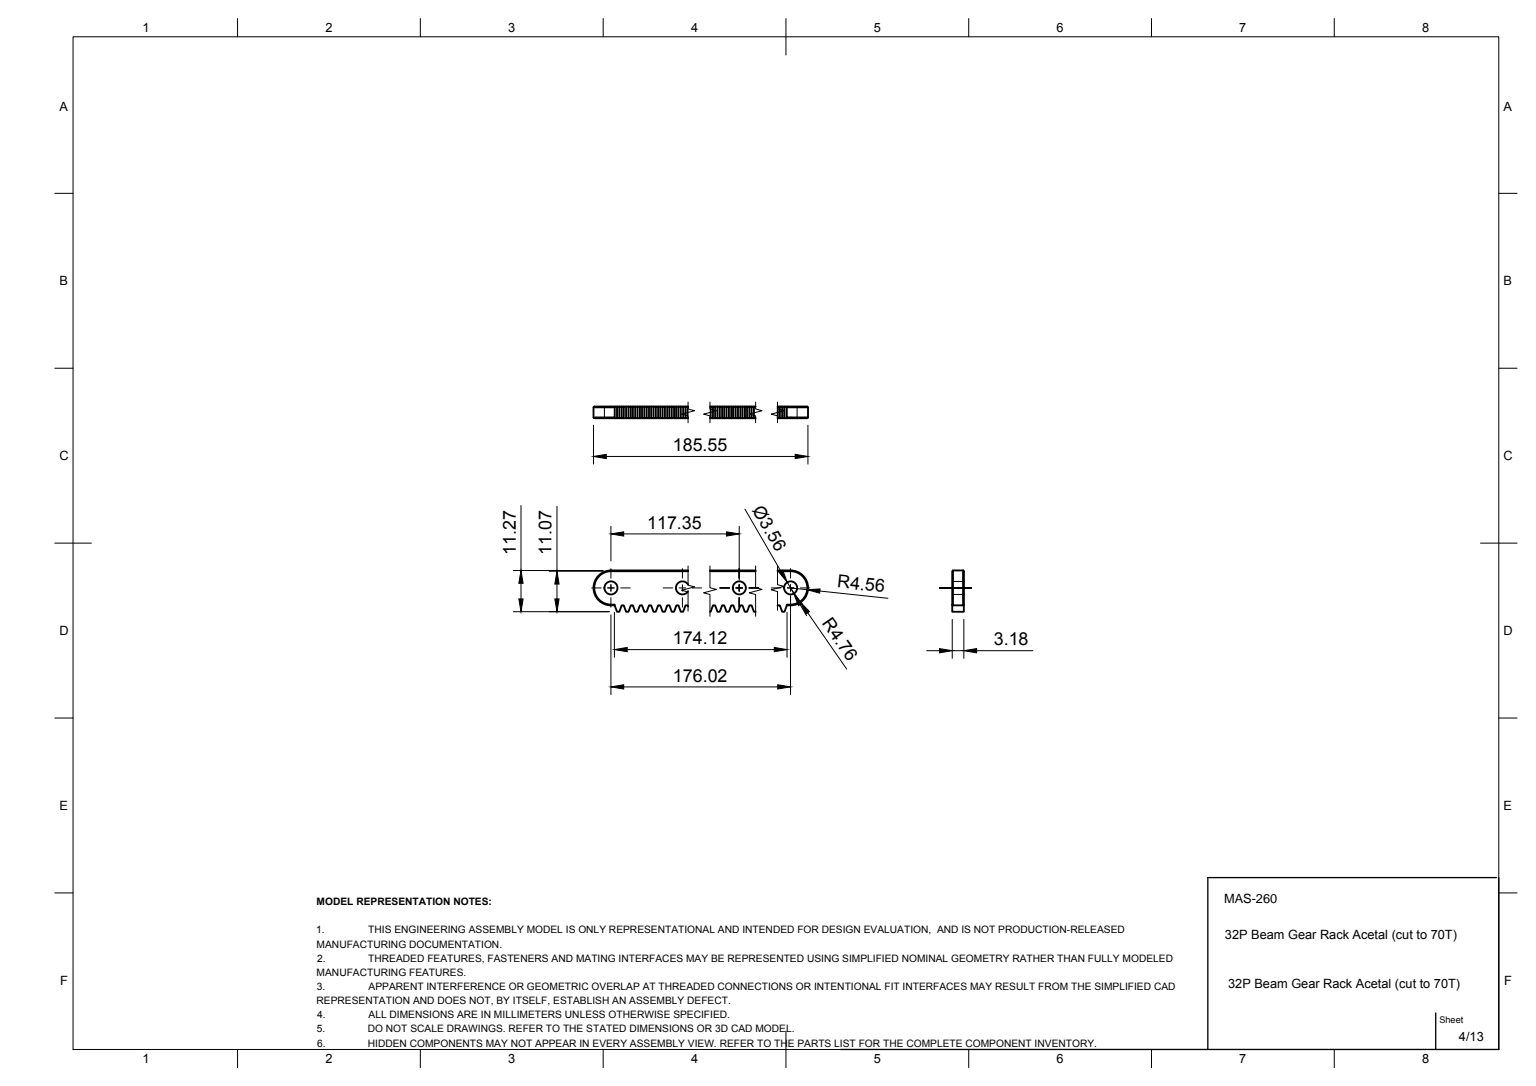
ISO-10303-21;
HEADER;
/* Generated by software containing ST-Developer
 * from STEP Tools, Inc. (www.steptools.com) 
 */

FILE_DESCRIPTION(
/* description */ (''),
/* implementation_level */ '2;1');

FILE_NAME(
/* name */ '32P Beam Gear Rack Acetal (cut to 70T).step',
/* time_stamp */ '2026-10-15T13:29:10-07:00',
/* author */ (''),
/* organization */ (''),
/* preprocessor_version */ 'ST-DEVELOPER v20.2',
/* originating_system */ 'Autodesk Translation Framework v15.15.0.0',
/* authorisation */ '');

FILE_SCHEMA (('AUTOMOTIVE_DESIGN { 1 0 10303 214 3 1 1 }'));
ENDSEC;

DATA;
#10=MECHANICAL_DESIGN_GEOMETRIC_PRESENTATION_REPRESENTATION('',(#939),#83219);
#911=SHAPE_REPRESENTATION_RELATIONSHIP('SRR','None',#83306,#925);
#925=ADVANCED_BREP_SHAPE_REPRESENTATION('',(#953),#83211);
#939=STYLED_ITEM('',(#83385),#953);
#953=MANIFOLD_SOLID_BREP('Body1',#26935);
#1061=FACE_BOUND('',#4681,.T.);
#1062=FACE_BOUND('',#4682,.T.);
#1063=FACE_BOUND('',#4683,.T.);
#1064=FACE_BOUND('',#4684,.T.);
#1065=FACE_BOUND('',#4685,.T.);
#1066=FACE_BOUND('',#4686,.T.);
#1067=FACE_BOUND('',#4687,.T.);
#1068=FACE_BOUND('',#4688,.T.);
#1069=FACE_BOUND('',#4689,.T.);
#1070=FACE_BOUND('',#4690,.T.);
#1071=FACE_BOUND('',#4692,.T.);
#1072=FACE_BOUND('',#4693,.T.);
#1073=FACE_BOUND('',#4694,.T.);
#1074=FACE_BOUND('',#4695,.T.);
#1075=FACE_BOUND('',#4696,.T.);
#1076=FACE_BOUND('',#4697,.T.);
#1077=FACE_BOUND('',#4698,.T.);
#1078=FACE_BOUND('',#4699,.T.);
#1079=FACE_BOUND('',#4700,.T.);
#1080=FACE_BOUND('',#4701,.T.);
#1423=PLANE('',#28001);
#1424=PLANE('',#28005);
#1425=PLANE('',#28009);
#1426=PLANE('',#28010);
#1427=PLANE('',#28013);
#1428=PLANE('',#28016);
#1429=PLANE('',#28017);
#1430=PLANE('',#28020);
#1431=PLANE('',#28023);
#1432=PLANE('',#28054);
#1433=PLANE('',#28055);
#1434=PLANE('',#28056);
#1435=PLANE('',#28057);
#1436=PLANE('',#28058);
#1437=PLANE('',#28059);
#1438=PLANE('',#28060);
#1439=PLANE('',#28061);
#1440=PLANE('',#28062);
#1441=PLANE('',#28063);
#1442=PLANE('',#28064);
#1443=PLANE('',#28065);
#1444=PLANE('',#28066);
#1445=PLANE('',#28067);
#1446=PLANE('',#28068);
#1447=PLANE('',#28069);
#1448=PLANE('',#28070);
#1449=PLANE('',#28071);
#1450=PLANE('',#28072);
#1451=PLANE('',#28073);
#1452=PLANE('',#28074);
#1453=PLANE('',#28075);
#1454=PLANE('',#28076);
#1455=PLANE('',#28077);
#1456=PLANE('',#28078);
#1457=PLANE('',#28079);
#1458=PLANE('',#28080);
#1459=PLANE('',#28081);
#1460=PLANE('',#28082);
#1461=PLANE('',#28083);
#1462=PLANE('',#28084);
#1463=PLANE('',#28085);
#1464=PLANE('',#28086);
#1465=PLANE('',#28087);
#1466=PLANE('',#28088);
#1467=PLANE('',#28089);
#1468=PLANE('',#28090);
#1469=PLANE('',#28091);
#1470=PLANE('',#28092);
#1471=PLANE('',#28093);
#1472=PLANE('',#28094);
#1473=PLANE('',#28095);
#1474=PLANE('',#28096);
#1475=PLANE('',#28097);
#1476=PLANE('',#28098);
#1477=PLANE('',#28099);
#1478=PLANE('',#28100);
#1479=PLANE('',#28101);
#1480=PLANE('',#28102);
#1481=PLANE('',#28103);
#1482=PLANE('',#28104);
#1483=PLANE('',#28105);
#1484=PLANE('',#28106);
#1485=PLANE('',#28107);
#1486=PLANE('',#28108);
#1487=PLANE('',#28109);
#1488=PLANE('',#28110);
#1489=PLANE('',#28111);
#1490=PLANE('',#28112);
#1491=PLANE('',#28113);
#1492=PLANE('',#28114);
#1493=PLANE('',#28115);
#1494=PLANE('',#28116);
#1495=PLANE('',#28117);
#1496=PLANE('',#28118);
#1497=PLANE('',#28119);
#1498=PLANE('',#28120);
#1499=PLANE('',#28121);
#1500=PLANE('',#28122);
#1501=PLANE('',#28123);
#1502=PLANE('',#28124);
#1503=PLANE('',#28125);
#1504=PLANE('',#28126);
#1505=PLANE('',#28127);
#1506=PLANE('',#28128);
#1507=PLANE('',#28129);
#1508=PLANE('',#28130);
#1509=PLANE('',#28131);
#1510=PLANE('',#28132);
#1511=PLANE('',#28133);
#1512=PLANE('',#28134);
#1513=PLANE('',#28135);
#1514=PLANE('',#28136);
#1515=PLANE('',#28137);
#1516=PLANE('',#28138);
#1517=PLANE('',#28139);
#1518=PLANE('',#28140);
#1519=PLANE('',#28141);
#1520=PLANE('',#28142);
#1521=PLANE('',#28143);
#1522=PLANE('',#28144);
#1523=PLANE('',#28145);
#1524=PLANE('',#28146);
#1525=PLANE('',#28147);
#1526=PLANE('',#28148);
#1527=PLANE('',#28149);
#1528=PLANE('',#28150);
#1529=PLANE('',#28151);
#1530=PLANE('',#28152);
#1531=PLANE('',#28153);
#1532=PLANE('',#28154);
#1533=PLANE('',#28155);
#1534=PLANE('',#28156);
#1535=PLANE('',#28157);
#1536=PLANE('',#28158);
#1537=PLANE('',#28159);
#1538=PLANE('',#28160);
#1539=PLANE('',#28161);
#1540=PLANE('',#28162);
#1541=PLANE('',#28163);
#1542=PLANE('',#28164);
#1543=PLANE('',#28165);
#1544=PLANE('',#28166);
#1545=PLANE('',#28167);
#1546=PLANE('',#28168);
#1547=PLANE('',#28169);
#1548=PLANE('',#28170);
#1549=PLANE('',#28171);
#1550=PLANE('',#28172);
#1551=PLANE('',#28173);
#1552=PLANE('',#28174);
#1553=PLANE('',#28175);
#1554=PLANE('',#28176);
#1555=PLANE('',#28177);
#1556=PLANE('',#28178);
#1557=PLANE('',#28179);
#1558=PLANE('',#28180);
#1559=PLANE('',#28181);
#1560=PLANE('',#28182);
#1561=PLANE('',#28183);
#1562=PLANE('',#28184);
#1563=PLANE('',#28185);
#1564=PLANE('',#28186);
#1565=PLANE('',#28187);
#1566=PLANE('',#28188);
#1567=PLANE('',#28189);
#1568=PLANE('',#28190);
#1569=PLANE('',#28191);
#1570=PLANE('',#28192);
#1571=PLANE('',#28193);
#1572=PLANE('',#28194);
#1573=PLANE('',#28195);
#1574=PLANE('',#28196);
#1575=PLANE('',#28197);
#1576=PLANE('',#28198);
#1577=PLANE('',#28199);
#1578=PLANE('',#28200);
#1579=PLANE('',#28201);
#1580=PLANE('',#28202);
#1581=PLANE('',#28203);
#1582=PLANE('',#28204);
#1583=PLANE('',#28205);
#1584=PLANE('',#28206);
#1585=PLANE('',#28207);
#1586=PLANE('',#28208);
#1587=PLANE('',#28209);
#1588=PLANE('',#28210);
#1589=PLANE('',#28211);
#1590=PLANE('',#28212);
#1591=PLANE('',#28213);
#1592=PLANE('',#28214);
#1593=PLANE('',#28215);
#1594=PLANE('',#28216);
#1595=PLANE('',#28217);
#1596=PLANE('',#28218);
#1597=PLANE('',#28219);
#1598=PLANE('',#28220);
#1599=PLANE('',#28221);
#1600=PLANE('',#28222);
#1601=PLANE('',#28223);
#1602=PLANE('',#28224);
#1603=PLANE('',#28225);
#1604=PLANE('',#28226);
#1605=PLANE('',#28227);
#1606=PLANE('',#28228);
#1607=PLANE('',#28229);
#1608=PLANE('',#28230);
#1609=PLANE('',#28231);
#1610=PLANE('',#28232);
#1611=PLANE('',#28233);
#1612=PLANE('',#28234);
#1613=PLANE('',#28235);
#1614=PLANE('',#28236);
#1615=PLANE('',#28237);
#1616=PLANE('',#28238);
#1617=PLANE('',#28239);
#1618=PLANE('',#28240);
#1619=PLANE('',#28241);
#1620=PLANE('',#28242);
#1621=PLANE('',#28243);
#1622=PLANE('',#28244);
#1623=PLANE('',#28245);
#1624=PLANE('',#28246);
#1625=PLANE('',#28247);
#1626=PLANE('',#28248);
#1627=PLANE('',#28249);
#1628=PLANE('',#28250);
#1629=PLANE('',#28251);
#1630=PLANE('',#28252);
#1631=PLANE('',#28253);
#1632=PLANE('',#28254);
#1633=PLANE('',#28255);
#1634=PLANE('',#28256);
#1635=PLANE('',#28257);
#1636=PLANE('',#28258);
#1637=PLANE('',#28259);
#1638=PLANE('',#28260);
#1639=PLANE('',#28261);
#1640=PLANE('',#28262);
#1641=PLANE('',#28263);
#1642=PLANE('',#28264);
#1643=PLANE('',#28265);
#1644=PLANE('',#28266);
#1645=PLANE('',#28267);
#1646=PLANE('',#28268);
#1647=PLANE('',#28269);
#1648=PLANE('',#28270);
#1649=PLANE('',#28271);
#1650=PLANE('',#28272);
#1651=PLANE('',#28273);
#1652=PLANE('',#28274);
#1653=PLANE('',#28275);
#1654=PLANE('',#28276);
#1655=PLANE('',#28277);
#1656=PLANE('',#28278);
#1657=PLANE('',#28279);
#1658=PLANE('',#28280);
#1659=PLANE('',#28281);
#1660=PLANE('',#28282);
#1661=PLANE('',#28283);
#1662=PLANE('',#28284);
#1663=PLANE('',#28285);
#1664=PLANE('',#28286);
#1665=PLANE('',#28287);
#1666=PLANE('',#28288);
#1667=PLANE('',#28289);
#1668=PLANE('',#28290);
#1669=PLANE('',#28291);
#1670=PLANE('',#28292);
#1671=PLANE('',#28293);
#1672=PLANE('',#28294);
#1673=PLANE('',#28295);
#1674=PLANE('',#28296);
#1675=PLANE('',#28297);
#1676=PLANE('',#28298);
#1677=PLANE('',#28299);
#1678=PLANE('',#28300);
#1679=PLANE('',#28301);
#1680=PLANE('',#28302);
#1681=PLANE('',#28303);
#1682=PLANE('',#28304);
#1683=PLANE('',#28305);
#1684=PLANE('',#28306);
#1685=PLANE('',#28307);
#1686=PLANE('',#28308);
#1687=PLANE('',#28309);
#1688=PLANE('',#28310);
#1689=PLANE('',#28311);
#1690=PLANE('',#28312);
#1691=PLANE('',#28313);
#1692=PLANE('',#28314);
#1693=PLANE('',#28315);
#1694=PLANE('',#28316);
#1695=PLANE('',#28317);
#1696=PLANE('',#28318);
#1697=PLANE('',#28319);
#1698=PLANE('',#28320);
#1699=PLANE('',#28321);
#1700=PLANE('',#28322);
#1701=PLANE('',#28323);
#1702=PLANE('',#28324);
#1703=PLANE('',#28325);
#1704=PLANE('',#28326);
#1705=PLANE('',#28327);
#1706=PLANE('',#28328);
#1707=PLANE('',#28329);
#1708=PLANE('',#28330);
#1709=PLANE('',#28331);
#1710=PLANE('',#28332);
#1711=PLANE('',#28333);
#1712=PLANE('',#28334);
#2282=CYLINDRICAL_SURFACE('',#28011,4.7625);
#2283=CYLINDRICAL_SURFACE('',#28014,4.7625);
#2284=CYLINDRICAL_SURFACE('',#28024,1.778);
#2285=CYLINDRICAL_SURFACE('',#28027,1.778);
#2286=CYLINDRICAL_SURFACE('',#28030,1.778);
#2287=CYLINDRICAL_SURFACE('',#28033,1.778);
#2288=CYLINDRICAL_SURFACE('',#28036,1.778);
#2289=CYLINDRICAL_SURFACE('',#28039,1.778);
#2290=CYLINDRICAL_SURFACE('',#28042,1.778);
#2291=CYLINDRICAL_SURFACE('',#28045,1.778);
#2292=CYLINDRICAL_SURFACE('',#28048,1.778);
#2293=CYLINDRICAL_SURFACE('',#28051,1.778);
#2897=FACE_OUTER_BOUND('',#4376,.T.);
#2898=FACE_OUTER_BOUND('',#4377,.T.);
#2899=FACE_OUTER_BOUND('',#4378,.T.);
#2900=FACE_OUTER_BOUND('',#4379,.T.);
#2901=FACE_OUTER_BOUND('',#4380,.T.);
#2902=FACE_OUTER_BOUND('',#4381,.T.);
#2903=FACE_OUTER_BOUND('',#4382,.T.);
#2904=FACE_OUTER_BOUND('',#4383,.T.);
#2905=FACE_OUTER_BOUND('',#4384,.T.);
#2906=FACE_OUTER_BOUND('',#4385,.T.);
#2907=FACE_OUTER_BOUND('',#4386,.T.);
#2908=FACE_OUTER_BOUND('',#4387,.T.);
#2909=FACE_OUTER_BOUND('',#4388,.T.);
#2910=FACE_OUTER_BOUND('',#4389,.T.);
#2911=FACE_OUTER_BOUND('',#4390,.T.);
#2912=FACE_OUTER_BOUND('',#4391,.T.);
#2913=FACE_OUTER_BOUND('',#4392,.T.);
#2914=FACE_OUTER_BOUND('',#4393,.T.);
#2915=FACE_OUTER_BOUND('',#4394,.T.);
#2916=FACE_OUTER_BOUND('',#4395,.T.);
#2917=FACE_OUTER_BOUND('',#4396,.T.);
#2918=FACE_OUTER_BOUND('',#4397,.T.);
#2919=FACE_OUTER_BOUND('',#4398,.T.);
#2920=FACE_OUTER_BOUND('',#4399,.T.);
#2921=FACE_OUTER_BOUND('',#4400,.T.);
#2922=FACE_OUTER_BOUND('',#4401,.T.);
#2923=FACE_OUTER_BOUND('',#4402,.T.);
#2924=FACE_OUTER_BOUND('',#4403,.T.);
#2925=FACE_OUTER_BOUND('',#4404,.T.);
#2926=FACE_OUTER_BOUND('',#4405,.T.);
#2927=FACE_OUTER_BOUND('',#4406,.T.);
#2928=FACE_OUTER_BOUND('',#4407,.T.);
#2929=FACE_OUTER_BOUND('',#4408,.T.);
#2930=FACE_OUTER_BOUND('',#4409,.T.);
#2931=FACE_OUTER_BOUND('',#4410,.T.);
#2932=FACE_OUTER_BOUND('',#4411,.T.);
#2933=FACE_OUTER_BOUND('',#4412,.T.);
#2934=FACE_OUTER_BOUND('',#4413,.T.);
#2935=FACE_OUTER_BOUND('',#4414,.T.);
#2936=FACE_OUTER_BOUND('',#4415,.T.);
#2937=FACE_OUTER_BOUND('',#4416,.T.);
#2938=FACE_OUTER_BOUND('',#4417,.T.);
#2939=FACE_OUTER_BOUND('',#4418,.T.);
#2940=FACE_OUTER_BOUND('',#4419,.T.);
#2941=FACE_OUTER_BOUND('',#4420,.T.);
#2942=FACE_OUTER_BOUND('',#4421,.T.);
#2943=FACE_OUTER_BOUND('',#4422,.T.);
#2944=FACE_OUTER_BOUND('',#4423,.T.);
#2945=FACE_OUTER_BOUND('',#4424,.T.);
#2946=FACE_OUTER_BOUND('',#4425,.T.);
#2947=FACE_OUTER_BOUND('',#4426,.T.);
#2948=FACE_OUTER_BOUND('',#4427,.T.);
#2949=FACE_OUTER_BOUND('',#4428,.T.);
#2950=FACE_OUTER_BOUND('',#4429,.T.);
#2951=FACE_OUTER_BOUND('',#4430,.T.);
#2952=FACE_OUTER_BOUND('',#4431,.T.);
#2953=FACE_OUTER_BOUND('',#4432,.T.);
#2954=FACE_OUTER_BOUND('',#4433,.T.);
#2955=FACE_OUTER_BOUND('',#4434,.T.);
#2956=FACE_OUTER_BOUND('',#4435,.T.);
#2957=FACE_OUTER_BOUND('',#4436,.T.);
#2958=FACE_OUTER_BOUND('',#4437,.T.);
#2959=FACE_OUTER_BOUND('',#4438,.T.);
#2960=FACE_OUTER_BOUND('',#4439,.T.);
#2961=FACE_OUTER_BOUND('',#4440,.T.);
#2962=FACE_OUTER_BOUND('',#4441,.T.);
#2963=FACE_OUTER_BOUND('',#4442,.T.);
#2964=FACE_OUTER_BOUND('',#4443,.T.);
#2965=FACE_OUTER_BOUND('',#4444,.T.);
#2966=FACE_OUTER_BOUND('',#4445,.T.);
#2967=FACE_OUTER_BOUND('',#4446,.T.);
#2968=FACE_OUTER_BOUND('',#4447,.T.);
#2969=FACE_OUTER_BOUND('',#4448,.T.);
#2970=FACE_OUTER_BOUND('',#4449,.T.);
#2971=FACE_OUTER_BOUND('',#4450,.T.);
#2972=FACE_OUTER_BOUND('',#4451,.T.);
#2973=FACE_OUTER_BOUND('',#4452,.T.);
#2974=FACE_OUTER_BOUND('',#4453,.T.);
#2975=FACE_OUTER_BOUND('',#4454,.T.);
#2976=FACE_OUTER_BOUND('',#4455,.T.);
#2977=FACE_OUTER_BOUND('',#4456,.T.);
#2978=FACE_OUTER_BOUND('',#4457,.T.);
#2979=FACE_OUTER_BOUND('',#4458,.T.);
#2980=FACE_OUTER_BOUND('',#4459,.T.);
#2981=FACE_OUTER_BOUND('',#4460,.T.);
#2982=FACE_OUTER_BOUND('',#4461,.T.);
#2983=FACE_OUTER_BOUND('',#4462,.T.);
#2984=FACE_OUTER_BOUND('',#4463,.T.);
#2985=FACE_OUTER_BOUND('',#4464,.T.);
#2986=FACE_OUTER_BOUND('',#4465,.T.);
#2987=FACE_OUTER_BOUND('',#4466,.T.);
#2988=FACE_OUTER_BOUND('',#4467,.T.);
#2989=FACE_OUTER_BOUND('',#4468,.T.);
#2990=FACE_OUTER_BOUND('',#4469,.T.);
#2991=FACE_OUTER_BOUND('',#4470,.T.);
#2992=FACE_OUTER_BOUND('',#4471,.T.);
#2993=FACE_OUTER_BOUND('',#4472,.T.);
#2994=FACE_OUTER_BOUND('',#4473,.T.);
#2995=FACE_OUTER_BOUND('',#4474,.T.);
#2996=FACE_OUTER_BOUND('',#4475,.T.);
#2997=FACE_OUTER_BOUND('',#4476,.T.);
#2998=FACE_OUTER_BOUND('',#4477,.T.);
#2999=FACE_OUTER_BOUND('',#4478,.T.);
#3000=FACE_OUTER_BOUND('',#4479,.T.);
#3001=FACE_OUTER_BOUND('',#4480,.T.);
#3002=FACE_OUTER_BOUND('',#4481,.T.);
#3003=FACE_OUTER_BOUND('',#4482,.T.);
#3004=FACE_OUTER_BOUND('',#4483,.T.);
#3005=FACE_OUTER_BOUND('',#4484,.T.);
#3006=FACE_OUTER_BOUND('',#4485,.T.);
#3007=FACE_OUTER_BOUND('',#4486,.T.);
#3008=FACE_OUTER_BOUND('',#4487,.T.);
#3009=FACE_OUTER_BOUND('',#4488,.T.);
#3010=FACE_OUTER_BOUND('',#4489,.T.);
#3011=FACE_OUTER_BOUND('',#4490,.T.);
#3012=FACE_OUTER_BOUND('',#4491,.T.);
#3013=FACE_OUTER_BOUND('',#4492,.T.);
#3014=FACE_OUTER_BOUND('',#4493,.T.);
#3015=FACE_OUTER_BOUND('',#4494,.T.);
#3016=FACE_OUTER_BOUND('',#4495,.T.);
#3017=FACE_OUTER_BOUND('',#4496,.T.);
#3018=FACE_OUTER_BOUND('',#4497,.T.);
#3019=FACE_OUTER_BOUND('',#4498,.T.);
#3020=FACE_OUTER_BOUND('',#4499,.T.);
#3021=FACE_OUTER_BOUND('',#4500,.T.);
#3022=FACE_OUTER_BOUND('',#4501,.T.);
#3023=FACE_OUTER_BOUND('',#4502,.T.);
#3024=FACE_OUTER_BOUND('',#4503,.T.);
#3025=FACE_OUTER_BOUND('',#4504,.T.);
#3026=FACE_OUTER_BOUND('',#4505,.T.);
#3027=FACE_OUTER_BOUND('',#4506,.T.);
#3028=FACE_OUTER_BOUND('',#4507,.T.);
#3029=FACE_OUTER_BOUND('',#4508,.T.);
#3030=FACE_OUTER_BOUND('',#4509,.T.);
#3031=FACE_OUTER_BOUND('',#4510,.T.);
#3032=FACE_OUTER_BOUND('',#4511,.T.);
#3033=FACE_OUTER_BOUND('',#4512,.T.);
#3034=FACE_OUTER_BOUND('',#4513,.T.);
#3035=FACE_OUTER_BOUND('',#4514,.T.);
#3036=FACE_OUTER_BOUND('',#4515,.T.);
#3037=FACE_OUTER_BOUND('',#4516,.T.);
#3038=FACE_OUTER_BOUND('',#4517,.T.);
#3039=FACE_OUTER_BOUND('',#4518,.T.);
#3040=FACE_OUTER_BOUND('',#4519,.T.);
#3041=FACE_OUTER_BOUND('',#4520,.T.);
#3042=FACE_OUTER_BOUND('',#4521,.T.);
#3043=FACE_OUTER_BOUND('',#4522,.T.);
#3044=FACE_OUTER_BOUND('',#4523,.T.);
#3045=FACE_OUTER_BOUND('',#4524,.T.);
#3046=FACE_OUTER_BOUND('',#4525,.T.);
#3047=FACE_OUTER_BOUND('',#4526,.T.);
#3048=FACE_OUTER_BOUND('',#4527,.T.);
#3049=FACE_OUTER_BOUND('',#4528,.T.);
#3050=FACE_OUTER_BOUND('',#4529,.T.);
#3051=FACE_OUTER_BOUND('',#4530,.T.);
#3052=FACE_OUTER_BOUND('',#4531,.T.);
#3053=FACE_OUTER_BOUND('',#4532,.T.);
#3054=FACE_OUTER_BOUND('',#4533,.T.);
#3055=FACE_OUTER_BOUND('',#4534,.T.);
#3056=FACE_OUTER_BOUND('',#4535,.T.);
#3057=FACE_OUTER_BOUND('',#4536,.T.);
#3058=FACE_OUTER_BOUND('',#4537,.T.);
#3059=FACE_OUTER_BOUND('',#4538,.T.);
#3060=FACE_OUTER_BOUND('',#4539,.T.);
#3061=FACE_OUTER_BOUND('',#4540,.T.);
#3062=FACE_OUTER_BOUND('',#4541,.T.);
#3063=FACE_OUTER_BOUND('',#4542,.T.);
#3064=FACE_OUTER_BOUND('',#4543,.T.);
#3065=FACE_OUTER_BOUND('',#4544,.T.);
#3066=FACE_OUTER_BOUND('',#4545,.T.);
#3067=FACE_OUTER_BOUND('',#4546,.T.);
#3068=FACE_OUTER_BOUND('',#4547,.T.);
#3069=FACE_OUTER_BOUND('',#4548,.T.);
#3070=FACE_OUTER_BOUND('',#4549,.T.);
#3071=FACE_OUTER_BOUND('',#4550,.T.);
#3072=FACE_OUTER_BOUND('',#4551,.T.);
#3073=FACE_OUTER_BOUND('',#4552,.T.);
#3074=FACE_OUTER_BOUND('',#4553,.T.);
#3075=FACE_OUTER_BOUND('',#4554,.T.);
#3076=FACE_OUTER_BOUND('',#4555,.T.);
#3077=FACE_OUTER_BOUND('',#4556,.T.);
#3078=FACE_OUTER_BOUND('',#4557,.T.);
#3079=FACE_OUTER_BOUND('',#4558,.T.);
#3080=FACE_OUTER_BOUND('',#4559,.T.);
#3081=FACE_OUTER_BOUND('',#4560,.T.);
#3082=FACE_OUTER_BOUND('',#4561,.T.);
#3083=FACE_OUTER_BOUND('',#4562,.T.);
#3084=FACE_OUTER_BOUND('',#4563,.T.);
#3085=FACE_OUTER_BOUND('',#4564,.T.);
#3086=FACE_OUTER_BOUND('',#4565,.T.);
#3087=FACE_OUTER_BOUND('',#4566,.T.);
#3088=FACE_OUTER_BOUND('',#4567,.T.);
#3089=FACE_OUTER_BOUND('',#4568,.T.);
#3090=FACE_OUTER_BOUND('',#4569,.T.);
#3091=FACE_OUTER_BOUND('',#4570,.T.);
#3092=FACE_OUTER_BOUND('',#4571,.T.);
#3093=FACE_OUTER_BOUND('',#4572,.T.);
#3094=FACE_OUTER_BOUND('',#4573,.T.);
#3095=FACE_OUTER_BOUND('',#4574,.T.);
#3096=FACE_OUTER_BOUND('',#4575,.T.);
#3097=FACE_OUTER_BOUND('',#4576,.T.);
#3098=FACE_OUTER_BOUND('',#4577,.T.);
#3099=FACE_OUTER_BOUND('',#4578,.T.);
#3100=FACE_OUTER_BOUND('',#4579,.T.);
#3101=FACE_OUTER_BOUND('',#4580,.T.);
#3102=FACE_OUTER_BOUND('',#4581,.T.);
#3103=FACE_OUTER_BOUND('',#4582,.T.);
#3104=FACE_OUTER_BOUND('',#4583,.T.);
#3105=FACE_OUTER_BOUND('',#4584,.T.);
#3106=FACE_OUTER_BOUND('',#4585,.T.);
#3107=FACE_OUTER_BOUND('',#4586,.T.);
#3108=FACE_OUTER_BOUND('',#4587,.T.);
#3109=FACE_OUTER_BOUND('',#4588,.T.);
#3110=FACE_OUTER_BOUND('',#4589,.T.);
#3111=FACE_OUTER_BOUND('',#4590,.T.);
#3112=FACE_OUTER_BOUND('',#4591,.T.);
#3113=FACE_OUTER_BOUND('',#4592,.T.);
#3114=FACE_OUTER_BOUND('',#4593,.T.);
#3115=FACE_OUTER_BOUND('',#4594,.T.);
#3116=FACE_OUTER_BOUND('',#4595,.T.);
#3117=FACE_OUTER_BOUND('',#4596,.T.);
#3118=FACE_OUTER_BOUND('',#4597,.T.);
#3119=FACE_OUTER_BOUND('',#4598,.T.);
#3120=FACE_OUTER_BOUND('',#4599,.T.);
#3121=FACE_OUTER_BOUND('',#4600,.T.);
#3122=FACE_OUTER_BOUND('',#4601,.T.);
#3123=FACE_OUTER_BOUND('',#4602,.T.);
#3124=FACE_OUTER_BOUND('',#4603,.T.);
#3125=FACE_OUTER_BOUND('',#4604,.T.);
#3126=FACE_OUTER_BOUND('',#4605,.T.);
#3127=FACE_OUTER_BOUND('',#4606,.T.);
#3128=FACE_OUTER_BOUND('',#4607,.T.);
#3129=FACE_OUTER_BOUND('',#4608,.T.);
#3130=FACE_OUTER_BOUND('',#4609,.T.);
#3131=FACE_OUTER_BOUND('',#4610,.T.);
#3132=FACE_OUTER_BOUND('',#4611,.T.);
#3133=FACE_OUTER_BOUND('',#4612,.T.);
#3134=FACE_OUTER_BOUND('',#4613,.T.);
#3135=FACE_OUTER_BOUND('',#4614,.T.);
#3136=FACE_OUTER_BOUND('',#4615,.T.);
#3137=FACE_OUTER_BOUND('',#4616,.T.);
#3138=FACE_OUTER_BOUND('',#4617,.T.);
#3139=FACE_OUTER_BOUND('',#4618,.T.);
#3140=FACE_OUTER_BOUND('',#4619,.T.);
#3141=FACE_OUTER_BOUND('',#4620,.T.);
#3142=FACE_OUTER_BOUND('',#4621,.T.);
#3143=FACE_OUTER_BOUND('',#4622,.T.);
#3144=FACE_OUTER_BOUND('',#4623,.T.);
#3145=FACE_OUTER_BOUND('',#4624,.T.);
#3146=FACE_OUTER_BOUND('',#4625,.T.);
#3147=FACE_OUTER_BOUND('',#4626,.T.);
#3148=FACE_OUTER_BOUND('',#4627,.T.);
#3149=FACE_OUTER_BOUND('',#4628,.T.);
#3150=FACE_OUTER_BOUND('',#4629,.T.);
#3151=FACE_OUTER_BOUND('',#4630,.T.);
#3152=FACE_OUTER_BOUND('',#4631,.T.);
#3153=FACE_OUTER_BOUND('',#4632,.T.);
#3154=FACE_OUTER_BOUND('',#4633,.T.);
#3155=FACE_OUTER_BOUND('',#4634,.T.);
#3156=FACE_OUTER_BOUND('',#4635,.T.);
#3157=FACE_OUTER_BOUND('',#4636,.T.);
#3158=FACE_OUTER_BOUND('',#4637,.T.);
#3159=FACE_OUTER_BOUND('',#4638,.T.);
#3160=FACE_OUTER_BOUND('',#4639,.T.);
#3161=FACE_OUTER_BOUND('',#4640,.T.);
#3162=FACE_OUTER_BOUND('',#4641,.T.);
#3163=FACE_OUTER_BOUND('',#4642,.T.);
#3164=FACE_OUTER_BOUND('',#4643,.T.);
#3165=FACE_OUTER_BOUND('',#4644,.T.);
#3166=FACE_OUTER_BOUND('',#4645,.T.);
#3167=FACE_OUTER_BOUND('',#4646,.T.);
#3168=FACE_OUTER_BOUND('',#4647,.T.);
#3169=FACE_OUTER_BOUND('',#4648,.T.);
#3170=FACE_OUTER_BOUND('',#4649,.T.);
#3171=FACE_OUTER_BOUND('',#4650,.T.);
#3172=FACE_OUTER_BOUND('',#4651,.T.);
#3173=FACE_OUTER_BOUND('',#4652,.T.);
#3174=FACE_OUTER_BOUND('',#4653,.T.);
#3175=FACE_OUTER_BOUND('',#4654,.T.);
#3176=FACE_OUTER_BOUND('',#4655,.T.);
#3177=FACE_OUTER_BOUND('',#4656,.T.);
#3178=FACE_OUTER_BOUND('',#4657,.T.);
#3179=FACE_OUTER_BOUND('',#4658,.T.);
#3180=FACE_OUTER_BOUND('',#4659,.T.);
#3181=FACE_OUTER_BOUND('',#4660,.T.);
#3182=FACE_OUTER_BOUND('',#4661,.T.);
#3183=FACE_OUTER_BOUND('',#4662,.T.);
#3184=FACE_OUTER_BOUND('',#4663,.T.);
#3185=FACE_OUTER_BOUND('',#4664,.T.);
#3186=FACE_OUTER_BOUND('',#4665,.T.);
#3187=FACE_OUTER_BOUND('',#4666,.T.);
#3188=FACE_OUTER_BOUND('',#4667,.T.);
#3189=FACE_OUTER_BOUND('',#4668,.T.);
#3190=FACE_OUTER_BOUND('',#4669,.T.);
#3191=FACE_OUTER_BOUND('',#4670,.T.);
#3192=FACE_OUTER_BOUND('',#4671,.T.);
#3193=FACE_OUTER_BOUND('',#4672,.T.);
#3194=FACE_OUTER_BOUND('',#4673,.T.);
#3195=FACE_OUTER_BOUND('',#4674,.T.);
#3196=FACE_OUTER_BOUND('',#4675,.T.);
#3197=FACE_OUTER_BOUND('',#4676,.T.);
#3198=FACE_OUTER_BOUND('',#4677,.T.);
#3199=FACE_OUTER_BOUND('',#4678,.T.);
#3200=FACE_OUTER_BOUND('',#4679,.T.);
#3201=FACE_OUTER_BOUND('',#4680,.T.);
#3202=FACE_OUTER_BOUND('',#4691,.T.);
#4376=EDGE_LOOP('',(#20474,#20475,#20476,#20477));
#4377=EDGE_LOOP('',(#20478,#20479,#20480,#20481));
#4378=EDGE_LOOP('',(#20482,#20483,#20484,#20485));
#4379=EDGE_LOOP('',(#20486,#20487,#20488,#20489));
#4380=EDGE_LOOP('',(#20490,#20491,#20492,#20493));
#4381=EDGE_LOOP('',(#20494,#20495,#20496,#20497));
#4382=EDGE_LOOP('',(#20498,#20499,#20500,#20501));
#4383=EDGE_LOOP('',(#20502,#20503,#20504,#20505));
#4384=EDGE_LOOP('',(#20506,#20507,#20508,#20509));
#4385=EDGE_LOOP('',(#20510,#20511,#20512,#20513));
#4386=EDGE_LOOP('',(#20514,#20515,#20516,#20517));
#4387=EDGE_LOOP('',(#20518,#20519,#20520,#20521));
#4388=EDGE_LOOP('',(#20522,#20523,#20524,#20525));
#4389=EDGE_LOOP('',(#20526,#20527,#20528,#20529));
#4390=EDGE_LOOP('',(#20530,#20531,#20532,#20533));
#4391=EDGE_LOOP('',(#20534,#20535,#20536,#20537));
#4392=EDGE_LOOP('',(#20538,#20539,#20540,#20541));
#4393=EDGE_LOOP('',(#20542,#20543,#20544,#20545));
#4394=EDGE_LOOP('',(#20546,#20547,#20548,#20549));
#4395=EDGE_LOOP('',(#20550,#20551,#20552,#20553));
#4396=EDGE_LOOP('',(#20554,#20555,#20556,#20557));
#4397=EDGE_LOOP('',(#20558,#20559,#20560,#20561));
#4398=EDGE_LOOP('',(#20562,#20563,#20564,#20565));
#4399=EDGE_LOOP('',(#20566,#20567,#20568,#20569));
#4400=EDGE_LOOP('',(#20570,#20571,#20572,#20573));
#4401=EDGE_LOOP('',(#20574,#20575,#20576,#20577,#20578,#20579));
#4402=EDGE_LOOP('',(#20580,#20581,#20582,#20583));
#4403=EDGE_LOOP('',(#20584,#20585,#20586,#20587));
#4404=EDGE_LOOP('',(#20588,#20589,#20590,#20591));
#4405=EDGE_LOOP('',(#20592,#20593,#20594,#20595));
#4406=EDGE_LOOP('',(#20596,#20597,#20598,#20599));
#4407=EDGE_LOOP('',(#20600,#20601,#20602,#20603));
#4408=EDGE_LOOP('',(#20604,#20605,#20606,#20607));
#4409=EDGE_LOOP('',(#20608,#20609,#20610,#20611));
#4410=EDGE_LOOP('',(#20612,#20613,#20614,#20615));
#4411=EDGE_LOOP('',(#20616,#20617,#20618,#20619));
#4412=EDGE_LOOP('',(#20620,#20621,#20622,#20623));
#4413=EDGE_LOOP('',(#20624,#20625,#20626,#20627));
#4414=EDGE_LOOP('',(#20628,#20629,#20630,#20631));
#4415=EDGE_LOOP('',(#20632,#20633,#20634,#20635));
#4416=EDGE_LOOP('',(#20636,#20637,#20638,#20639));
#4417=EDGE_LOOP('',(#20640,#20641,#20642,#20643));
#4418=EDGE_LOOP('',(#20644,#20645,#20646,#20647));
#4419=EDGE_LOOP('',(#20648,#20649,#20650,#20651));
#4420=EDGE_LOOP('',(#20652,#20653,#20654,#20655));
#4421=EDGE_LOOP('',(#20656,#20657,#20658,#20659));
#4422=EDGE_LOOP('',(#20660,#20661,#20662,#20663));
#4423=EDGE_LOOP('',(#20664,#20665,#20666,#20667));
#4424=EDGE_LOOP('',(#20668,#20669,#20670,#20671));
#4425=EDGE_LOOP('',(#20672,#20673,#20674,#20675));
#4426=EDGE_LOOP('',(#20676,#20677,#20678,#20679));
#4427=EDGE_LOOP('',(#20680,#20681,#20682,#20683));
#4428=EDGE_LOOP('',(#20684,#20685,#20686,#20687));
#4429=EDGE_LOOP('',(#20688,#20689,#20690,#20691));
#4430=EDGE_LOOP('',(#20692,#20693,#20694,#20695));
#4431=EDGE_LOOP('',(#20696,#20697,#20698,#20699));
#4432=EDGE_LOOP('',(#20700,#20701,#20702,#20703));
#4433=EDGE_LOOP('',(#20704,#20705,#20706,#20707));
#4434=EDGE_LOOP('',(#20708,#20709,#20710,#20711));
#4435=EDGE_LOOP('',(#20712,#20713,#20714,#20715));
#4436=EDGE_LOOP('',(#20716,#20717,#20718,#20719));
#4437=EDGE_LOOP('',(#20720,#20721,#20722,#20723));
#4438=EDGE_LOOP('',(#20724,#20725,#20726,#20727));
#4439=EDGE_LOOP('',(#20728,#20729,#20730,#20731));
#4440=EDGE_LOOP('',(#20732,#20733,#20734,#20735));
#4441=EDGE_LOOP('',(#20736,#20737,#20738,#20739));
#4442=EDGE_LOOP('',(#20740,#20741,#20742,#20743));
#4443=EDGE_LOOP('',(#20744,#20745,#20746,#20747));
#4444=EDGE_LOOP('',(#20748,#20749,#20750,#20751));
#4445=EDGE_LOOP('',(#20752,#20753,#20754,#20755));
#4446=EDGE_LOOP('',(#20756,#20757,#20758,#20759));
#4447=EDGE_LOOP('',(#20760,#20761,#20762,#20763));
#4448=EDGE_LOOP('',(#20764,#20765,#20766,#20767));
#4449=EDGE_LOOP('',(#20768,#20769,#20770,#20771));
#4450=EDGE_LOOP('',(#20772,#20773,#20774,#20775));
#4451=EDGE_LOOP('',(#20776,#20777,#20778,#20779));
#4452=EDGE_LOOP('',(#20780,#20781,#20782,#20783));
#4453=EDGE_LOOP('',(#20784,#20785,#20786,#20787));
#4454=EDGE_LOOP('',(#20788,#20789,#20790,#20791));
#4455=EDGE_LOOP('',(#20792,#20793,#20794,#20795));
#4456=EDGE_LOOP('',(#20796,#20797,#20798,#20799));
#4457=EDGE_LOOP('',(#20800,#20801,#20802,#20803));
#4458=EDGE_LOOP('',(#20804,#20805,#20806,#20807));
#4459=EDGE_LOOP('',(#20808,#20809,#20810,#20811));
#4460=EDGE_LOOP('',(#20812,#20813,#20814,#20815));
#4461=EDGE_LOOP('',(#20816,#20817,#20818,#20819));
#4462=EDGE_LOOP('',(#20820,#20821,#20822,#20823));
#4463=EDGE_LOOP('',(#20824,#20825,#20826,#20827));
#4464=EDGE_LOOP('',(#20828,#20829,#20830,#20831));
#4465=EDGE_LOOP('',(#20832,#20833,#20834,#20835));
#4466=EDGE_LOOP('',(#20836,#20837,#20838,#20839));
#4467=EDGE_LOOP('',(#20840,#20841,#20842,#20843));
#4468=EDGE_LOOP('',(#20844,#20845,#20846,#20847));
#4469=EDGE_LOOP('',(#20848,#20849,#20850,#20851));
#4470=EDGE_LOOP('',(#20852,#20853,#20854,#20855));
#4471=EDGE_LOOP('',(#20856,#20857,#20858,#20859));
#4472=EDGE_LOOP('',(#20860,#20861,#20862,#20863));
#4473=EDGE_LOOP('',(#20864,#20865,#20866,#20867));
#4474=EDGE_LOOP('',(#20868,#20869,#20870,#20871));
#4475=EDGE_LOOP('',(#20872,#20873,#20874,#20875));
#4476=EDGE_LOOP('',(#20876,#20877,#20878,#20879));
#4477=EDGE_LOOP('',(#20880,#20881,#20882,#20883));
#4478=EDGE_LOOP('',(#20884,#20885,#20886,#20887));
#4479=EDGE_LOOP('',(#20888,#20889,#20890,#20891));
#4480=EDGE_LOOP('',(#20892,#20893,#20894,#20895));
#4481=EDGE_LOOP('',(#20896,#20897,#20898,#20899));
#4482=EDGE_LOOP('',(#20900,#20901,#20902,#20903));
#4483=EDGE_LOOP('',(#20904,#20905,#20906,#20907));
#4484=EDGE_LOOP('',(#20908,#20909,#20910,#20911));
#4485=EDGE_LOOP('',(#20912,#20913,#20914,#20915));
#4486=EDGE_LOOP('',(#20916,#20917,#20918,#20919));
#4487=EDGE_LOOP('',(#20920,#20921,#20922,#20923));
#4488=EDGE_LOOP('',(#20924,#20925,#20926,#20927));
#4489=EDGE_LOOP('',(#20928,#20929,#20930,#20931));
#4490=EDGE_LOOP('',(#20932,#20933,#20934,#20935));
#4491=EDGE_LOOP('',(#20936,#20937,#20938,#20939));
#4492=EDGE_LOOP('',(#20940,#20941,#20942,#20943));
#4493=EDGE_LOOP('',(#20944,#20945,#20946,#20947));
#4494=EDGE_LOOP('',(#20948,#20949,#20950,#20951));
#4495=EDGE_LOOP('',(#20952,#20953,#20954,#20955));
#4496=EDGE_LOOP('',(#20956,#20957,#20958,#20959));
#4497=EDGE_LOOP('',(#20960,#20961,#20962,#20963));
#4498=EDGE_LOOP('',(#20964,#20965,#20966,#20967));
#4499=EDGE_LOOP('',(#20968,#20969,#20970,#20971));
#4500=EDGE_LOOP('',(#20972,#20973,#20974,#20975));
#4501=EDGE_LOOP('',(#20976,#20977,#20978,#20979));
#4502=EDGE_LOOP('',(#20980,#20981,#20982,#20983));
#4503=EDGE_LOOP('',(#20984,#20985,#20986,#20987));
#4504=EDGE_LOOP('',(#20988,#20989,#20990,#20991));
#4505=EDGE_LOOP('',(#20992,#20993,#20994,#20995));
#4506=EDGE_LOOP('',(#20996,#20997,#20998,#20999));
#4507=EDGE_LOOP('',(#21000,#21001,#21002,#21003));
#4508=EDGE_LOOP('',(#21004,#21005,#21006,#21007));
#4509=EDGE_LOOP('',(#21008,#21009,#21010,#21011));
#4510=EDGE_LOOP('',(#21012,#21013,#21014,#21015));
#4511=EDGE_LOOP('',(#21016,#21017,#21018,#21019));
#4512=EDGE_LOOP('',(#21020,#21021,#21022,#21023));
#4513=EDGE_LOOP('',(#21024,#21025,#21026,#21027));
#4514=EDGE_LOOP('',(#21028,#21029,#21030,#21031));
#4515=EDGE_LOOP('',(#21032,#21033,#21034,#21035));
#4516=EDGE_LOOP('',(#21036,#21037,#21038,#21039));
#4517=EDGE_LOOP('',(#21040,#21041,#21042,#21043));
#4518=EDGE_LOOP('',(#21044,#21045,#21046,#21047));
#4519=EDGE_LOOP('',(#21048,#21049,#21050,#21051));
#4520=EDGE_LOOP('',(#21052,#21053,#21054,#21055));
#4521=EDGE_LOOP('',(#21056,#21057,#21058,#21059));
#4522=EDGE_LOOP('',(#21060,#21061,#21062,#21063));
#4523=EDGE_LOOP('',(#21064,#21065,#21066,#21067));
#4524=EDGE_LOOP('',(#21068,#21069,#21070,#21071));
#4525=EDGE_LOOP('',(#21072,#21073,#21074,#21075));
#4526=EDGE_LOOP('',(#21076,#21077,#21078,#21079));
#4527=EDGE_LOOP('',(#21080,#21081,#21082,#21083));
#4528=EDGE_LOOP('',(#21084,#21085,#21086,#21087));
#4529=EDGE_LOOP('',(#21088,#21089,#21090,#21091));
#4530=EDGE_LOOP('',(#21092,#21093,#21094,#21095));
#4531=EDGE_LOOP('',(#21096,#21097,#21098,#21099));
#4532=EDGE_LOOP('',(#21100,#21101,#21102,#21103));
#4533=EDGE_LOOP('',(#21104,#21105,#21106,#21107));
#4534=EDGE_LOOP('',(#21108,#21109,#21110,#21111));
#4535=EDGE_LOOP('',(#21112,#21113,#21114,#21115));
#4536=EDGE_LOOP('',(#21116,#21117,#21118,#21119));
#4537=EDGE_LOOP('',(#21120,#21121,#21122,#21123));
#4538=EDGE_LOOP('',(#21124,#21125,#21126,#21127));
#4539=EDGE_LOOP('',(#21128,#21129,#21130,#21131));
#4540=EDGE_LOOP('',(#21132,#21133,#21134,#21135));
#4541=EDGE_LOOP('',(#21136,#21137,#21138,#21139));
#4542=EDGE_LOOP('',(#21140,#21141,#21142,#21143));
#4543=EDGE_LOOP('',(#21144,#21145,#21146,#21147));
#4544=EDGE_LOOP('',(#21148,#21149,#21150,#21151));
#4545=EDGE_LOOP('',(#21152,#21153,#21154,#21155));
#4546=EDGE_LOOP('',(#21156,#21157,#21158,#21159));
#4547=EDGE_LOOP('',(#21160,#21161,#21162,#21163));
#4548=EDGE_LOOP('',(#21164,#21165,#21166,#21167));
#4549=EDGE_LOOP('',(#21168,#21169,#21170,#21171));
#4550=EDGE_LOOP('',(#21172,#21173,#21174,#21175));
#4551=EDGE_LOOP('',(#21176,#21177,#21178,#21179));
#4552=EDGE_LOOP('',(#21180,#21181,#21182,#21183));
#4553=EDGE_LOOP('',(#21184,#21185,#21186,#21187));
#4554=EDGE_LOOP('',(#21188,#21189,#21190,#21191));
#4555=EDGE_LOOP('',(#21192,#21193,#21194,#21195));
#4556=EDGE_LOOP('',(#21196,#21197,#21198,#21199));
#4557=EDGE_LOOP('',(#21200,#21201,#21202,#21203));
#4558=EDGE_LOOP('',(#21204,#21205,#21206,#21207));
#4559=EDGE_LOOP('',(#21208,#21209,#21210,#21211));
#4560=EDGE_LOOP('',(#21212,#21213,#21214,#21215));
#4561=EDGE_LOOP('',(#21216,#21217,#21218,#21219));
#4562=EDGE_LOOP('',(#21220,#21221,#21222,#21223));
#4563=EDGE_LOOP('',(#21224,#21225,#21226,#21227));
#4564=EDGE_LOOP('',(#21228,#21229,#21230,#21231));
#4565=EDGE_LOOP('',(#21232,#21233,#21234,#21235));
#4566=EDGE_LOOP('',(#21236,#21237,#21238,#21239));
#4567=EDGE_LOOP('',(#21240,#21241,#21242,#21243));
#4568=EDGE_LOOP('',(#21244,#21245,#21246,#21247));
#4569=EDGE_LOOP('',(#21248,#21249,#21250,#21251));
#4570=EDGE_LOOP('',(#21252,#21253,#21254,#21255));
#4571=EDGE_LOOP('',(#21256,#21257,#21258,#21259));
#4572=EDGE_LOOP('',(#21260,#21261,#21262,#21263));
#4573=EDGE_LOOP('',(#21264,#21265,#21266,#21267));
#4574=EDGE_LOOP('',(#21268,#21269,#21270,#21271));
#4575=EDGE_LOOP('',(#21272,#21273,#21274,#21275));
#4576=EDGE_LOOP('',(#21276,#21277,#21278,#21279));
#4577=EDGE_LOOP('',(#21280,#21281,#21282,#21283));
#4578=EDGE_LOOP('',(#21284,#21285,#21286,#21287));
#4579=EDGE_LOOP('',(#21288,#21289,#21290,#21291));
#4580=EDGE_LOOP('',(#21292,#21293,#21294,#21295));
#4581=EDGE_LOOP('',(#21296,#21297,#21298,#21299));
#4582=EDGE_LOOP('',(#21300,#21301,#21302,#21303));
#4583=EDGE_LOOP('',(#21304,#21305,#21306,#21307));
#4584=EDGE_LOOP('',(#21308,#21309,#21310,#21311));
#4585=EDGE_LOOP('',(#21312,#21313,#21314,#21315));
#4586=EDGE_LOOP('',(#21316,#21317,#21318,#21319));
#4587=EDGE_LOOP('',(#21320,#21321,#21322,#21323));
#4588=EDGE_LOOP('',(#21324,#21325,#21326,#21327));
#4589=EDGE_LOOP('',(#21328,#21329,#21330,#21331));
#4590=EDGE_LOOP('',(#21332,#21333,#21334,#21335));
#4591=EDGE_LOOP('',(#21336,#21337,#21338,#21339));
#4592=EDGE_LOOP('',(#21340,#21341,#21342,#21343));
#4593=EDGE_LOOP('',(#21344,#21345,#21346,#21347));
#4594=EDGE_LOOP('',(#21348,#21349,#21350,#21351));
#4595=EDGE_LOOP('',(#21352,#21353,#21354,#21355));
#4596=EDGE_LOOP('',(#21356,#21357,#21358,#21359));
#4597=EDGE_LOOP('',(#21360,#21361,#21362,#21363));
#4598=EDGE_LOOP('',(#21364,#21365,#21366,#21367));
#4599=EDGE_LOOP('',(#21368,#21369,#21370,#21371));
#4600=EDGE_LOOP('',(#21372,#21373,#21374,#21375));
#4601=EDGE_LOOP('',(#21376,#21377,#21378,#21379));
#4602=EDGE_LOOP('',(#21380,#21381,#21382,#21383));
#4603=EDGE_LOOP('',(#21384,#21385,#21386,#21387));
#4604=EDGE_LOOP('',(#21388,#21389,#21390,#21391));
#4605=EDGE_LOOP('',(#21392,#21393,#21394,#21395));
#4606=EDGE_LOOP('',(#21396,#21397,#21398,#21399));
#4607=EDGE_LOOP('',(#21400,#21401,#21402,#21403));
#4608=EDGE_LOOP('',(#21404,#21405,#21406,#21407));
#4609=EDGE_LOOP('',(#21408,#21409,#21410,#21411));
#4610=EDGE_LOOP('',(#21412,#21413,#21414,#21415));
#4611=EDGE_LOOP('',(#21416,#21417,#21418,#21419));
#4612=EDGE_LOOP('',(#21420,#21421,#21422,#21423));
#4613=EDGE_LOOP('',(#21424,#21425,#21426,#21427));
#4614=EDGE_LOOP('',(#21428,#21429,#21430,#21431));
#4615=EDGE_LOOP('',(#21432,#21433,#21434,#21435));
#4616=EDGE_LOOP('',(#21436,#21437,#21438,#21439));
#4617=EDGE_LOOP('',(#21440,#21441,#21442,#21443));
#4618=EDGE_LOOP('',(#21444,#21445,#21446,#21447));
#4619=EDGE_LOOP('',(#21448,#21449,#21450,#21451));
#4620=EDGE_LOOP('',(#21452,#21453,#21454,#21455));
#4621=EDGE_LOOP('',(#21456,#21457,#21458,#21459));
#4622=EDGE_LOOP('',(#21460,#21461,#21462,#21463));
#4623=EDGE_LOOP('',(#21464,#21465,#21466,#21467));
#4624=EDGE_LOOP('',(#21468,#21469,#21470,#21471));
#4625=EDGE_LOOP('',(#21472,#21473,#21474,#21475));
#4626=EDGE_LOOP('',(#21476,#21477,#21478,#21479));
#4627=EDGE_LOOP('',(#21480,#21481,#21482,#21483));
#4628=EDGE_LOOP('',(#21484,#21485,#21486,#21487));
#4629=EDGE_LOOP('',(#21488,#21489,#21490,#21491));
#4630=EDGE_LOOP('',(#21492,#21493,#21494,#21495));
#4631=EDGE_LOOP('',(#21496,#21497,#21498,#21499));
#4632=EDGE_LOOP('',(#21500,#21501,#21502,#21503));
#4633=EDGE_LOOP('',(#21504,#21505,#21506,#21507));
#4634=EDGE_LOOP('',(#21508,#21509,#21510,#21511));
#4635=EDGE_LOOP('',(#21512,#21513,#21514,#21515));
#4636=EDGE_LOOP('',(#21516,#21517,#21518,#21519));
#4637=EDGE_LOOP('',(#21520,#21521,#21522,#21523));
#4638=EDGE_LOOP('',(#21524,#21525,#21526,#21527));
#4639=EDGE_LOOP('',(#21528,#21529,#21530,#21531));
#4640=EDGE_LOOP('',(#21532,#21533,#21534,#21535));
#4641=EDGE_LOOP('',(#21536,#21537,#21538,#21539));
#4642=EDGE_LOOP('',(#21540,#21541,#21542,#21543));
#4643=EDGE_LOOP('',(#21544,#21545,#21546,#21547));
#4644=EDGE_LOOP('',(#21548,#21549,#21550,#21551));
#4645=EDGE_LOOP('',(#21552,#21553,#21554,#21555));
#4646=EDGE_LOOP('',(#21556,#21557,#21558,#21559));
#4647=EDGE_LOOP('',(#21560,#21561,#21562,#21563));
#4648=EDGE_LOOP('',(#21564,#21565,#21566,#21567));
#4649=EDGE_LOOP('',(#21568,#21569,#21570,#21571));
#4650=EDGE_LOOP('',(#21572,#21573,#21574,#21575));
#4651=EDGE_LOOP('',(#21576,#21577,#21578,#21579));
#4652=EDGE_LOOP('',(#21580,#21581,#21582,#21583));
#4653=EDGE_LOOP('',(#21584,#21585,#21586,#21587));
#4654=EDGE_LOOP('',(#21588,#21589,#21590,#21591));
#4655=EDGE_LOOP('',(#21592,#21593,#21594,#21595));
#4656=EDGE_LOOP('',(#21596,#21597,#21598,#21599));
#4657=EDGE_LOOP('',(#21600,#21601,#21602,#21603));
#4658=EDGE_LOOP('',(#21604,#21605,#21606,#21607));
#4659=EDGE_LOOP('',(#21608,#21609,#21610,#21611));
#4660=EDGE_LOOP('',(#21612,#21613,#21614,#21615));
#4661=EDGE_LOOP('',(#21616,#21617,#21618,#21619));
#4662=EDGE_LOOP('',(#21620,#21621,#21622,#21623));
#4663=EDGE_LOOP('',(#21624,#21625,#21626,#21627));
#4664=EDGE_LOOP('',(#21628,#21629,#21630,#21631));
#4665=EDGE_LOOP('',(#21632,#21633,#21634,#21635));
#4666=EDGE_LOOP('',(#21636,#21637,#21638,#21639));
#4667=EDGE_LOOP('',(#21640,#21641,#21642,#21643));
#4668=EDGE_LOOP('',(#21644,#21645,#21646,#21647));
#4669=EDGE_LOOP('',(#21648,#21649,#21650,#21651));
#4670=EDGE_LOOP('',(#21652,#21653,#21654,#21655));
#4671=EDGE_LOOP('',(#21656,#21657,#21658,#21659));
#4672=EDGE_LOOP('',(#21660,#21661,#21662,#21663));
#4673=EDGE_LOOP('',(#21664,#21665,#21666,#21667));
#4674=EDGE_LOOP('',(#21668,#21669,#21670,#21671));
#4675=EDGE_LOOP('',(#21672,#21673,#21674,#21675));
#4676=EDGE_LOOP('',(#21676,#21677,#21678,#21679));
#4677=EDGE_LOOP('',(#21680,#21681,#21682,#21683));
#4678=EDGE_LOOP('',(#21684,#21685,#21686,#21687));
#4679=EDGE_LOOP('',(#21688,#21689,#21690,#21691,#21692,#21693));
#4680=EDGE_LOOP('',(#21694,#21695,#21696,#21697,#21698,#21699,#21700,#21701,
#21702,#21703,#21704,#21705,#21706,#21707,#21708,#21709,#21710,#21711,#21712,
#21713,#21714,#21715,#21716,#21717,#21718,#21719,#21720,#21721,#21722,#21723,
#21724,#21725,#21726,#21727,#21728,#21729,#21730,#21731,#21732,#21733,#21734,
#21735,#21736,#21737,#21738,#21739,#21740,#21741,#21742,#21743,#21744,#21745,
#21746,#21747,#21748,#21749,#21750,#21751,#21752,#21753,#21754,#21755,#21756,
#21757,#21758,#21759,#21760,#21761,#21762,#21763,#21764,#21765,#21766,#21767,
#21768,#21769,#21770,#21771,#21772,#21773,#21774,#21775,#21776,#21777,#21778,
#21779,#21780,#21781,#21782,#21783,#21784,#21785,#21786,#21787,#21788,#21789,
#21790,#21791,#21792,#21793,#21794,#21795,#21796,#21797,#21798,#21799,#21800,
#21801,#21802,#21803,#21804,#21805,#21806,#21807,#21808,#21809,#21810,#21811,
#21812,#21813,#21814,#21815,#21816,#21817,#21818,#21819,#21820,#21821,#21822,
#21823,#21824,#21825,#21826,#21827,#21828,#21829,#21830,#21831,#21832,#21833,
#21834,#21835,#21836,#21837,#21838,#21839,#21840,#21841,#21842,#21843,#21844,
#21845,#21846,#21847,#21848,#21849,#21850,#21851,#21852,#21853,#21854,#21855,
#21856,#21857,#21858,#21859,#21860,#21861,#21862,#21863,#21864,#21865,#21866,
#21867,#21868,#21869,#21870,#21871,#21872,#21873,#21874,#21875,#21876,#21877,
#21878,#21879,#21880,#21881,#21882,#21883,#21884,#21885,#21886,#21887,#21888,
#21889,#21890,#21891,#21892,#21893,#21894,#21895,#21896,#21897,#21898,#21899,
#21900,#21901,#21902,#21903,#21904,#21905,#21906,#21907,#21908,#21909,#21910,
#21911,#21912,#21913,#21914,#21915,#21916,#21917,#21918,#21919,#21920,#21921,
#21922,#21923,#21924,#21925,#21926,#21927,#21928,#21929,#21930,#21931,#21932,
#21933,#21934,#21935,#21936,#21937,#21938,#21939,#21940,#21941,#21942,#21943,
#21944,#21945,#21946,#21947,#21948,#21949,#21950,#21951,#21952,#21953,#21954,
#21955,#21956,#21957,#21958,#21959,#21960,#21961,#21962,#21963,#21964,#21965,
#21966,#21967,#21968,#21969,#21970,#21971,#21972,#21973,#21974,#21975,#21976,
#21977));
#4681=EDGE_LOOP('',(#21978));
#4682=EDGE_LOOP('',(#21979));
#4683=EDGE_LOOP('',(#21980));
#4684=EDGE_LOOP('',(#21981));
#4685=EDGE_LOOP('',(#21982));
#4686=EDGE_LOOP('',(#21983));
#4687=EDGE_LOOP('',(#21984));
#4688=EDGE_LOOP('',(#21985));
#4689=EDGE_LOOP('',(#21986));
#4690=EDGE_LOOP('',(#21987));
#4691=EDGE_LOOP('',(#21988,#21989,#21990,#21991,#21992,#21993,#21994,#21995,
#21996,#21997,#21998,#21999,#22000,#22001,#22002,#22003,#22004,#22005,#22006,
#22007,#22008,#22009,#22010,#22011,#22012,#22013,#22014,#22015,#22016,#22017,
#22018,#22019,#22020,#22021,#22022,#22023,#22024,#22025,#22026,#22027,#22028,
#22029,#22030,#22031,#22032,#22033,#22034,#22035,#22036,#22037,#22038,#22039,
#22040,#22041,#22042,#22043,#22044,#22045,#22046,#22047,#22048,#22049,#22050,
#22051,#22052,#22053,#22054,#22055,#22056,#22057,#22058,#22059,#22060,#22061,
#22062,#22063,#22064,#22065,#22066,#22067,#22068,#22069,#22070,#22071,#22072,
#22073,#22074,#22075,#22076,#22077,#22078,#22079,#22080,#22081,#22082,#22083,
#22084,#22085,#22086,#22087,#22088,#22089,#22090,#22091,#22092,#22093,#22094,
#22095,#22096,#22097,#22098,#22099,#22100,#22101,#22102,#22103,#22104,#22105,
#22106,#22107,#22108,#22109,#22110,#22111,#22112,#22113,#22114,#22115,#22116,
#22117,#22118,#22119,#22120,#22121,#22122,#22123,#22124,#22125,#22126,#22127,
#22128,#22129,#22130,#22131,#22132,#22133,#22134,#22135,#22136,#22137,#22138,
#22139,#22140,#22141,#22142,#22143,#22144,#22145,#22146,#22147,#22148,#22149,
#22150,#22151,#22152,#22153,#22154,#22155,#22156,#22157,#22158,#22159,#22160,
#22161,#22162,#22163,#22164,#22165,#22166,#22167,#22168,#22169,#22170,#22171,
#22172,#22173,#22174,#22175,#22176,#22177,#22178,#22179,#22180,#22181,#22182,
#22183,#22184,#22185,#22186,#22187,#22188,#22189,#22190,#22191,#22192,#22193,
#22194,#22195,#22196,#22197,#22198,#22199,#22200,#22201,#22202,#22203,#22204,
#22205,#22206,#22207,#22208,#22209,#22210,#22211,#22212,#22213,#22214,#22215,
#22216,#22217,#22218,#22219,#22220,#22221,#22222,#22223,#22224,#22225,#22226,
#22227,#22228,#22229,#22230,#22231,#22232,#22233,#22234,#22235,#22236,#22237,
#22238,#22239,#22240,#22241,#22242,#22243,#22244,#22245,#22246,#22247,#22248,
#22249,#22250,#22251,#22252,#22253,#22254,#22255,#22256,#22257,#22258,#22259,
#22260,#22261,#22262,#22263,#22264,#22265,#22266,#22267,#22268,#22269,#22270,
#22271));
#4692=EDGE_LOOP('',(#22272));
#4693=EDGE_LOOP('',(#22273));
#4694=EDGE_LOOP('',(#22274));
#4695=EDGE_LOOP('',(#22275));
#4696=EDGE_LOOP('',(#22276));
#4697=EDGE_LOOP('',(#22277));
#4698=EDGE_LOOP('',(#22278));
#4699=EDGE_LOOP('',(#22279));
#4700=EDGE_LOOP('',(#22280));
#4701=EDGE_LOOP('',(#22281));
#6115=LINE('',#50944,#8626);
#6116=LINE('',#50946,#8627);
#6117=LINE('',#50948,#8628);
#6118=LINE('',#50949,#8629);
#6119=LINE('',#50953,#8630);
#6120=LINE('',#50959,#8631);
#6121=LINE('',#50960,#8632);
#6122=LINE('',#50961,#8633);
#6123=LINE('',#50965,#8634);
#6124=LINE('',#50971,#8635);
#6125=LINE('',#50972,#8636);
#6126=LINE('',#50973,#8637);
#6127=LINE('',#50976,#8638);
#6128=LINE('',#50978,#8639);
#6129=LINE('',#50979,#8640);
#6130=LINE('',#50982,#8641);
#6131=LINE('',#50986,#8642);
#6132=LINE('',#50987,#8643);
#6133=LINE('',#50990,#8644);
#6134=LINE('',#50994,#8645);
#6135=LINE('',#50995,#8646);
#6136=LINE('',#50998,#8647);
#6137=LINE('',#51000,#8648);
#6138=LINE('',#51001,#8649);
#6139=LINE('',#51004,#8650);
#6140=LINE('',#51008,#8651);
#6141=LINE('',#51009,#8652);
#6142=LINE('',#51012,#8653);
#6143=LINE('',#51016,#8654);
#6144=LINE('',#51017,#8655);
#6145=LINE('',#51022,#8656);
#6146=LINE('',#51028,#8657);
#6147=LINE('',#51034,#8658);
#6148=LINE('',#51040,#8659);
#6149=LINE('',#51046,#8660);
#6150=LINE('',#51052,#8661);
#6151=LINE('',#51058,#8662);
#6152=LINE('',#51064,#8663);
#6153=LINE('',#51070,#8664);
#6154=LINE('',#51076,#8665);
#6155=LINE('',#51080,#8666);
#6156=LINE('',#51082,#8667);
#6157=LINE('',#51083,#8668);
#6158=LINE('',#51086,#8669);
#6159=LINE('',#51088,#8670);
#6160=LINE('',#51089,#8671);
#6161=LINE('',#51092,#8672);
#6162=LINE('',#51094,#8673);
#6163=LINE('',#51095,#8674);
#6164=LINE('',#51098,#8675);
#6165=LINE('',#51100,#8676);
#6166=LINE('',#51101,#8677);
#6167=LINE('',#51104,#8678);
#6168=LINE('',#51106,#8679);
#6169=LINE('',#51107,#8680);
#6170=LINE('',#51110,#8681);
#6171=LINE('',#51112,#8682);
#6172=LINE('',#51113,#8683);
#6173=LINE('',#51116,#8684);
#6174=LINE('',#51118,#8685);
#6175=LINE('',#51119,#8686);
#6176=LINE('',#51122,#8687);
#6177=LINE('',#51124,#8688);
#6178=LINE('',#51125,#8689);
#6179=LINE('',#51128,#8690);
#6180=LINE('',#51130,#8691);
#6181=LINE('',#51131,#8692);
#6182=LINE('',#51134,#8693);
#6183=LINE('',#51136,#8694);
#6184=LINE('',#51137,#8695);
#6185=LINE('',#51140,#8696);
#6186=LINE('',#51142,#8697);
#6187=LINE('',#51143,#8698);
#6188=LINE('',#51146,#8699);
#6189=LINE('',#51148,#8700);
#6190=LINE('',#51149,#8701);
#6191=LINE('',#51152,#8702);
#6192=LINE('',#51154,#8703);
#6193=LINE('',#51155,#8704);
#6194=LINE('',#51158,#8705);
#6195=LINE('',#51160,#8706);
#6196=LINE('',#51161,#8707);
#6197=LINE('',#51164,#8708);
#6198=LINE('',#51166,#8709);
#6199=LINE('',#51167,#8710);
#6200=LINE('',#51170,#8711);
#6201=LINE('',#51172,#8712);
#6202=LINE('',#51173,#8713);
#6203=LINE('',#51176,#8714);
#6204=LINE('',#51178,#8715);
#6205=LINE('',#51179,#8716);
#6206=LINE('',#51182,#8717);
#6207=LINE('',#51184,#8718);
#6208=LINE('',#51185,#8719);
#6209=LINE('',#51188,#8720);
#6210=LINE('',#51190,#8721);
#6211=LINE('',#51191,#8722);
#6212=LINE('',#51194,#8723);
#6213=LINE('',#51196,#8724);
#6214=LINE('',#51197,#8725);
#6215=LINE('',#51200,#8726);
#6216=LINE('',#51202,#8727);
#6217=LINE('',#51203,#8728);
#6218=LINE('',#51206,#8729);
#6219=LINE('',#51208,#8730);
#6220=LINE('',#51209,#8731);
#6221=LINE('',#51212,#8732);
#6222=LINE('',#51214,#8733);
#6223=LINE('',#51215,#8734);
#6224=LINE('',#51218,#8735);
#6225=LINE('',#51220,#8736);
#6226=LINE('',#51221,#8737);
#6227=LINE('',#51224,#8738);
#6228=LINE('',#51226,#8739);
#6229=LINE('',#51227,#8740);
#6230=LINE('',#51230,#8741);
#6231=LINE('',#51232,#8742);
#6232=LINE('',#51233,#8743);
#6233=LINE('',#51236,#8744);
#6234=LINE('',#51238,#8745);
#6235=LINE('',#51239,#8746);
#6236=LINE('',#51242,#8747);
#6237=LINE('',#51244,#8748);
#6238=LINE('',#51245,#8749);
#6239=LINE('',#51248,#8750);
#6240=LINE('',#51250,#8751);
#6241=LINE('',#51251,#8752);
#6242=LINE('',#51254,#8753);
#6243=LINE('',#51256,#8754);
#6244=LINE('',#51257,#8755);
#6245=LINE('',#51260,#8756);
#6246=LINE('',#51262,#8757);
#6247=LINE('',#51263,#8758);
#6248=LINE('',#51266,#8759);
#6249=LINE('',#51268,#8760);
#6250=LINE('',#51269,#8761);
#6251=LINE('',#51272,#8762);
#6252=LINE('',#51274,#8763);
#6253=LINE('',#51275,#8764);
#6254=LINE('',#51278,#8765);
#6255=LINE('',#51280,#8766);
#6256=LINE('',#51281,#8767);
#6257=LINE('',#51284,#8768);
#6258=LINE('',#51286,#8769);
#6259=LINE('',#51287,#8770);
#6260=LINE('',#51290,#8771);
#6261=LINE('',#51292,#8772);
#6262=LINE('',#51293,#8773);
#6263=LINE('',#51296,#8774);
#6264=LINE('',#51298,#8775);
#6265=LINE('',#51299,#8776);
#6266=LINE('',#51302,#8777);
#6267=LINE('',#51304,#8778);
#6268=LINE('',#51305,#8779);
#6269=LINE('',#51308,#8780);
#6270=LINE('',#51310,#8781);
#6271=LINE('',#51311,#8782);
#6272=LINE('',#51314,#8783);
#6273=LINE('',#51316,#8784);
#6274=LINE('',#51317,#8785);
#6275=LINE('',#51320,#8786);
#6276=LINE('',#51322,#8787);
#6277=LINE('',#51323,#8788);
#6278=LINE('',#51326,#8789);
#6279=LINE('',#51328,#8790);
#6280=LINE('',#51329,#8791);
#6281=LINE('',#51332,#8792);
#6282=LINE('',#51334,#8793);
#6283=LINE('',#51335,#8794);
#6284=LINE('',#51338,#8795);
#6285=LINE('',#51340,#8796);
#6286=LINE('',#51341,#8797);
#6287=LINE('',#51344,#8798);
#6288=LINE('',#51346,#8799);
#6289=LINE('',#51347,#8800);
#6290=LINE('',#51350,#8801);
#6291=LINE('',#51352,#8802);
#6292=LINE('',#51353,#8803);
#6293=LINE('',#51356,#8804);
#6294=LINE('',#51358,#8805);
#6295=LINE('',#51359,#8806);
#6296=LINE('',#51362,#8807);
#6297=LINE('',#51364,#8808);
#6298=LINE('',#51365,#8809);
#6299=LINE('',#51368,#8810);
#6300=LINE('',#51370,#8811);
#6301=LINE('',#51371,#8812);
#6302=LINE('',#51374,#8813);
#6303=LINE('',#51376,#8814);
#6304=LINE('',#51377,#8815);
#6305=LINE('',#51380,#8816);
#6306=LINE('',#51382,#8817);
#6307=LINE('',#51383,#8818);
#6308=LINE('',#51386,#8819);
#6309=LINE('',#51388,#8820);
#6310=LINE('',#51389,#8821);
#6311=LINE('',#51392,#8822);
#6312=LINE('',#51394,#8823);
#6313=LINE('',#51395,#8824);
#6314=LINE('',#51398,#8825);
#6315=LINE('',#51400,#8826);
#6316=LINE('',#51401,#8827);
#6317=LINE('',#51404,#8828);
#6318=LINE('',#51406,#8829);
#6319=LINE('',#51407,#8830);
#6320=LINE('',#51410,#8831);
#6321=LINE('',#51412,#8832);
#6322=LINE('',#51413,#8833);
#6323=LINE('',#51416,#8834);
#6324=LINE('',#51418,#8835);
#6325=LINE('',#51419,#8836);
#6326=LINE('',#51422,#8837);
#6327=LINE('',#51424,#8838);
#6328=LINE('',#51425,#8839);
#6329=LINE('',#51428,#8840);
#6330=LINE('',#51430,#8841);
#6331=LINE('',#51431,#8842);
#6332=LINE('',#51434,#8843);
#6333=LINE('',#51436,#8844);
#6334=LINE('',#51437,#8845);
#6335=LINE('',#51440,#8846);
#6336=LINE('',#51442,#8847);
#6337=LINE('',#51443,#8848);
#6338=LINE('',#51446,#8849);
#6339=LINE('',#51448,#8850);
#6340=LINE('',#51449,#8851);
#6341=LINE('',#51452,#8852);
#6342=LINE('',#51454,#8853);
#6343=LINE('',#51455,#8854);
#6344=LINE('',#51458,#8855);
#6345=LINE('',#51460,#8856);
#6346=LINE('',#51461,#8857);
#6347=LINE('',#51464,#8858);
#6348=LINE('',#51466,#8859);
#6349=LINE('',#51467,#8860);
#6350=LINE('',#51470,#8861);
#6351=LINE('',#51472,#8862);
#6352=LINE('',#51473,#8863);
#6353=LINE('',#51476,#8864);
#6354=LINE('',#51478,#8865);
#6355=LINE('',#51479,#8866);
#6356=LINE('',#51482,#8867);
#6357=LINE('',#51484,#8868);
#6358=LINE('',#51485,#8869);
#6359=LINE('',#51488,#8870);
#6360=LINE('',#51490,#8871);
#6361=LINE('',#51491,#8872);
#6362=LINE('',#51494,#8873);
#6363=LINE('',#51496,#8874);
#6364=LINE('',#51497,#8875);
#6365=LINE('',#51500,#8876);
#6366=LINE('',#51502,#8877);
#6367=LINE('',#51503,#8878);
#6368=LINE('',#51506,#8879);
#6369=LINE('',#51508,#8880);
#6370=LINE('',#51509,#8881);
#6371=LINE('',#51512,#8882);
#6372=LINE('',#51514,#8883);
#6373=LINE('',#51515,#8884);
#6374=LINE('',#51518,#8885);
#6375=LINE('',#51520,#8886);
#6376=LINE('',#51521,#8887);
#6377=LINE('',#51524,#8888);
#6378=LINE('',#51526,#8889);
#6379=LINE('',#51527,#8890);
#6380=LINE('',#51530,#8891);
#6381=LINE('',#51532,#8892);
#6382=LINE('',#51533,#8893);
#6383=LINE('',#51536,#8894);
#6384=LINE('',#51538,#8895);
#6385=LINE('',#51539,#8896);
#6386=LINE('',#51542,#8897);
#6387=LINE('',#51544,#8898);
#6388=LINE('',#51545,#8899);
#6389=LINE('',#51548,#8900);
#6390=LINE('',#51550,#8901);
#6391=LINE('',#51551,#8902);
#6392=LINE('',#51554,#8903);
#6393=LINE('',#51556,#8904);
#6394=LINE('',#51557,#8905);
#6395=LINE('',#51560,#8906);
#6396=LINE('',#51562,#8907);
#6397=LINE('',#51563,#8908);
#6398=LINE('',#51566,#8909);
#6399=LINE('',#51568,#8910);
#6400=LINE('',#51569,#8911);
#6401=LINE('',#51572,#8912);
#6402=LINE('',#51574,#8913);
#6403=LINE('',#51575,#8914);
#6404=LINE('',#51578,#8915);
#6405=LINE('',#51580,#8916);
#6406=LINE('',#51581,#8917);
#6407=LINE('',#51584,#8918);
#6408=LINE('',#51586,#8919);
#6409=LINE('',#51587,#8920);
#6410=LINE('',#51590,#8921);
#6411=LINE('',#51592,#8922);
#6412=LINE('',#51593,#8923);
#6413=LINE('',#51596,#8924);
#6414=LINE('',#51598,#8925);
#6415=LINE('',#51599,#8926);
#6416=LINE('',#51602,#8927);
#6417=LINE('',#51604,#8928);
#6418=LINE('',#51605,#8929);
#6419=LINE('',#51608,#8930);
#6420=LINE('',#51610,#8931);
#6421=LINE('',#51611,#8932);
#6422=LINE('',#51614,#8933);
#6423=LINE('',#51616,#8934);
#6424=LINE('',#51617,#8935);
#6425=LINE('',#51620,#8936);
#6426=LINE('',#51622,#8937);
#6427=LINE('',#51623,#8938);
#6428=LINE('',#51626,#8939);
#6429=LINE('',#51628,#8940);
#6430=LINE('',#51629,#8941);
#6431=LINE('',#51632,#8942);
#6432=LINE('',#51634,#8943);
#6433=LINE('',#51635,#8944);
#6434=LINE('',#51638,#8945);
#6435=LINE('',#51640,#8946);
#6436=LINE('',#51641,#8947);
#6437=LINE('',#51644,#8948);
#6438=LINE('',#51646,#8949);
#6439=LINE('',#51647,#8950);
#6440=LINE('',#51650,#8951);
#6441=LINE('',#51652,#8952);
#6442=LINE('',#51653,#8953);
#6443=LINE('',#51656,#8954);
#6444=LINE('',#51658,#8955);
#6445=LINE('',#51659,#8956);
#6446=LINE('',#51662,#8957);
#6447=LINE('',#51664,#8958);
#6448=LINE('',#51665,#8959);
#6449=LINE('',#51668,#8960);
#6450=LINE('',#51670,#8961);
#6451=LINE('',#51671,#8962);
#6452=LINE('',#51674,#8963);
#6453=LINE('',#51676,#8964);
#6454=LINE('',#51677,#8965);
#6455=LINE('',#51680,#8966);
#6456=LINE('',#51682,#8967);
#6457=LINE('',#51683,#8968);
#6458=LINE('',#51686,#8969);
#6459=LINE('',#51688,#8970);
#6460=LINE('',#51689,#8971);
#6461=LINE('',#51692,#8972);
#6462=LINE('',#51694,#8973);
#6463=LINE('',#51695,#8974);
#6464=LINE('',#51698,#8975);
#6465=LINE('',#51700,#8976);
#6466=LINE('',#51701,#8977);
#6467=LINE('',#51704,#8978);
#6468=LINE('',#51706,#8979);
#6469=LINE('',#51707,#8980);
#6470=LINE('',#51710,#8981);
#6471=LINE('',#51712,#8982);
#6472=LINE('',#51713,#8983);
#6473=LINE('',#51716,#8984);
#6474=LINE('',#51718,#8985);
#6475=LINE('',#51719,#8986);
#6476=LINE('',#51722,#8987);
#6477=LINE('',#51724,#8988);
#6478=LINE('',#51725,#8989);
#6479=LINE('',#51728,#8990);
#6480=LINE('',#51730,#8991);
#6481=LINE('',#51731,#8992);
#6482=LINE('',#51734,#8993);
#6483=LINE('',#51736,#8994);
#6484=LINE('',#51737,#8995);
#6485=LINE('',#51740,#8996);
#6486=LINE('',#51742,#8997);
#6487=LINE('',#51743,#8998);
#6488=LINE('',#51746,#8999);
#6489=LINE('',#51748,#9000);
#6490=LINE('',#51749,#9001);
#6491=LINE('',#51752,#9002);
#6492=LINE('',#51754,#9003);
#6493=LINE('',#51755,#9004);
#6494=LINE('',#51758,#9005);
#6495=LINE('',#51760,#9006);
#6496=LINE('',#51761,#9007);
#6497=LINE('',#51764,#9008);
#6498=LINE('',#51766,#9009);
#6499=LINE('',#51767,#9010);
#6500=LINE('',#51770,#9011);
#6501=LINE('',#51772,#9012);
#6502=LINE('',#51773,#9013);
#6503=LINE('',#51776,#9014);
#6504=LINE('',#51778,#9015);
#6505=LINE('',#51779,#9016);
#6506=LINE('',#51782,#9017);
#6507=LINE('',#51784,#9018);
#6508=LINE('',#51785,#9019);
#6509=LINE('',#51788,#9020);
#6510=LINE('',#51790,#9021);
#6511=LINE('',#51791,#9022);
#6512=LINE('',#51794,#9023);
#6513=LINE('',#51796,#9024);
#6514=LINE('',#51797,#9025);
#6515=LINE('',#51800,#9026);
#6516=LINE('',#51802,#9027);
#6517=LINE('',#51803,#9028);
#6518=LINE('',#51806,#9029);
#6519=LINE('',#51808,#9030);
#6520=LINE('',#51809,#9031);
#6521=LINE('',#51812,#9032);
#6522=LINE('',#51814,#9033);
#6523=LINE('',#51815,#9034);
#6524=LINE('',#51818,#9035);
#6525=LINE('',#51820,#9036);
#6526=LINE('',#51821,#9037);
#6527=LINE('',#51824,#9038);
#6528=LINE('',#51826,#9039);
#6529=LINE('',#51827,#9040);
#6530=LINE('',#51830,#9041);
#6531=LINE('',#51832,#9042);
#6532=LINE('',#51833,#9043);
#6533=LINE('',#51836,#9044);
#6534=LINE('',#51838,#9045);
#6535=LINE('',#51839,#9046);
#6536=LINE('',#51842,#9047);
#6537=LINE('',#51844,#9048);
#6538=LINE('',#51845,#9049);
#6539=LINE('',#51848,#9050);
#6540=LINE('',#51850,#9051);
#6541=LINE('',#51851,#9052);
#6542=LINE('',#51854,#9053);
#6543=LINE('',#51856,#9054);
#6544=LINE('',#51857,#9055);
#6545=LINE('',#51860,#9056);
#6546=LINE('',#51862,#9057);
#6547=LINE('',#51863,#9058);
#6548=LINE('',#51866,#9059);
#6549=LINE('',#51868,#9060);
#6550=LINE('',#51869,#9061);
#6551=LINE('',#51872,#9062);
#6552=LINE('',#51874,#9063);
#6553=LINE('',#51875,#9064);
#6554=LINE('',#51878,#9065);
#6555=LINE('',#51880,#9066);
#6556=LINE('',#51881,#9067);
#6557=LINE('',#51884,#9068);
#6558=LINE('',#51886,#9069);
#6559=LINE('',#51887,#9070);
#6560=LINE('',#51890,#9071);
#6561=LINE('',#51892,#9072);
#6562=LINE('',#51893,#9073);
#6563=LINE('',#51896,#9074);
#6564=LINE('',#51898,#9075);
#6565=LINE('',#51899,#9076);
#6566=LINE('',#51902,#9077);
#6567=LINE('',#51904,#9078);
#6568=LINE('',#51905,#9079);
#6569=LINE('',#51908,#9080);
#6570=LINE('',#51910,#9081);
#6571=LINE('',#51911,#9082);
#6572=LINE('',#51914,#9083);
#6573=LINE('',#51916,#9084);
#6574=LINE('',#51917,#9085);
#6575=LINE('',#51920,#9086);
#6576=LINE('',#51922,#9087);
#6577=LINE('',#51923,#9088);
#6578=LINE('',#51926,#9089);
#6579=LINE('',#51928,#9090);
#6580=LINE('',#51929,#9091);
#6581=LINE('',#51932,#9092);
#6582=LINE('',#51934,#9093);
#6583=LINE('',#51935,#9094);
#6584=LINE('',#51938,#9095);
#6585=LINE('',#51940,#9096);
#6586=LINE('',#51941,#9097);
#6587=LINE('',#51944,#9098);
#6588=LINE('',#51946,#9099);
#6589=LINE('',#51947,#9100);
#6590=LINE('',#51950,#9101);
#6591=LINE('',#51952,#9102);
#6592=LINE('',#51953,#9103);
#6593=LINE('',#51956,#9104);
#6594=LINE('',#51958,#9105);
#6595=LINE('',#51959,#9106);
#6596=LINE('',#51962,#9107);
#6597=LINE('',#51964,#9108);
#6598=LINE('',#51965,#9109);
#6599=LINE('',#51968,#9110);
#6600=LINE('',#51970,#9111);
#6601=LINE('',#51971,#9112);
#6602=LINE('',#51974,#9113);
#6603=LINE('',#51976,#9114);
#6604=LINE('',#51977,#9115);
#6605=LINE('',#51980,#9116);
#6606=LINE('',#51982,#9117);
#6607=LINE('',#51983,#9118);
#6608=LINE('',#51986,#9119);
#6609=LINE('',#51988,#9120);
#6610=LINE('',#51989,#9121);
#6611=LINE('',#51992,#9122);
#6612=LINE('',#51994,#9123);
#6613=LINE('',#51995,#9124);
#6614=LINE('',#51998,#9125);
#6615=LINE('',#52000,#9126);
#6616=LINE('',#52001,#9127);
#6617=LINE('',#52004,#9128);
#6618=LINE('',#52006,#9129);
#6619=LINE('',#52007,#9130);
#6620=LINE('',#52010,#9131);
#6621=LINE('',#52012,#9132);
#6622=LINE('',#52013,#9133);
#6623=LINE('',#52016,#9134);
#6624=LINE('',#52018,#9135);
#6625=LINE('',#52019,#9136);
#6626=LINE('',#52022,#9137);
#6627=LINE('',#52024,#9138);
#6628=LINE('',#52025,#9139);
#6629=LINE('',#52028,#9140);
#6630=LINE('',#52030,#9141);
#6631=LINE('',#52031,#9142);
#6632=LINE('',#52034,#9143);
#6633=LINE('',#52036,#9144);
#6634=LINE('',#52037,#9145);
#6635=LINE('',#52040,#9146);
#6636=LINE('',#52042,#9147);
#6637=LINE('',#52043,#9148);
#6638=LINE('',#52046,#9149);
#6639=LINE('',#52048,#9150);
#6640=LINE('',#52049,#9151);
#6641=LINE('',#52052,#9152);
#6642=LINE('',#52054,#9153);
#6643=LINE('',#52055,#9154);
#6644=LINE('',#52058,#9155);
#6645=LINE('',#52060,#9156);
#6646=LINE('',#52061,#9157);
#6647=LINE('',#52064,#9158);
#6648=LINE('',#52066,#9159);
#6649=LINE('',#52067,#9160);
#6650=LINE('',#52070,#9161);
#6651=LINE('',#52072,#9162);
#6652=LINE('',#52073,#9163);
#6653=LINE('',#52076,#9164);
#6654=LINE('',#52078,#9165);
#6655=LINE('',#52079,#9166);
#6656=LINE('',#52082,#9167);
#6657=LINE('',#52084,#9168);
#6658=LINE('',#52085,#9169);
#6659=LINE('',#52088,#9170);
#6660=LINE('',#52090,#9171);
#6661=LINE('',#52091,#9172);
#6662=LINE('',#52094,#9173);
#6663=LINE('',#52096,#9174);
#6664=LINE('',#52097,#9175);
#6665=LINE('',#52100,#9176);
#6666=LINE('',#52102,#9177);
#6667=LINE('',#52103,#9178);
#6668=LINE('',#52106,#9179);
#6669=LINE('',#52108,#9180);
#6670=LINE('',#52109,#9181);
#6671=LINE('',#52112,#9182);
#6672=LINE('',#52114,#9183);
#6673=LINE('',#52115,#9184);
#6674=LINE('',#52118,#9185);
#6675=LINE('',#52120,#9186);
#6676=LINE('',#52121,#9187);
#6677=LINE('',#52124,#9188);
#6678=LINE('',#52126,#9189);
#6679=LINE('',#52127,#9190);
#6680=LINE('',#52130,#9191);
#6681=LINE('',#52132,#9192);
#6682=LINE('',#52133,#9193);
#6683=LINE('',#52136,#9194);
#6684=LINE('',#52138,#9195);
#6685=LINE('',#52139,#9196);
#6686=LINE('',#52142,#9197);
#6687=LINE('',#52144,#9198);
#6688=LINE('',#52145,#9199);
#6689=LINE('',#52148,#9200);
#6690=LINE('',#52150,#9201);
#6691=LINE('',#52151,#9202);
#6692=LINE('',#52154,#9203);
#6693=LINE('',#52156,#9204);
#6694=LINE('',#52157,#9205);
#6695=LINE('',#52160,#9206);
#6696=LINE('',#52162,#9207);
#6697=LINE('',#52163,#9208);
#6698=LINE('',#52166,#9209);
#6699=LINE('',#52168,#9210);
#6700=LINE('',#52169,#9211);
#6701=LINE('',#52172,#9212);
#6702=LINE('',#52174,#9213);
#6703=LINE('',#52175,#9214);
#6704=LINE('',#52178,#9215);
#6705=LINE('',#52180,#9216);
#6706=LINE('',#52181,#9217);
#6707=LINE('',#52184,#9218);
#6708=LINE('',#52186,#9219);
#6709=LINE('',#52187,#9220);
#6710=LINE('',#52190,#9221);
#6711=LINE('',#52192,#9222);
#6712=LINE('',#52193,#9223);
#6713=LINE('',#52196,#9224);
#6714=LINE('',#52198,#9225);
#6715=LINE('',#52199,#9226);
#6716=LINE('',#52202,#9227);
#6717=LINE('',#52204,#9228);
#6718=LINE('',#52205,#9229);
#6719=LINE('',#52208,#9230);
#6720=LINE('',#52210,#9231);
#6721=LINE('',#52211,#9232);
#6722=LINE('',#52214,#9233);
#6723=LINE('',#52216,#9234);
#6724=LINE('',#52217,#9235);
#6725=LINE('',#52220,#9236);
#6726=LINE('',#52222,#9237);
#6727=LINE('',#52223,#9238);
#6728=LINE('',#52226,#9239);
#6729=LINE('',#52228,#9240);
#6730=LINE('',#52229,#9241);
#6731=LINE('',#52232,#9242);
#6732=LINE('',#52234,#9243);
#6733=LINE('',#52235,#9244);
#6734=LINE('',#52238,#9245);
#6735=LINE('',#52240,#9246);
#6736=LINE('',#52241,#9247);
#6737=LINE('',#52244,#9248);
#6738=LINE('',#52246,#9249);
#6739=LINE('',#52247,#9250);
#6740=LINE('',#52250,#9251);
#6741=LINE('',#52252,#9252);
#6742=LINE('',#52253,#9253);
#6743=LINE('',#52256,#9254);
#6744=LINE('',#52258,#9255);
#6745=LINE('',#52259,#9256);
#6746=LINE('',#52262,#9257);
#6747=LINE('',#52264,#9258);
#6748=LINE('',#52265,#9259);
#6749=LINE('',#52268,#9260);
#6750=LINE('',#52270,#9261);
#6751=LINE('',#52271,#9262);
#6752=LINE('',#52274,#9263);
#6753=LINE('',#52276,#9264);
#6754=LINE('',#52277,#9265);
#6755=LINE('',#52280,#9266);
#6756=LINE('',#52282,#9267);
#6757=LINE('',#52283,#9268);
#6758=LINE('',#52286,#9269);
#6759=LINE('',#52288,#9270);
#6760=LINE('',#52289,#9271);
#6761=LINE('',#52292,#9272);
#6762=LINE('',#52294,#9273);
#6763=LINE('',#52295,#9274);
#6764=LINE('',#52298,#9275);
#6765=LINE('',#52300,#9276);
#6766=LINE('',#52301,#9277);
#6767=LINE('',#52304,#9278);
#6768=LINE('',#52306,#9279);
#6769=LINE('',#52307,#9280);
#6770=LINE('',#52310,#9281);
#6771=LINE('',#52312,#9282);
#6772=LINE('',#52313,#9283);
#6773=LINE('',#52316,#9284);
#6774=LINE('',#52318,#9285);
#6775=LINE('',#52319,#9286);
#6776=LINE('',#52322,#9287);
#6777=LINE('',#52324,#9288);
#6778=LINE('',#52325,#9289);
#6779=LINE('',#52328,#9290);
#6780=LINE('',#52330,#9291);
#6781=LINE('',#52331,#9292);
#6782=LINE('',#52334,#9293);
#6783=LINE('',#52336,#9294);
#6784=LINE('',#52337,#9295);
#6785=LINE('',#52340,#9296);
#6786=LINE('',#52342,#9297);
#6787=LINE('',#52343,#9298);
#6788=LINE('',#52346,#9299);
#6789=LINE('',#52348,#9300);
#6790=LINE('',#52349,#9301);
#6791=LINE('',#52352,#9302);
#6792=LINE('',#52354,#9303);
#6793=LINE('',#52355,#9304);
#6794=LINE('',#52358,#9305);
#6795=LINE('',#52360,#9306);
#6796=LINE('',#52361,#9307);
#6797=LINE('',#52364,#9308);
#6798=LINE('',#52366,#9309);
#6799=LINE('',#52367,#9310);
#6800=LINE('',#52370,#9311);
#6801=LINE('',#52372,#9312);
#6802=LINE('',#52373,#9313);
#6803=LINE('',#52376,#9314);
#6804=LINE('',#52378,#9315);
#6805=LINE('',#52379,#9316);
#6806=LINE('',#52382,#9317);
#6807=LINE('',#52384,#9318);
#6808=LINE('',#52385,#9319);
#6809=LINE('',#52388,#9320);
#6810=LINE('',#52390,#9321);
#6811=LINE('',#52391,#9322);
#6812=LINE('',#52394,#9323);
#6813=LINE('',#52396,#9324);
#6814=LINE('',#52397,#9325);
#6815=LINE('',#52400,#9326);
#6816=LINE('',#52402,#9327);
#6817=LINE('',#52403,#9328);
#6818=LINE('',#52406,#9329);
#6819=LINE('',#52408,#9330);
#6820=LINE('',#52409,#9331);
#6821=LINE('',#52412,#9332);
#6822=LINE('',#52414,#9333);
#6823=LINE('',#52415,#9334);
#6824=LINE('',#52418,#9335);
#6825=LINE('',#52420,#9336);
#6826=LINE('',#52421,#9337);
#6827=LINE('',#52424,#9338);
#6828=LINE('',#52426,#9339);
#6829=LINE('',#52427,#9340);
#6830=LINE('',#52430,#9341);
#6831=LINE('',#52432,#9342);
#6832=LINE('',#52433,#9343);
#6833=LINE('',#52436,#9344);
#6834=LINE('',#52438,#9345);
#6835=LINE('',#52439,#9346);
#6836=LINE('',#52442,#9347);
#6837=LINE('',#52444,#9348);
#6838=LINE('',#52445,#9349);
#6839=LINE('',#52448,#9350);
#6840=LINE('',#52450,#9351);
#6841=LINE('',#52451,#9352);
#6842=LINE('',#52454,#9353);
#6843=LINE('',#52456,#9354);
#6844=LINE('',#52457,#9355);
#6845=LINE('',#52460,#9356);
#6846=LINE('',#52462,#9357);
#6847=LINE('',#52463,#9358);
#6848=LINE('',#52466,#9359);
#6849=LINE('',#52468,#9360);
#6850=LINE('',#52469,#9361);
#6851=LINE('',#52472,#9362);
#6852=LINE('',#52474,#9363);
#6853=LINE('',#52475,#9364);
#6854=LINE('',#52478,#9365);
#6855=LINE('',#52480,#9366);
#6856=LINE('',#52481,#9367);
#6857=LINE('',#52484,#9368);
#6858=LINE('',#52486,#9369);
#6859=LINE('',#52487,#9370);
#6860=LINE('',#52490,#9371);
#6861=LINE('',#52492,#9372);
#6862=LINE('',#52493,#9373);
#6863=LINE('',#52496,#9374);
#6864=LINE('',#52498,#9375);
#6865=LINE('',#52499,#9376);
#6866=LINE('',#52502,#9377);
#6867=LINE('',#52504,#9378);
#6868=LINE('',#52505,#9379);
#6869=LINE('',#52508,#9380);
#6870=LINE('',#52510,#9381);
#6871=LINE('',#52511,#9382);
#6872=LINE('',#52514,#9383);
#6873=LINE('',#52516,#9384);
#6874=LINE('',#52517,#9385);
#6875=LINE('',#52520,#9386);
#6876=LINE('',#52522,#9387);
#6877=LINE('',#52523,#9388);
#6878=LINE('',#52526,#9389);
#6879=LINE('',#52528,#9390);
#6880=LINE('',#52529,#9391);
#6881=LINE('',#52532,#9392);
#6882=LINE('',#52534,#9393);
#6883=LINE('',#52535,#9394);
#6884=LINE('',#52538,#9395);
#6885=LINE('',#52540,#9396);
#6886=LINE('',#52541,#9397);
#6887=LINE('',#52544,#9398);
#6888=LINE('',#52546,#9399);
#6889=LINE('',#52547,#9400);
#6890=LINE('',#52550,#9401);
#6891=LINE('',#52552,#9402);
#6892=LINE('',#52553,#9403);
#6893=LINE('',#52556,#9404);
#6894=LINE('',#52558,#9405);
#6895=LINE('',#52559,#9406);
#6896=LINE('',#52562,#9407);
#6897=LINE('',#52564,#9408);
#6898=LINE('',#52565,#9409);
#6899=LINE('',#52568,#9410);
#6900=LINE('',#52570,#9411);
#6901=LINE('',#52571,#9412);
#6902=LINE('',#52574,#9413);
#6903=LINE('',#52576,#9414);
#6904=LINE('',#52577,#9415);
#6905=LINE('',#52580,#9416);
#6906=LINE('',#52582,#9417);
#6907=LINE('',#52583,#9418);
#6908=LINE('',#52586,#9419);
#6909=LINE('',#52588,#9420);
#6910=LINE('',#52589,#9421);
#6911=LINE('',#52592,#9422);
#6912=LINE('',#52594,#9423);
#6913=LINE('',#52595,#9424);
#6914=LINE('',#52598,#9425);
#6915=LINE('',#52600,#9426);
#6916=LINE('',#52601,#9427);
#6917=LINE('',#52604,#9428);
#6918=LINE('',#52606,#9429);
#6919=LINE('',#52607,#9430);
#6920=LINE('',#52610,#9431);
#6921=LINE('',#52612,#9432);
#6922=LINE('',#52613,#9433);
#6923=LINE('',#52616,#9434);
#6924=LINE('',#52618,#9435);
#6925=LINE('',#52619,#9436);
#6926=LINE('',#52622,#9437);
#6927=LINE('',#52624,#9438);
#6928=LINE('',#52625,#9439);
#6929=LINE('',#52628,#9440);
#6930=LINE('',#52630,#9441);
#6931=LINE('',#52631,#9442);
#6932=LINE('',#52634,#9443);
#6933=LINE('',#52636,#9444);
#6934=LINE('',#52637,#9445);
#6935=LINE('',#52640,#9446);
#6936=LINE('',#52642,#9447);
#6937=LINE('',#52643,#9448);
#6938=LINE('',#52646,#9449);
#6939=LINE('',#52648,#9450);
#6940=LINE('',#52649,#9451);
#6941=LINE('',#52652,#9452);
#6942=LINE('',#52654,#9453);
#6943=LINE('',#52655,#9454);
#6944=LINE('',#52658,#9455);
#6945=LINE('',#52660,#9456);
#6946=LINE('',#52661,#9457);
#6947=LINE('',#52664,#9458);
#6948=LINE('',#52666,#9459);
#6949=LINE('',#52667,#9460);
#6950=LINE('',#52670,#9461);
#6951=LINE('',#52672,#9462);
#6952=LINE('',#52673,#9463);
#6953=LINE('',#52676,#9464);
#6954=LINE('',#52678,#9465);
#6955=LINE('',#52679,#9466);
#6956=LINE('',#52682,#9467);
#6957=LINE('',#52684,#9468);
#6958=LINE('',#52685,#9469);
#6959=LINE('',#52688,#9470);
#6960=LINE('',#52690,#9471);
#6961=LINE('',#52691,#9472);
#6962=LINE('',#52694,#9473);
#6963=LINE('',#52696,#9474);
#6964=LINE('',#52697,#9475);
#6965=LINE('',#52700,#9476);
#6966=LINE('',#52702,#9477);
#6967=LINE('',#52703,#9478);
#6968=LINE('',#52706,#9479);
#6969=LINE('',#52708,#9480);
#6970=LINE('',#52709,#9481);
#6971=LINE('',#52712,#9482);
#6972=LINE('',#52714,#9483);
#6973=LINE('',#52715,#9484);
#6974=LINE('',#52718,#9485);
#6975=LINE('',#52720,#9486);
#6976=LINE('',#52721,#9487);
#6977=LINE('',#52724,#9488);
#6978=LINE('',#52726,#9489);
#6979=LINE('',#52727,#9490);
#6980=LINE('',#52730,#9491);
#6981=LINE('',#52732,#9492);
#6982=LINE('',#52733,#9493);
#6983=LINE('',#52736,#9494);
#6984=LINE('',#52738,#9495);
#6985=LINE('',#52739,#9496);
#6986=LINE('',#52742,#9497);
#6987=LINE('',#52744,#9498);
#6988=LINE('',#52745,#9499);
#6989=LINE('',#52747,#9500);
#6990=LINE('',#52748,#9501);
#8626=VECTOR('',#31901,10.);
#8627=VECTOR('',#31902,10.);
#8628=VECTOR('',#31903,10.);
#8629=VECTOR('',#31904,10.);
#8630=VECTOR('',#31907,10.);
#8631=VECTOR('',#31914,10.);
#8632=VECTOR('',#31915,10.);
#8633=VECTOR('',#31916,10.);
#8634=VECTOR('',#31919,10.);
#8635=VECTOR('',#31926,10.);
#8636=VECTOR('',#31927,10.);
#8637=VECTOR('',#31928,10.);
#8638=VECTOR('',#31931,10.);
#8639=VECTOR('',#31932,10.);
#8640=VECTOR('',#31933,10.);
#8641=VECTOR('',#31936,10.);
#8642=VECTOR('',#31941,10.);
#8643=VECTOR('',#31942,10.);
#8644=VECTOR('',#31945,10.);
#8645=VECTOR('',#31950,10.);
#8646=VECTOR('',#31951,10.);
#8647=VECTOR('',#31954,10.);
#8648=VECTOR('',#31955,10.);
#8649=VECTOR('',#31956,10.);
#8650=VECTOR('',#31959,10.);
#8651=VECTOR('',#31964,10.);
#8652=VECTOR('',#31965,10.);
#8653=VECTOR('',#31968,10.);
#8654=VECTOR('',#31973,10.);
#8655=VECTOR('',#31974,10.);
#8656=VECTOR('',#31979,1.778);
#8657=VECTOR('',#31986,1.778);
#8658=VECTOR('',#31993,1.778);
#8659=VECTOR('',#32000,1.778);
#8660=VECTOR('',#32007,1.778);
#8661=VECTOR('',#32014,1.778);
#8662=VECTOR('',#32021,1.778);
#8663=VECTOR('',#32028,1.778);
#8664=VECTOR('',#32035,1.778);
#8665=VECTOR('',#32042,1.778);
#8666=VECTOR('',#32047,10.);
#8667=VECTOR('',#32048,10.);
#8668=VECTOR('',#32049,10.);
#8669=VECTOR('',#32052,10.);
#8670=VECTOR('',#32053,10.);
#8671=VECTOR('',#32054,10.);
#8672=VECTOR('',#32057,10.);
#8673=VECTOR('',#32058,10.);
#8674=VECTOR('',#32059,10.);
#8675=VECTOR('',#32062,10.);
#8676=VECTOR('',#32063,10.);
#8677=VECTOR('',#32064,10.);
#8678=VECTOR('',#32067,10.);
#8679=VECTOR('',#32068,10.);
#8680=VECTOR('',#32069,10.);
#8681=VECTOR('',#32072,10.);
#8682=VECTOR('',#32073,10.);
#8683=VECTOR('',#32074,10.);
#8684=VECTOR('',#32077,10.);
#8685=VECTOR('',#32078,10.);
#8686=VECTOR('',#32079,10.);
#8687=VECTOR('',#32082,10.);
#8688=VECTOR('',#32083,10.);
#8689=VECTOR('',#32084,10.);
#8690=VECTOR('',#32087,10.);
#8691=VECTOR('',#32088,10.);
#8692=VECTOR('',#32089,10.);
#8693=VECTOR('',#32092,10.);
#8694=VECTOR('',#32093,10.);
#8695=VECTOR('',#32094,10.);
#8696=VECTOR('',#32097,10.);
#8697=VECTOR('',#32098,10.);
#8698=VECTOR('',#32099,10.);
#8699=VECTOR('',#32102,10.);
#8700=VECTOR('',#32103,10.);
#8701=VECTOR('',#32104,10.);
#8702=VECTOR('',#32107,10.);
#8703=VECTOR('',#32108,10.);
#8704=VECTOR('',#32109,10.);
#8705=VECTOR('',#32112,10.);
#8706=VECTOR('',#32113,10.);
#8707=VECTOR('',#32114,10.);
#8708=VECTOR('',#32117,10.);
#8709=VECTOR('',#32118,10.);
#8710=VECTOR('',#32119,10.);
#8711=VECTOR('',#32122,10.);
#8712=VECTOR('',#32123,10.);
#8713=VECTOR('',#32124,10.);
#8714=VECTOR('',#32127,10.);
#8715=VECTOR('',#32128,10.);
#8716=VECTOR('',#32129,10.);
#8717=VECTOR('',#32132,10.);
#8718=VECTOR('',#32133,10.);
#8719=VECTOR('',#32134,10.);
#8720=VECTOR('',#32137,10.);
#8721=VECTOR('',#32138,10.);
#8722=VECTOR('',#32139,10.);
#8723=VECTOR('',#32142,10.);
#8724=VECTOR('',#32143,10.);
#8725=VECTOR('',#32144,10.);
#8726=VECTOR('',#32147,10.);
#8727=VECTOR('',#32148,10.);
#8728=VECTOR('',#32149,10.);
#8729=VECTOR('',#32152,10.);
#8730=VECTOR('',#32153,10.);
#8731=VECTOR('',#32154,10.);
#8732=VECTOR('',#32157,10.);
#8733=VECTOR('',#32158,10.);
#8734=VECTOR('',#32159,10.);
#8735=VECTOR('',#32162,10.);
#8736=VECTOR('',#32163,10.);
#8737=VECTOR('',#32164,10.);
#8738=VECTOR('',#32167,10.);
#8739=VECTOR('',#32168,10.);
#8740=VECTOR('',#32169,10.);
#8741=VECTOR('',#32172,10.);
#8742=VECTOR('',#32173,10.);
#8743=VECTOR('',#32174,10.);
#8744=VECTOR('',#32177,10.);
#8745=VECTOR('',#32178,10.);
#8746=VECTOR('',#32179,10.);
#8747=VECTOR('',#32182,10.);
#8748=VECTOR('',#32183,10.);
#8749=VECTOR('',#32184,10.);
#8750=VECTOR('',#32187,10.);
#8751=VECTOR('',#32188,10.);
#8752=VECTOR('',#32189,10.);
#8753=VECTOR('',#32192,10.);
#8754=VECTOR('',#32193,10.);
#8755=VECTOR('',#32194,10.);
#8756=VECTOR('',#32197,10.);
#8757=VECTOR('',#32198,10.);
#8758=VECTOR('',#32199,10.);
#8759=VECTOR('',#32202,10.);
#8760=VECTOR('',#32203,10.);
#8761=VECTOR('',#32204,10.);
#8762=VECTOR('',#32207,10.);
#8763=VECTOR('',#32208,10.);
#8764=VECTOR('',#32209,10.);
#8765=VECTOR('',#32212,10.);
#8766=VECTOR('',#32213,10.);
#8767=VECTOR('',#32214,10.);
#8768=VECTOR('',#32217,10.);
#8769=VECTOR('',#32218,10.);
#8770=VECTOR('',#32219,10.);
#8771=VECTOR('',#32222,10.);
#8772=VECTOR('',#32223,10.);
#8773=VECTOR('',#32224,10.);
#8774=VECTOR('',#32227,9.99999999999999);
#8775=VECTOR('',#32228,9.99999999999999);
#8776=VECTOR('',#32229,10.);
#8777=VECTOR('',#32232,10.);
#8778=VECTOR('',#32233,10.);
#8779=VECTOR('',#32234,10.);
#8780=VECTOR('',#32237,9.99999999999999);
#8781=VECTOR('',#32238,9.99999999999999);
#8782=VECTOR('',#32239,10.);
#8783=VECTOR('',#32242,10.);
#8784=VECTOR('',#32243,10.);
#8785=VECTOR('',#32244,10.);
#8786=VECTOR('',#32247,9.99999999999999);
#8787=VECTOR('',#32248,9.99999999999999);
#8788=VECTOR('',#32249,10.);
#8789=VECTOR('',#32252,10.);
#8790=VECTOR('',#32253,10.);
#8791=VECTOR('',#32254,10.);
#8792=VECTOR('',#32257,10.);
#8793=VECTOR('',#32258,10.);
#8794=VECTOR('',#32259,10.);
#8795=VECTOR('',#32262,10.);
#8796=VECTOR('',#32263,10.);
#8797=VECTOR('',#32264,10.);
#8798=VECTOR('',#32267,10.);
#8799=VECTOR('',#32268,10.);
#8800=VECTOR('',#32269,10.);
#8801=VECTOR('',#32272,10.);
#8802=VECTOR('',#32273,10.);
#8803=VECTOR('',#32274,10.);
#8804=VECTOR('',#32277,10.);
#8805=VECTOR('',#32278,10.);
#8806=VECTOR('',#32279,10.);
#8807=VECTOR('',#32282,10.);
#8808=VECTOR('',#32283,10.);
#8809=VECTOR('',#32284,10.);
#8810=VECTOR('',#32287,10.);
#8811=VECTOR('',#32288,10.);
#8812=VECTOR('',#32289,10.);
#8813=VECTOR('',#32292,10.);
#8814=VECTOR('',#32293,10.);
#8815=VECTOR('',#32294,10.);
#8816=VECTOR('',#32297,10.);
#8817=VECTOR('',#32298,10.);
#8818=VECTOR('',#32299,10.);
#8819=VECTOR('',#32302,10.);
#8820=VECTOR('',#32303,10.);
#8821=VECTOR('',#32304,10.);
#8822=VECTOR('',#32307,10.);
#8823=VECTOR('',#32308,10.);
#8824=VECTOR('',#32309,10.);
#8825=VECTOR('',#32312,10.);
#8826=VECTOR('',#32313,10.);
#8827=VECTOR('',#32314,10.);
#8828=VECTOR('',#32317,9.99999999999999);
#8829=VECTOR('',#32318,9.99999999999999);
#8830=VECTOR('',#32319,10.);
#8831=VECTOR('',#32322,10.);
#8832=VECTOR('',#32323,10.);
#8833=VECTOR('',#32324,10.);
#8834=VECTOR('',#32327,9.99999999999999);
#8835=VECTOR('',#32328,9.99999999999999);
#8836=VECTOR('',#32329,10.);
#8837=VECTOR('',#32332,10.);
#8838=VECTOR('',#32333,10.);
#8839=VECTOR('',#32334,10.);
#8840=VECTOR('',#32337,9.99999999999999);
#8841=VECTOR('',#32338,9.99999999999999);
#8842=VECTOR('',#32339,10.);
#8843=VECTOR('',#32342,10.);
#8844=VECTOR('',#32343,10.);
#8845=VECTOR('',#32344,10.);
#8846=VECTOR('',#32347,9.99999999999999);
#8847=VECTOR('',#32348,9.99999999999999);
#8848=VECTOR('',#32349,10.);
#8849=VECTOR('',#32352,10.);
#8850=VECTOR('',#32353,10.);
#8851=VECTOR('',#32354,10.);
#8852=VECTOR('',#32357,9.99999999999999);
#8853=VECTOR('',#32358,9.99999999999999);
#8854=VECTOR('',#32359,10.);
#8855=VECTOR('',#32362,10.);
#8856=VECTOR('',#32363,10.);
#8857=VECTOR('',#32364,10.);
#8858=VECTOR('',#32367,9.99999999999999);
#8859=VECTOR('',#32368,9.99999999999999);
#8860=VECTOR('',#32369,10.);
#8861=VECTOR('',#32372,10.);
#8862=VECTOR('',#32373,10.);
#8863=VECTOR('',#32374,10.);
#8864=VECTOR('',#32377,10.);
#8865=VECTOR('',#32378,10.);
#8866=VECTOR('',#32379,10.);
#8867=VECTOR('',#32382,10.);
#8868=VECTOR('',#32383,10.);
#8869=VECTOR('',#32384,10.);
#8870=VECTOR('',#32387,10.);
#8871=VECTOR('',#32388,10.);
#8872=VECTOR('',#32389,10.);
#8873=VECTOR('',#32392,10.);
#8874=VECTOR('',#32393,10.);
#8875=VECTOR('',#32394,10.);
#8876=VECTOR('',#32397,10.);
#8877=VECTOR('',#32398,10.);
#8878=VECTOR('',#32399,10.);
#8879=VECTOR('',#32402,10.);
#8880=VECTOR('',#32403,10.);
#8881=VECTOR('',#32404,10.);
#8882=VECTOR('',#32407,10.);
#8883=VECTOR('',#32408,10.);
#8884=VECTOR('',#32409,10.);
#8885=VECTOR('',#32412,10.);
#8886=VECTOR('',#32413,10.);
#8887=VECTOR('',#32414,10.);
#8888=VECTOR('',#32417,10.);
#8889=VECTOR('',#32418,10.);
#8890=VECTOR('',#32419,10.);
#8891=VECTOR('',#32422,10.);
#8892=VECTOR('',#32423,10.);
#8893=VECTOR('',#32424,10.);
#8894=VECTOR('',#32427,10.);
#8895=VECTOR('',#32428,10.);
#8896=VECTOR('',#32429,10.);
#8897=VECTOR('',#32432,10.);
#8898=VECTOR('',#32433,10.);
#8899=VECTOR('',#32434,10.);
#8900=VECTOR('',#32437,10.);
#8901=VECTOR('',#32438,10.);
#8902=VECTOR('',#32439,10.);
#8903=VECTOR('',#32442,10.);
#8904=VECTOR('',#32443,10.);
#8905=VECTOR('',#32444,10.);
#8906=VECTOR('',#32447,10.);
#8907=VECTOR('',#32448,10.);
#8908=VECTOR('',#32449,10.);
#8909=VECTOR('',#32452,10.);
#8910=VECTOR('',#32453,10.);
#8911=VECTOR('',#32454,10.);
#8912=VECTOR('',#32457,10.);
#8913=VECTOR('',#32458,10.);
#8914=VECTOR('',#32459,10.);
#8915=VECTOR('',#32462,10.);
#8916=VECTOR('',#32463,10.);
#8917=VECTOR('',#32464,10.);
#8918=VECTOR('',#32467,10.);
#8919=VECTOR('',#32468,10.);
#8920=VECTOR('',#32469,10.);
#8921=VECTOR('',#32472,10.);
#8922=VECTOR('',#32473,10.);
#8923=VECTOR('',#32474,10.);
#8924=VECTOR('',#32477,10.);
#8925=VECTOR('',#32478,10.);
#8926=VECTOR('',#32479,10.);
#8927=VECTOR('',#32482,10.);
#8928=VECTOR('',#32483,10.);
#8929=VECTOR('',#32484,10.);
#8930=VECTOR('',#32487,10.);
#8931=VECTOR('',#32488,10.);
#8932=VECTOR('',#32489,10.);
#8933=VECTOR('',#32492,10.);
#8934=VECTOR('',#32493,10.);
#8935=VECTOR('',#32494,10.);
#8936=VECTOR('',#32497,10.);
#8937=VECTOR('',#32498,10.);
#8938=VECTOR('',#32499,10.);
#8939=VECTOR('',#32502,10.);
#8940=VECTOR('',#32503,10.);
#8941=VECTOR('',#32504,10.);
#8942=VECTOR('',#32507,10.);
#8943=VECTOR('',#32508,10.);
#8944=VECTOR('',#32509,10.);
#8945=VECTOR('',#32512,10.);
#8946=VECTOR('',#32513,10.);
#8947=VECTOR('',#32514,10.);
#8948=VECTOR('',#32517,10.);
#8949=VECTOR('',#32518,10.);
#8950=VECTOR('',#32519,10.);
#8951=VECTOR('',#32522,10.);
#8952=VECTOR('',#32523,10.);
#8953=VECTOR('',#32524,10.);
#8954=VECTOR('',#32527,10.);
#8955=VECTOR('',#32528,10.);
#8956=VECTOR('',#32529,10.);
#8957=VECTOR('',#32532,10.);
#8958=VECTOR('',#32533,10.);
#8959=VECTOR('',#32534,10.);
#8960=VECTOR('',#32537,10.);
#8961=VECTOR('',#32538,10.);
#8962=VECTOR('',#32539,10.);
#8963=VECTOR('',#32542,10.);
#8964=VECTOR('',#32543,10.);
#8965=VECTOR('',#32544,10.);
#8966=VECTOR('',#32547,10.);
#8967=VECTOR('',#32548,10.);
#8968=VECTOR('',#32549,10.);
#8969=VECTOR('',#32552,10.);
#8970=VECTOR('',#32553,10.);
#8971=VECTOR('',#32554,10.);
#8972=VECTOR('',#32557,10.);
#8973=VECTOR('',#32558,10.);
#8974=VECTOR('',#32559,10.);
#8975=VECTOR('',#32562,10.);
#8976=VECTOR('',#32563,10.);
#8977=VECTOR('',#32564,10.);
#8978=VECTOR('',#32567,10.);
#8979=VECTOR('',#32568,10.);
#8980=VECTOR('',#32569,10.);
#8981=VECTOR('',#32572,10.);
#8982=VECTOR('',#32573,10.);
#8983=VECTOR('',#32574,10.);
#8984=VECTOR('',#32577,10.);
#8985=VECTOR('',#32578,10.);
#8986=VECTOR('',#32579,10.);
#8987=VECTOR('',#32582,10.);
#8988=VECTOR('',#32583,10.);
#8989=VECTOR('',#32584,10.);
#8990=VECTOR('',#32587,10.);
#8991=VECTOR('',#32588,10.);
#8992=VECTOR('',#32589,10.);
#8993=VECTOR('',#32592,10.);
#8994=VECTOR('',#32593,10.);
#8995=VECTOR('',#32594,10.);
#8996=VECTOR('',#32597,10.);
#8997=VECTOR('',#32598,10.);
#8998=VECTOR('',#32599,10.);
#8999=VECTOR('',#32602,10.);
#9000=VECTOR('',#32603,10.);
#9001=VECTOR('',#32604,10.);
#9002=VECTOR('',#32607,10.);
#9003=VECTOR('',#32608,10.);
#9004=VECTOR('',#32609,10.);
#9005=VECTOR('',#32612,10.);
#9006=VECTOR('',#32613,10.);
#9007=VECTOR('',#32614,10.);
#9008=VECTOR('',#32617,10.);
#9009=VECTOR('',#32618,10.);
#9010=VECTOR('',#32619,10.);
#9011=VECTOR('',#32622,10.);
#9012=VECTOR('',#32623,10.);
#9013=VECTOR('',#32624,10.);
#9014=VECTOR('',#32627,10.);
#9015=VECTOR('',#32628,10.);
#9016=VECTOR('',#32629,10.);
#9017=VECTOR('',#32632,10.);
#9018=VECTOR('',#32633,10.);
#9019=VECTOR('',#32634,10.);
#9020=VECTOR('',#32637,10.);
#9021=VECTOR('',#32638,10.);
#9022=VECTOR('',#32639,10.);
#9023=VECTOR('',#32642,10.);
#9024=VECTOR('',#32643,10.);
#9025=VECTOR('',#32644,10.);
#9026=VECTOR('',#32647,10.);
#9027=VECTOR('',#32648,10.);
#9028=VECTOR('',#32649,10.);
#9029=VECTOR('',#32652,10.);
#9030=VECTOR('',#32653,10.);
#9031=VECTOR('',#32654,10.);
#9032=VECTOR('',#32657,10.);
#9033=VECTOR('',#32658,10.);
#9034=VECTOR('',#32659,10.);
#9035=VECTOR('',#32662,10.);
#9036=VECTOR('',#32663,10.);
#9037=VECTOR('',#32664,10.);
#9038=VECTOR('',#32667,10.);
#9039=VECTOR('',#32668,10.);
#9040=VECTOR('',#32669,10.);
#9041=VECTOR('',#32672,10.);
#9042=VECTOR('',#32673,10.);
#9043=VECTOR('',#32674,10.);
#9044=VECTOR('',#32677,10.);
#9045=VECTOR('',#32678,10.);
#9046=VECTOR('',#32679,10.);
#9047=VECTOR('',#32682,10.);
#9048=VECTOR('',#32683,10.);
#9049=VECTOR('',#32684,10.);
#9050=VECTOR('',#32687,10.);
#9051=VECTOR('',#32688,10.);
#9052=VECTOR('',#32689,10.);
#9053=VECTOR('',#32692,10.);
#9054=VECTOR('',#32693,10.);
#9055=VECTOR('',#32694,10.);
#9056=VECTOR('',#32697,10.);
#9057=VECTOR('',#32698,10.);
#9058=VECTOR('',#32699,10.);
#9059=VECTOR('',#32702,10.);
#9060=VECTOR('',#32703,10.);
#9061=VECTOR('',#32704,10.);
#9062=VECTOR('',#32707,10.);
#9063=VECTOR('',#32708,10.);
#9064=VECTOR('',#32709,10.);
#9065=VECTOR('',#32712,10.);
#9066=VECTOR('',#32713,10.);
#9067=VECTOR('',#32714,10.);
#9068=VECTOR('',#32717,10.);
#9069=VECTOR('',#32718,10.);
#9070=VECTOR('',#32719,10.);
#9071=VECTOR('',#32722,10.);
#9072=VECTOR('',#32723,10.);
#9073=VECTOR('',#32724,10.);
#9074=VECTOR('',#32727,10.);
#9075=VECTOR('',#32728,10.);
#9076=VECTOR('',#32729,10.);
#9077=VECTOR('',#32732,10.);
#9078=VECTOR('',#32733,10.);
#9079=VECTOR('',#32734,10.);
#9080=VECTOR('',#32737,10.);
#9081=VECTOR('',#32738,10.);
#9082=VECTOR('',#32739,10.);
#9083=VECTOR('',#32742,10.);
#9084=VECTOR('',#32743,10.);
#9085=VECTOR('',#32744,10.);
#9086=VECTOR('',#32747,10.);
#9087=VECTOR('',#32748,10.);
#9088=VECTOR('',#32749,10.);
#9089=VECTOR('',#32752,10.);
#9090=VECTOR('',#32753,10.);
#9091=VECTOR('',#32754,10.);
#9092=VECTOR('',#32757,10.);
#9093=VECTOR('',#32758,10.);
#9094=VECTOR('',#32759,10.);
#9095=VECTOR('',#32762,10.);
#9096=VECTOR('',#32763,10.);
#9097=VECTOR('',#32764,10.);
#9098=VECTOR('',#32767,10.);
#9099=VECTOR('',#32768,10.);
#9100=VECTOR('',#32769,10.);
#9101=VECTOR('',#32772,10.);
#9102=VECTOR('',#32773,10.);
#9103=VECTOR('',#32774,10.);
#9104=VECTOR('',#32777,10.);
#9105=VECTOR('',#32778,10.);
#9106=VECTOR('',#32779,10.);
#9107=VECTOR('',#32782,10.);
#9108=VECTOR('',#32783,10.);
#9109=VECTOR('',#32784,10.);
#9110=VECTOR('',#32787,10.);
#9111=VECTOR('',#32788,10.);
#9112=VECTOR('',#32789,10.);
#9113=VECTOR('',#32792,10.);
#9114=VECTOR('',#32793,10.);
#9115=VECTOR('',#32794,10.);
#9116=VECTOR('',#32797,10.);
#9117=VECTOR('',#32798,10.);
#9118=VECTOR('',#32799,10.);
#9119=VECTOR('',#32802,10.);
#9120=VECTOR('',#32803,10.);
#9121=VECTOR('',#32804,10.);
#9122=VECTOR('',#32807,10.);
#9123=VECTOR('',#32808,10.);
#9124=VECTOR('',#32809,10.);
#9125=VECTOR('',#32812,10.);
#9126=VECTOR('',#32813,10.);
#9127=VECTOR('',#32814,10.);
#9128=VECTOR('',#32817,10.);
#9129=VECTOR('',#32818,10.);
#9130=VECTOR('',#32819,10.);
#9131=VECTOR('',#32822,10.);
#9132=VECTOR('',#32823,10.);
#9133=VECTOR('',#32824,10.);
#9134=VECTOR('',#32827,10.);
#9135=VECTOR('',#32828,10.);
#9136=VECTOR('',#32829,10.);
#9137=VECTOR('',#32832,10.);
#9138=VECTOR('',#32833,10.);
#9139=VECTOR('',#32834,10.);
#9140=VECTOR('',#32837,10.);
#9141=VECTOR('',#32838,10.);
#9142=VECTOR('',#32839,10.);
#9143=VECTOR('',#32842,10.);
#9144=VECTOR('',#32843,10.);
#9145=VECTOR('',#32844,10.);
#9146=VECTOR('',#32847,10.);
#9147=VECTOR('',#32848,10.);
#9148=VECTOR('',#32849,10.);
#9149=VECTOR('',#32852,10.);
#9150=VECTOR('',#32853,10.);
#9151=VECTOR('',#32854,10.);
#9152=VECTOR('',#32857,10.);
#9153=VECTOR('',#32858,10.);
#9154=VECTOR('',#32859,10.);
#9155=VECTOR('',#32862,10.);
#9156=VECTOR('',#32863,10.);
#9157=VECTOR('',#32864,10.);
#9158=VECTOR('',#32867,10.);
#9159=VECTOR('',#32868,10.);
#9160=VECTOR('',#32869,10.);
#9161=VECTOR('',#32872,10.);
#9162=VECTOR('',#32873,10.);
#9163=VECTOR('',#32874,10.);
#9164=VECTOR('',#32877,10.);
#9165=VECTOR('',#32878,10.);
#9166=VECTOR('',#32879,10.);
#9167=VECTOR('',#32882,10.);
#9168=VECTOR('',#32883,10.);
#9169=VECTOR('',#32884,10.);
#9170=VECTOR('',#32887,10.);
#9171=VECTOR('',#32888,10.);
#9172=VECTOR('',#32889,10.);
#9173=VECTOR('',#32892,10.);
#9174=VECTOR('',#32893,10.);
#9175=VECTOR('',#32894,10.);
#9176=VECTOR('',#32897,10.);
#9177=VECTOR('',#32898,10.);
#9178=VECTOR('',#32899,10.);
#9179=VECTOR('',#32902,10.);
#9180=VECTOR('',#32903,10.);
#9181=VECTOR('',#32904,10.);
#9182=VECTOR('',#32907,10.);
#9183=VECTOR('',#32908,10.);
#9184=VECTOR('',#32909,10.);
#9185=VECTOR('',#32912,10.);
#9186=VECTOR('',#32913,10.);
#9187=VECTOR('',#32914,10.);
#9188=VECTOR('',#32917,10.);
#9189=VECTOR('',#32918,10.);
#9190=VECTOR('',#32919,10.);
#9191=VECTOR('',#32922,10.);
#9192=VECTOR('',#32923,10.);
#9193=VECTOR('',#32924,10.);
#9194=VECTOR('',#32927,10.);
#9195=VECTOR('',#32928,10.);
#9196=VECTOR('',#32929,10.);
#9197=VECTOR('',#32932,10.);
#9198=VECTOR('',#32933,10.);
#9199=VECTOR('',#32934,10.);
#9200=VECTOR('',#32937,10.);
#9201=VECTOR('',#32938,10.);
#9202=VECTOR('',#32939,10.);
#9203=VECTOR('',#32942,10.);
#9204=VECTOR('',#32943,10.);
#9205=VECTOR('',#32944,10.);
#9206=VECTOR('',#32947,10.);
#9207=VECTOR('',#32948,10.);
#9208=VECTOR('',#32949,10.);
#9209=VECTOR('',#32952,10.);
#9210=VECTOR('',#32953,10.);
#9211=VECTOR('',#32954,10.);
#9212=VECTOR('',#32957,10.);
#9213=VECTOR('',#32958,10.);
#9214=VECTOR('',#32959,10.);
#9215=VECTOR('',#32962,10.);
#9216=VECTOR('',#32963,10.);
#9217=VECTOR('',#32964,10.);
#9218=VECTOR('',#32967,10.);
#9219=VECTOR('',#32968,10.);
#9220=VECTOR('',#32969,10.);
#9221=VECTOR('',#32972,10.);
#9222=VECTOR('',#32973,10.);
#9223=VECTOR('',#32974,10.);
#9224=VECTOR('',#32977,10.);
#9225=VECTOR('',#32978,10.);
#9226=VECTOR('',#32979,10.);
#9227=VECTOR('',#32982,10.);
#9228=VECTOR('',#32983,10.);
#9229=VECTOR('',#32984,10.);
#9230=VECTOR('',#32987,10.);
#9231=VECTOR('',#32988,10.);
#9232=VECTOR('',#32989,10.);
#9233=VECTOR('',#32992,10.);
#9234=VECTOR('',#32993,10.);
#9235=VECTOR('',#32994,10.);
#9236=VECTOR('',#32997,10.);
#9237=VECTOR('',#32998,10.);
#9238=VECTOR('',#32999,10.);
#9239=VECTOR('',#33002,10.);
#9240=VECTOR('',#33003,10.);
#9241=VECTOR('',#33004,10.);
#9242=VECTOR('',#33007,10.);
#9243=VECTOR('',#33008,10.);
#9244=VECTOR('',#33009,10.);
#9245=VECTOR('',#33012,10.);
#9246=VECTOR('',#33013,10.);
#9247=VECTOR('',#33014,10.);
#9248=VECTOR('',#33017,10.);
#9249=VECTOR('',#33018,10.);
#9250=VECTOR('',#33019,10.);
#9251=VECTOR('',#33022,10.);
#9252=VECTOR('',#33023,10.);
#9253=VECTOR('',#33024,10.);
#9254=VECTOR('',#33027,10.);
#9255=VECTOR('',#33028,10.);
#9256=VECTOR('',#33029,10.);
#9257=VECTOR('',#33032,10.);
#9258=VECTOR('',#33033,10.);
#9259=VECTOR('',#33034,10.);
#9260=VECTOR('',#33037,10.);
#9261=VECTOR('',#33038,10.);
#9262=VECTOR('',#33039,10.);
#9263=VECTOR('',#33042,10.);
#9264=VECTOR('',#33043,10.);
#9265=VECTOR('',#33044,10.);
#9266=VECTOR('',#33047,10.);
#9267=VECTOR('',#33048,10.);
#9268=VECTOR('',#33049,10.);
#9269=VECTOR('',#33052,10.);
#9270=VECTOR('',#33053,10.);
#9271=VECTOR('',#33054,10.);
#9272=VECTOR('',#33057,10.);
#9273=VECTOR('',#33058,10.);
#9274=VECTOR('',#33059,10.);
#9275=VECTOR('',#33062,10.);
#9276=VECTOR('',#33063,10.);
#9277=VECTOR('',#33064,10.);
#9278=VECTOR('',#33067,10.);
#9279=VECTOR('',#33068,10.);
#9280=VECTOR('',#33069,10.);
#9281=VECTOR('',#33072,10.);
#9282=VECTOR('',#33073,10.);
#9283=VECTOR('',#33074,10.);
#9284=VECTOR('',#33077,10.);
#9285=VECTOR('',#33078,10.);
#9286=VECTOR('',#33079,10.);
#9287=VECTOR('',#33082,10.);
#9288=VECTOR('',#33083,10.);
#9289=VECTOR('',#33084,10.);
#9290=VECTOR('',#33087,10.);
#9291=VECTOR('',#33088,10.);
#9292=VECTOR('',#33089,10.);
#9293=VECTOR('',#33092,10.);
#9294=VECTOR('',#33093,10.);
#9295=VECTOR('',#33094,10.);
#9296=VECTOR('',#33097,10.);
#9297=VECTOR('',#33098,10.);
#9298=VECTOR('',#33099,10.);
#9299=VECTOR('',#33102,10.);
#9300=VECTOR('',#33103,10.);
#9301=VECTOR('',#33104,10.);
#9302=VECTOR('',#33107,10.);
#9303=VECTOR('',#33108,10.);
#9304=VECTOR('',#33109,10.);
#9305=VECTOR('',#33112,10.);
#9306=VECTOR('',#33113,10.);
#9307=VECTOR('',#33114,10.);
#9308=VECTOR('',#33117,9.99999999999999);
#9309=VECTOR('',#33118,9.99999999999999);
#9310=VECTOR('',#33119,10.);
#9311=VECTOR('',#33122,10.);
#9312=VECTOR('',#33123,10.);
#9313=VECTOR('',#33124,10.);
#9314=VECTOR('',#33127,9.99999999999999);
#9315=VECTOR('',#33128,9.99999999999999);
#9316=VECTOR('',#33129,10.);
#9317=VECTOR('',#33132,10.);
#9318=VECTOR('',#33133,10.);
#9319=VECTOR('',#33134,10.);
#9320=VECTOR('',#33137,9.99999999999999);
#9321=VECTOR('',#33138,9.99999999999999);
#9322=VECTOR('',#33139,10.);
#9323=VECTOR('',#33142,10.);
#9324=VECTOR('',#33143,10.);
#9325=VECTOR('',#33144,10.);
#9326=VECTOR('',#33147,9.99999999999999);
#9327=VECTOR('',#33148,9.99999999999999);
#9328=VECTOR('',#33149,10.);
#9329=VECTOR('',#33152,10.);
#9330=VECTOR('',#33153,10.);
#9331=VECTOR('',#33154,10.);
#9332=VECTOR('',#33157,9.99999999999999);
#9333=VECTOR('',#33158,9.99999999999999);
#9334=VECTOR('',#33159,10.);
#9335=VECTOR('',#33162,10.);
#9336=VECTOR('',#33163,10.);
#9337=VECTOR('',#33164,10.);
#9338=VECTOR('',#33167,9.99999999999999);
#9339=VECTOR('',#33168,9.99999999999999);
#9340=VECTOR('',#33169,10.);
#9341=VECTOR('',#33172,10.);
#9342=VECTOR('',#33173,10.);
#9343=VECTOR('',#33174,10.);
#9344=VECTOR('',#33177,10.);
#9345=VECTOR('',#33178,10.);
#9346=VECTOR('',#33179,10.);
#9347=VECTOR('',#33182,10.);
#9348=VECTOR('',#33183,10.);
#9349=VECTOR('',#33184,10.);
#9350=VECTOR('',#33187,10.);
#9351=VECTOR('',#33188,10.);
#9352=VECTOR('',#33189,10.);
#9353=VECTOR('',#33192,10.);
#9354=VECTOR('',#33193,10.);
#9355=VECTOR('',#33194,10.);
#9356=VECTOR('',#33197,10.);
#9357=VECTOR('',#33198,10.);
#9358=VECTOR('',#33199,10.);
#9359=VECTOR('',#33202,10.);
#9360=VECTOR('',#33203,10.);
#9361=VECTOR('',#33204,10.);
#9362=VECTOR('',#33207,10.);
#9363=VECTOR('',#33208,10.);
#9364=VECTOR('',#33209,10.);
#9365=VECTOR('',#33212,10.);
#9366=VECTOR('',#33213,10.);
#9367=VECTOR('',#33214,10.);
#9368=VECTOR('',#33217,10.);
#9369=VECTOR('',#33218,10.);
#9370=VECTOR('',#33219,10.);
#9371=VECTOR('',#33222,10.);
#9372=VECTOR('',#33223,10.);
#9373=VECTOR('',#33224,10.);
#9374=VECTOR('',#33227,10.);
#9375=VECTOR('',#33228,10.);
#9376=VECTOR('',#33229,10.);
#9377=VECTOR('',#33232,10.);
#9378=VECTOR('',#33233,10.);
#9379=VECTOR('',#33234,10.);
#9380=VECTOR('',#33237,9.99999999999999);
#9381=VECTOR('',#33238,9.99999999999999);
#9382=VECTOR('',#33239,10.);
#9383=VECTOR('',#33242,10.);
#9384=VECTOR('',#33243,10.);
#9385=VECTOR('',#33244,10.);
#9386=VECTOR('',#33247,9.99999999999999);
#9387=VECTOR('',#33248,9.99999999999999);
#9388=VECTOR('',#33249,10.);
#9389=VECTOR('',#33252,10.);
#9390=VECTOR('',#33253,10.);
#9391=VECTOR('',#33254,10.);
#9392=VECTOR('',#33257,9.99999999999999);
#9393=VECTOR('',#33258,9.99999999999999);
#9394=VECTOR('',#33259,10.);
#9395=VECTOR('',#33262,10.);
#9396=VECTOR('',#33263,10.);
#9397=VECTOR('',#33264,10.);
#9398=VECTOR('',#33267,10.);
#9399=VECTOR('',#33268,10.);
#9400=VECTOR('',#33269,10.);
#9401=VECTOR('',#33272,10.);
#9402=VECTOR('',#33273,10.);
#9403=VECTOR('',#33274,10.);
#9404=VECTOR('',#33277,10.);
#9405=VECTOR('',#33278,10.);
#9406=VECTOR('',#33279,10.);
#9407=VECTOR('',#33282,10.);
#9408=VECTOR('',#33283,10.);
#9409=VECTOR('',#33284,10.);
#9410=VECTOR('',#33287,10.);
#9411=VECTOR('',#33288,10.);
#9412=VECTOR('',#33289,10.);
#9413=VECTOR('',#33292,10.);
#9414=VECTOR('',#33293,10.);
#9415=VECTOR('',#33294,10.);
#9416=VECTOR('',#33297,10.);
#9417=VECTOR('',#33298,10.);
#9418=VECTOR('',#33299,10.);
#9419=VECTOR('',#33302,10.);
#9420=VECTOR('',#33303,10.);
#9421=VECTOR('',#33304,10.);
#9422=VECTOR('',#33307,10.);
#9423=VECTOR('',#33308,10.);
#9424=VECTOR('',#33309,10.);
#9425=VECTOR('',#33312,10.);
#9426=VECTOR('',#33313,10.);
#9427=VECTOR('',#33314,10.);
#9428=VECTOR('',#33317,10.);
#9429=VECTOR('',#33318,10.);
#9430=VECTOR('',#33319,10.);
#9431=VECTOR('',#33322,10.);
#9432=VECTOR('',#33323,10.);
#9433=VECTOR('',#33324,10.);
#9434=VECTOR('',#33327,10.);
#9435=VECTOR('',#33328,10.);
#9436=VECTOR('',#33329,10.);
#9437=VECTOR('',#33332,10.);
#9438=VECTOR('',#33333,10.);
#9439=VECTOR('',#33334,10.);
#9440=VECTOR('',#33337,10.);
#9441=VECTOR('',#33338,10.);
#9442=VECTOR('',#33339,10.);
#9443=VECTOR('',#33342,10.);
#9444=VECTOR('',#33343,10.);
#9445=VECTOR('',#33344,10.);
#9446=VECTOR('',#33347,10.);
#9447=VECTOR('',#33348,10.);
#9448=VECTOR('',#33349,10.);
#9449=VECTOR('',#33352,10.);
#9450=VECTOR('',#33353,10.);
#9451=VECTOR('',#33354,10.);
#9452=VECTOR('',#33357,10.);
#9453=VECTOR('',#33358,10.);
#9454=VECTOR('',#33359,10.);
#9455=VECTOR('',#33362,10.);
#9456=VECTOR('',#33363,10.);
#9457=VECTOR('',#33364,10.);
#9458=VECTOR('',#33367,10.);
#9459=VECTOR('',#33368,10.);
#9460=VECTOR('',#33369,10.);
#9461=VECTOR('',#33372,10.);
#9462=VECTOR('',#33373,10.);
#9463=VECTOR('',#33374,10.);
#9464=VECTOR('',#33377,10.);
#9465=VECTOR('',#33378,10.);
#9466=VECTOR('',#33379,10.);
#9467=VECTOR('',#33382,10.);
#9468=VECTOR('',#33383,10.);
#9469=VECTOR('',#33384,10.);
#9470=VECTOR('',#33387,10.);
#9471=VECTOR('',#33388,10.);
#9472=VECTOR('',#33389,10.);
#9473=VECTOR('',#33392,10.);
#9474=VECTOR('',#33393,10.);
#9475=VECTOR('',#33394,10.);
#9476=VECTOR('',#33397,10.);
#9477=VECTOR('',#33398,10.);
#9478=VECTOR('',#33399,10.);
#9479=VECTOR('',#33402,10.);
#9480=VECTOR('',#33403,10.);
#9481=VECTOR('',#33404,10.);
#9482=VECTOR('',#33407,10.);
#9483=VECTOR('',#33408,10.);
#9484=VECTOR('',#33409,10.);
#9485=VECTOR('',#33412,10.);
#9486=VECTOR('',#33413,10.);
#9487=VECTOR('',#33414,10.);
#9488=VECTOR('',#33417,10.);
#9489=VECTOR('',#33418,10.);
#9490=VECTOR('',#33419,10.);
#9491=VECTOR('',#33422,10.);
#9492=VECTOR('',#33423,10.);
#9493=VECTOR('',#33424,10.);
#9494=VECTOR('',#33427,10.);
#9495=VECTOR('',#33428,10.);
#9496=VECTOR('',#33429,10.);
#9497=VECTOR('',#33432,10.);
#9498=VECTOR('',#33433,10.);
#9499=VECTOR('',#33434,10.);
#9500=VECTOR('',#33437,10.);
#9501=VECTOR('',#33438,10.);
#10688=CIRCLE('',#28003,4.5625);
#10689=CIRCLE('',#28004,4.7625);
#10690=CIRCLE('',#28007,4.5625);
#10691=CIRCLE('',#28008,4.7625);
#10692=CIRCLE('',#28012,4.7625);
#10693=CIRCLE('',#28015,4.7625);
#10694=CIRCLE('',#28019,4.5625);
#10695=CIRCLE('',#28022,4.5625);
#10696=CIRCLE('',#28025,1.778);
#10697=CIRCLE('',#28026,1.778);
#10698=CIRCLE('',#28028,1.778);
#10699=CIRCLE('',#28029,1.778);
#10700=CIRCLE('',#28031,1.778);
#10701=CIRCLE('',#28032,1.778);
#10702=CIRCLE('',#28034,1.778);
#10703=CIRCLE('',#28035,1.778);
#10704=CIRCLE('',#28037,1.778);
#10705=CIRCLE('',#28038,1.778);
#10706=CIRCLE('',#28040,1.778);
#10707=CIRCLE('',#28041,1.778);
#10708=CIRCLE('',#28043,1.778);
#10709=CIRCLE('',#28044,1.778);
#10710=CIRCLE('',#28046,1.778);
#10711=CIRCLE('',#28047,1.778);
#10712=CIRCLE('',#28049,1.778);
#10713=CIRCLE('',#28050,1.778);
#10714=CIRCLE('',#28052,1.778);
#10715=CIRCLE('',#28053,1.778);
#11979=VERTEX_POINT('',#50942);
#11980=VERTEX_POINT('',#50943);
#11981=VERTEX_POINT('',#50945);
#11982=VERTEX_POINT('',#50947);
#11983=VERTEX_POINT('',#50951);
#11984=VERTEX_POINT('',#50952);
#11985=VERTEX_POINT('',#50957);
#11986=VERTEX_POINT('',#50958);
#11987=VERTEX_POINT('',#50963);
#11988=VERTEX_POINT('',#50964);
#11989=VERTEX_POINT('',#50969);
#11990=VERTEX_POINT('',#50970);
#11991=VERTEX_POINT('',#50975);
#11992=VERTEX_POINT('',#50977);
#11993=VERTEX_POINT('',#50981);
#11994=VERTEX_POINT('',#50985);
#11995=VERTEX_POINT('',#50989);
#11996=VERTEX_POINT('',#50993);
#11997=VERTEX_POINT('',#50997);
#11998=VERTEX_POINT('',#50999);
#11999=VERTEX_POINT('',#51003);
#12000=VERTEX_POINT('',#51007);
#12001=VERTEX_POINT('',#51011);
#12002=VERTEX_POINT('',#51015);
#12003=VERTEX_POINT('',#51019);
#12004=VERTEX_POINT('',#51021);
#12005=VERTEX_POINT('',#51025);
#12006=VERTEX_POINT('',#51027);
#12007=VERTEX_POINT('',#51031);
#12008=VERTEX_POINT('',#51033);
#12009=VERTEX_POINT('',#51037);
#12010=VERTEX_POINT('',#51039);
#12011=VERTEX_POINT('',#51043);
#12012=VERTEX_POINT('',#51045);
#12013=VERTEX_POINT('',#51049);
#12014=VERTEX_POINT('',#51051);
#12015=VERTEX_POINT('',#51055);
#12016=VERTEX_POINT('',#51057);
#12017=VERTEX_POINT('',#51061);
#12018=VERTEX_POINT('',#51063);
#12019=VERTEX_POINT('',#51067);
#12020=VERTEX_POINT('',#51069);
#12021=VERTEX_POINT('',#51073);
#12022=VERTEX_POINT('',#51075);
#12023=VERTEX_POINT('',#51079);
#12024=VERTEX_POINT('',#51081);
#12025=VERTEX_POINT('',#51085);
#12026=VERTEX_POINT('',#51087);
#12027=VERTEX_POINT('',#51091);
#12028=VERTEX_POINT('',#51093);
#12029=VERTEX_POINT('',#51097);
#12030=VERTEX_POINT('',#51099);
#12031=VERTEX_POINT('',#51103);
#12032=VERTEX_POINT('',#51105);
#12033=VERTEX_POINT('',#51109);
#12034=VERTEX_POINT('',#51111);
#12035=VERTEX_POINT('',#51115);
#12036=VERTEX_POINT('',#51117);
#12037=VERTEX_POINT('',#51121);
#12038=VERTEX_POINT('',#51123);
#12039=VERTEX_POINT('',#51127);
#12040=VERTEX_POINT('',#51129);
#12041=VERTEX_POINT('',#51133);
#12042=VERTEX_POINT('',#51135);
#12043=VERTEX_POINT('',#51139);
#12044=VERTEX_POINT('',#51141);
#12045=VERTEX_POINT('',#51145);
#12046=VERTEX_POINT('',#51147);
#12047=VERTEX_POINT('',#51151);
#12048=VERTEX_POINT('',#51153);
#12049=VERTEX_POINT('',#51157);
#12050=VERTEX_POINT('',#51159);
#12051=VERTEX_POINT('',#51163);
#12052=VERTEX_POINT('',#51165);
#12053=VERTEX_POINT('',#51169);
#12054=VERTEX_POINT('',#51171);
#12055=VERTEX_POINT('',#51175);
#12056=VERTEX_POINT('',#51177);
#12057=VERTEX_POINT('',#51181);
#12058=VERTEX_POINT('',#51183);
#12059=VERTEX_POINT('',#51187);
#12060=VERTEX_POINT('',#51189);
#12061=VERTEX_POINT('',#51193);
#12062=VERTEX_POINT('',#51195);
#12063=VERTEX_POINT('',#51199);
#12064=VERTEX_POINT('',#51201);
#12065=VERTEX_POINT('',#51205);
#12066=VERTEX_POINT('',#51207);
#12067=VERTEX_POINT('',#51211);
#12068=VERTEX_POINT('',#51213);
#12069=VERTEX_POINT('',#51217);
#12070=VERTEX_POINT('',#51219);
#12071=VERTEX_POINT('',#51223);
#12072=VERTEX_POINT('',#51225);
#12073=VERTEX_POINT('',#51229);
#12074=VERTEX_POINT('',#51231);
#12075=VERTEX_POINT('',#51235);
#12076=VERTEX_POINT('',#51237);
#12077=VERTEX_POINT('',#51241);
#12078=VERTEX_POINT('',#51243);
#12079=VERTEX_POINT('',#51247);
#12080=VERTEX_POINT('',#51249);
#12081=VERTEX_POINT('',#51253);
#12082=VERTEX_POINT('',#51255);
#12083=VERTEX_POINT('',#51259);
#12084=VERTEX_POINT('',#51261);
#12085=VERTEX_POINT('',#51265);
#12086=VERTEX_POINT('',#51267);
#12087=VERTEX_POINT('',#51271);
#12088=VERTEX_POINT('',#51273);
#12089=VERTEX_POINT('',#51277);
#12090=VERTEX_POINT('',#51279);
#12091=VERTEX_POINT('',#51283);
#12092=VERTEX_POINT('',#51285);
#12093=VERTEX_POINT('',#51289);
#12094=VERTEX_POINT('',#51291);
#12095=VERTEX_POINT('',#51295);
#12096=VERTEX_POINT('',#51297);
#12097=VERTEX_POINT('',#51301);
#12098=VERTEX_POINT('',#51303);
#12099=VERTEX_POINT('',#51307);
#12100=VERTEX_POINT('',#51309);
#12101=VERTEX_POINT('',#51313);
#12102=VERTEX_POINT('',#51315);
#12103=VERTEX_POINT('',#51319);
#12104=VERTEX_POINT('',#51321);
#12105=VERTEX_POINT('',#51325);
#12106=VERTEX_POINT('',#51327);
#12107=VERTEX_POINT('',#51331);
#12108=VERTEX_POINT('',#51333);
#12109=VERTEX_POINT('',#51337);
#12110=VERTEX_POINT('',#51339);
#12111=VERTEX_POINT('',#51343);
#12112=VERTEX_POINT('',#51345);
#12113=VERTEX_POINT('',#51349);
#12114=VERTEX_POINT('',#51351);
#12115=VERTEX_POINT('',#51355);
#12116=VERTEX_POINT('',#51357);
#12117=VERTEX_POINT('',#51361);
#12118=VERTEX_POINT('',#51363);
#12119=VERTEX_POINT('',#51367);
#12120=VERTEX_POINT('',#51369);
#12121=VERTEX_POINT('',#51373);
#12122=VERTEX_POINT('',#51375);
#12123=VERTEX_POINT('',#51379);
#12124=VERTEX_POINT('',#51381);
#12125=VERTEX_POINT('',#51385);
#12126=VERTEX_POINT('',#51387);
#12127=VERTEX_POINT('',#51391);
#12128=VERTEX_POINT('',#51393);
#12129=VERTEX_POINT('',#51397);
#12130=VERTEX_POINT('',#51399);
#12131=VERTEX_POINT('',#51403);
#12132=VERTEX_POINT('',#51405);
#12133=VERTEX_POINT('',#51409);
#12134=VERTEX_POINT('',#51411);
#12135=VERTEX_POINT('',#51415);
#12136=VERTEX_POINT('',#51417);
#12137=VERTEX_POINT('',#51421);
#12138=VERTEX_POINT('',#51423);
#12139=VERTEX_POINT('',#51427);
#12140=VERTEX_POINT('',#51429);
#12141=VERTEX_POINT('',#51433);
#12142=VERTEX_POINT('',#51435);
#12143=VERTEX_POINT('',#51439);
#12144=VERTEX_POINT('',#51441);
#12145=VERTEX_POINT('',#51445);
#12146=VERTEX_POINT('',#51447);
#12147=VERTEX_POINT('',#51451);
#12148=VERTEX_POINT('',#51453);
#12149=VERTEX_POINT('',#51457);
#12150=VERTEX_POINT('',#51459);
#12151=VERTEX_POINT('',#51463);
#12152=VERTEX_POINT('',#51465);
#12153=VERTEX_POINT('',#51469);
#12154=VERTEX_POINT('',#51471);
#12155=VERTEX_POINT('',#51475);
#12156=VERTEX_POINT('',#51477);
#12157=VERTEX_POINT('',#51481);
#12158=VERTEX_POINT('',#51483);
#12159=VERTEX_POINT('',#51487);
#12160=VERTEX_POINT('',#51489);
#12161=VERTEX_POINT('',#51493);
#12162=VERTEX_POINT('',#51495);
#12163=VERTEX_POINT('',#51499);
#12164=VERTEX_POINT('',#51501);
#12165=VERTEX_POINT('',#51505);
#12166=VERTEX_POINT('',#51507);
#12167=VERTEX_POINT('',#51511);
#12168=VERTEX_POINT('',#51513);
#12169=VERTEX_POINT('',#51517);
#12170=VERTEX_POINT('',#51519);
#12171=VERTEX_POINT('',#51523);
#12172=VERTEX_POINT('',#51525);
#12173=VERTEX_POINT('',#51529);
#12174=VERTEX_POINT('',#51531);
#12175=VERTEX_POINT('',#51535);
#12176=VERTEX_POINT('',#51537);
#12177=VERTEX_POINT('',#51541);
#12178=VERTEX_POINT('',#51543);
#12179=VERTEX_POINT('',#51547);
#12180=VERTEX_POINT('',#51549);
#12181=VERTEX_POINT('',#51553);
#12182=VERTEX_POINT('',#51555);
#12183=VERTEX_POINT('',#51559);
#12184=VERTEX_POINT('',#51561);
#12185=VERTEX_POINT('',#51565);
#12186=VERTEX_POINT('',#51567);
#12187=VERTEX_POINT('',#51571);
#12188=VERTEX_POINT('',#51573);
#12189=VERTEX_POINT('',#51577);
#12190=VERTEX_POINT('',#51579);
#12191=VERTEX_POINT('',#51583);
#12192=VERTEX_POINT('',#51585);
#12193=VERTEX_POINT('',#51589);
#12194=VERTEX_POINT('',#51591);
#12195=VERTEX_POINT('',#51595);
#12196=VERTEX_POINT('',#51597);
#12197=VERTEX_POINT('',#51601);
#12198=VERTEX_POINT('',#51603);
#12199=VERTEX_POINT('',#51607);
#12200=VERTEX_POINT('',#51609);
#12201=VERTEX_POINT('',#51613);
#12202=VERTEX_POINT('',#51615);
#12203=VERTEX_POINT('',#51619);
#12204=VERTEX_POINT('',#51621);
#12205=VERTEX_POINT('',#51625);
#12206=VERTEX_POINT('',#51627);
#12207=VERTEX_POINT('',#51631);
#12208=VERTEX_POINT('',#51633);
#12209=VERTEX_POINT('',#51637);
#12210=VERTEX_POINT('',#51639);
#12211=VERTEX_POINT('',#51643);
#12212=VERTEX_POINT('',#51645);
#12213=VERTEX_POINT('',#51649);
#12214=VERTEX_POINT('',#51651);
#12215=VERTEX_POINT('',#51655);
#12216=VERTEX_POINT('',#51657);
#12217=VERTEX_POINT('',#51661);
#12218=VERTEX_POINT('',#51663);
#12219=VERTEX_POINT('',#51667);
#12220=VERTEX_POINT('',#51669);
#12221=VERTEX_POINT('',#51673);
#12222=VERTEX_POINT('',#51675);
#12223=VERTEX_POINT('',#51679);
#12224=VERTEX_POINT('',#51681);
#12225=VERTEX_POINT('',#51685);
#12226=VERTEX_POINT('',#51687);
#12227=VERTEX_POINT('',#51691);
#12228=VERTEX_POINT('',#51693);
#12229=VERTEX_POINT('',#51697);
#12230=VERTEX_POINT('',#51699);
#12231=VERTEX_POINT('',#51703);
#12232=VERTEX_POINT('',#51705);
#12233=VERTEX_POINT('',#51709);
#12234=VERTEX_POINT('',#51711);
#12235=VERTEX_POINT('',#51715);
#12236=VERTEX_POINT('',#51717);
#12237=VERTEX_POINT('',#51721);
#12238=VERTEX_POINT('',#51723);
#12239=VERTEX_POINT('',#51727);
#12240=VERTEX_POINT('',#51729);
#12241=VERTEX_POINT('',#51733);
#12242=VERTEX_POINT('',#51735);
#12243=VERTEX_POINT('',#51739);
#12244=VERTEX_POINT('',#51741);
#12245=VERTEX_POINT('',#51745);
#12246=VERTEX_POINT('',#51747);
#12247=VERTEX_POINT('',#51751);
#12248=VERTEX_POINT('',#51753);
#12249=VERTEX_POINT('',#51757);
#12250=VERTEX_POINT('',#51759);
#12251=VERTEX_POINT('',#51763);
#12252=VERTEX_POINT('',#51765);
#12253=VERTEX_POINT('',#51769);
#12254=VERTEX_POINT('',#51771);
#12255=VERTEX_POINT('',#51775);
#12256=VERTEX_POINT('',#51777);
#12257=VERTEX_POINT('',#51781);
#12258=VERTEX_POINT('',#51783);
#12259=VERTEX_POINT('',#51787);
#12260=VERTEX_POINT('',#51789);
#12261=VERTEX_POINT('',#51793);
#12262=VERTEX_POINT('',#51795);
#12263=VERTEX_POINT('',#51799);
#12264=VERTEX_POINT('',#51801);
#12265=VERTEX_POINT('',#51805);
#12266=VERTEX_POINT('',#51807);
#12267=VERTEX_POINT('',#51811);
#12268=VERTEX_POINT('',#51813);
#12269=VERTEX_POINT('',#51817);
#12270=VERTEX_POINT('',#51819);
#12271=VERTEX_POINT('',#51823);
#12272=VERTEX_POINT('',#51825);
#12273=VERTEX_POINT('',#51829);
#12274=VERTEX_POINT('',#51831);
#12275=VERTEX_POINT('',#51835);
#12276=VERTEX_POINT('',#51837);
#12277=VERTEX_POINT('',#51841);
#12278=VERTEX_POINT('',#51843);
#12279=VERTEX_POINT('',#51847);
#12280=VERTEX_POINT('',#51849);
#12281=VERTEX_POINT('',#51853);
#12282=VERTEX_POINT('',#51855);
#12283=VERTEX_POINT('',#51859);
#12284=VERTEX_POINT('',#51861);
#12285=VERTEX_POINT('',#51865);
#12286=VERTEX_POINT('',#51867);
#12287=VERTEX_POINT('',#51871);
#12288=VERTEX_POINT('',#51873);
#12289=VERTEX_POINT('',#51877);
#12290=VERTEX_POINT('',#51879);
#12291=VERTEX_POINT('',#51883);
#12292=VERTEX_POINT('',#51885);
#12293=VERTEX_POINT('',#51889);
#12294=VERTEX_POINT('',#51891);
#12295=VERTEX_POINT('',#51895);
#12296=VERTEX_POINT('',#51897);
#12297=VERTEX_POINT('',#51901);
#12298=VERTEX_POINT('',#51903);
#12299=VERTEX_POINT('',#51907);
#12300=VERTEX_POINT('',#51909);
#12301=VERTEX_POINT('',#51913);
#12302=VERTEX_POINT('',#51915);
#12303=VERTEX_POINT('',#51919);
#12304=VERTEX_POINT('',#51921);
#12305=VERTEX_POINT('',#51925);
#12306=VERTEX_POINT('',#51927);
#12307=VERTEX_POINT('',#51931);
#12308=VERTEX_POINT('',#51933);
#12309=VERTEX_POINT('',#51937);
#12310=VERTEX_POINT('',#51939);
#12311=VERTEX_POINT('',#51943);
#12312=VERTEX_POINT('',#51945);
#12313=VERTEX_POINT('',#51949);
#12314=VERTEX_POINT('',#51951);
#12315=VERTEX_POINT('',#51955);
#12316=VERTEX_POINT('',#51957);
#12317=VERTEX_POINT('',#51961);
#12318=VERTEX_POINT('',#51963);
#12319=VERTEX_POINT('',#51967);
#12320=VERTEX_POINT('',#51969);
#12321=VERTEX_POINT('',#51973);
#12322=VERTEX_POINT('',#51975);
#12323=VERTEX_POINT('',#51979);
#12324=VERTEX_POINT('',#51981);
#12325=VERTEX_POINT('',#51985);
#12326=VERTEX_POINT('',#51987);
#12327=VERTEX_POINT('',#51991);
#12328=VERTEX_POINT('',#51993);
#12329=VERTEX_POINT('',#51997);
#12330=VERTEX_POINT('',#51999);
#12331=VERTEX_POINT('',#52003);
#12332=VERTEX_POINT('',#52005);
#12333=VERTEX_POINT('',#52009);
#12334=VERTEX_POINT('',#52011);
#12335=VERTEX_POINT('',#52015);
#12336=VERTEX_POINT('',#52017);
#12337=VERTEX_POINT('',#52021);
#12338=VERTEX_POINT('',#52023);
#12339=VERTEX_POINT('',#52027);
#12340=VERTEX_POINT('',#52029);
#12341=VERTEX_POINT('',#52033);
#12342=VERTEX_POINT('',#52035);
#12343=VERTEX_POINT('',#52039);
#12344=VERTEX_POINT('',#52041);
#12345=VERTEX_POINT('',#52045);
#12346=VERTEX_POINT('',#52047);
#12347=VERTEX_POINT('',#52051);
#12348=VERTEX_POINT('',#52053);
#12349=VERTEX_POINT('',#52057);
#12350=VERTEX_POINT('',#52059);
#12351=VERTEX_POINT('',#52063);
#12352=VERTEX_POINT('',#52065);
#12353=VERTEX_POINT('',#52069);
#12354=VERTEX_POINT('',#52071);
#12355=VERTEX_POINT('',#52075);
#12356=VERTEX_POINT('',#52077);
#12357=VERTEX_POINT('',#52081);
#12358=VERTEX_POINT('',#52083);
#12359=VERTEX_POINT('',#52087);
#12360=VERTEX_POINT('',#52089);
#12361=VERTEX_POINT('',#52093);
#12362=VERTEX_POINT('',#52095);
#12363=VERTEX_POINT('',#52099);
#12364=VERTEX_POINT('',#52101);
#12365=VERTEX_POINT('',#52105);
#12366=VERTEX_POINT('',#52107);
#12367=VERTEX_POINT('',#52111);
#12368=VERTEX_POINT('',#52113);
#12369=VERTEX_POINT('',#52117);
#12370=VERTEX_POINT('',#52119);
#12371=VERTEX_POINT('',#52123);
#12372=VERTEX_POINT('',#52125);
#12373=VERTEX_POINT('',#52129);
#12374=VERTEX_POINT('',#52131);
#12375=VERTEX_POINT('',#52135);
#12376=VERTEX_POINT('',#52137);
#12377=VERTEX_POINT('',#52141);
#12378=VERTEX_POINT('',#52143);
#12379=VERTEX_POINT('',#52147);
#12380=VERTEX_POINT('',#52149);
#12381=VERTEX_POINT('',#52153);
#12382=VERTEX_POINT('',#52155);
#12383=VERTEX_POINT('',#52159);
#12384=VERTEX_POINT('',#52161);
#12385=VERTEX_POINT('',#52165);
#12386=VERTEX_POINT('',#52167);
#12387=VERTEX_POINT('',#52171);
#12388=VERTEX_POINT('',#52173);
#12389=VERTEX_POINT('',#52177);
#12390=VERTEX_POINT('',#52179);
#12391=VERTEX_POINT('',#52183);
#12392=VERTEX_POINT('',#52185);
#12393=VERTEX_POINT('',#52189);
#12394=VERTEX_POINT('',#52191);
#12395=VERTEX_POINT('',#52195);
#12396=VERTEX_POINT('',#52197);
#12397=VERTEX_POINT('',#52201);
#12398=VERTEX_POINT('',#52203);
#12399=VERTEX_POINT('',#52207);
#12400=VERTEX_POINT('',#52209);
#12401=VERTEX_POINT('',#52213);
#12402=VERTEX_POINT('',#52215);
#12403=VERTEX_POINT('',#52219);
#12404=VERTEX_POINT('',#52221);
#12405=VERTEX_POINT('',#52225);
#12406=VERTEX_POINT('',#52227);
#12407=VERTEX_POINT('',#52231);
#12408=VERTEX_POINT('',#52233);
#12409=VERTEX_POINT('',#52237);
#12410=VERTEX_POINT('',#52239);
#12411=VERTEX_POINT('',#52243);
#12412=VERTEX_POINT('',#52245);
#12413=VERTEX_POINT('',#52249);
#12414=VERTEX_POINT('',#52251);
#12415=VERTEX_POINT('',#52255);
#12416=VERTEX_POINT('',#52257);
#12417=VERTEX_POINT('',#52261);
#12418=VERTEX_POINT('',#52263);
#12419=VERTEX_POINT('',#52267);
#12420=VERTEX_POINT('',#52269);
#12421=VERTEX_POINT('',#52273);
#12422=VERTEX_POINT('',#52275);
#12423=VERTEX_POINT('',#52279);
#12424=VERTEX_POINT('',#52281);
#12425=VERTEX_POINT('',#52285);
#12426=VERTEX_POINT('',#52287);
#12427=VERTEX_POINT('',#52291);
#12428=VERTEX_POINT('',#52293);
#12429=VERTEX_POINT('',#52297);
#12430=VERTEX_POINT('',#52299);
#12431=VERTEX_POINT('',#52303);
#12432=VERTEX_POINT('',#52305);
#12433=VERTEX_POINT('',#52309);
#12434=VERTEX_POINT('',#52311);
#12435=VERTEX_POINT('',#52315);
#12436=VERTEX_POINT('',#52317);
#12437=VERTEX_POINT('',#52321);
#12438=VERTEX_POINT('',#52323);
#12439=VERTEX_POINT('',#52327);
#12440=VERTEX_POINT('',#52329);
#12441=VERTEX_POINT('',#52333);
#12442=VERTEX_POINT('',#52335);
#12443=VERTEX_POINT('',#52339);
#12444=VERTEX_POINT('',#52341);
#12445=VERTEX_POINT('',#52345);
#12446=VERTEX_POINT('',#52347);
#12447=VERTEX_POINT('',#52351);
#12448=VERTEX_POINT('',#52353);
#12449=VERTEX_POINT('',#52357);
#12450=VERTEX_POINT('',#52359);
#12451=VERTEX_POINT('',#52363);
#12452=VERTEX_POINT('',#52365);
#12453=VERTEX_POINT('',#52369);
#12454=VERTEX_POINT('',#52371);
#12455=VERTEX_POINT('',#52375);
#12456=VERTEX_POINT('',#52377);
#12457=VERTEX_POINT('',#52381);
#12458=VERTEX_POINT('',#52383);
#12459=VERTEX_POINT('',#52387);
#12460=VERTEX_POINT('',#52389);
#12461=VERTEX_POINT('',#52393);
#12462=VERTEX_POINT('',#52395);
#12463=VERTEX_POINT('',#52399);
#12464=VERTEX_POINT('',#52401);
#12465=VERTEX_POINT('',#52405);
#12466=VERTEX_POINT('',#52407);
#12467=VERTEX_POINT('',#52411);
#12468=VERTEX_POINT('',#52413);
#12469=VERTEX_POINT('',#52417);
#12470=VERTEX_POINT('',#52419);
#12471=VERTEX_POINT('',#52423);
#12472=VERTEX_POINT('',#52425);
#12473=VERTEX_POINT('',#52429);
#12474=VERTEX_POINT('',#52431);
#12475=VERTEX_POINT('',#52435);
#12476=VERTEX_POINT('',#52437);
#12477=VERTEX_POINT('',#52441);
#12478=VERTEX_POINT('',#52443);
#12479=VERTEX_POINT('',#52447);
#12480=VERTEX_POINT('',#52449);
#12481=VERTEX_POINT('',#52453);
#12482=VERTEX_POINT('',#52455);
#12483=VERTEX_POINT('',#52459);
#12484=VERTEX_POINT('',#52461);
#12485=VERTEX_POINT('',#52465);
#12486=VERTEX_POINT('',#52467);
#12487=VERTEX_POINT('',#52471);
#12488=VERTEX_POINT('',#52473);
#12489=VERTEX_POINT('',#52477);
#12490=VERTEX_POINT('',#52479);
#12491=VERTEX_POINT('',#52483);
#12492=VERTEX_POINT('',#52485);
#12493=VERTEX_POINT('',#52489);
#12494=VERTEX_POINT('',#52491);
#12495=VERTEX_POINT('',#52495);
#12496=VERTEX_POINT('',#52497);
#12497=VERTEX_POINT('',#52501);
#12498=VERTEX_POINT('',#52503);
#12499=VERTEX_POINT('',#52507);
#12500=VERTEX_POINT('',#52509);
#12501=VERTEX_POINT('',#52513);
#12502=VERTEX_POINT('',#52515);
#12503=VERTEX_POINT('',#52519);
#12504=VERTEX_POINT('',#52521);
#12505=VERTEX_POINT('',#52525);
#12506=VERTEX_POINT('',#52527);
#12507=VERTEX_POINT('',#52531);
#12508=VERTEX_POINT('',#52533);
#12509=VERTEX_POINT('',#52537);
#12510=VERTEX_POINT('',#52539);
#12511=VERTEX_POINT('',#52543);
#12512=VERTEX_POINT('',#52545);
#12513=VERTEX_POINT('',#52549);
#12514=VERTEX_POINT('',#52551);
#12515=VERTEX_POINT('',#52555);
#12516=VERTEX_POINT('',#52557);
#12517=VERTEX_POINT('',#52561);
#12518=VERTEX_POINT('',#52563);
#12519=VERTEX_POINT('',#52567);
#12520=VERTEX_POINT('',#52569);
#12521=VERTEX_POINT('',#52573);
#12522=VERTEX_POINT('',#52575);
#12523=VERTEX_POINT('',#52579);
#12524=VERTEX_POINT('',#52581);
#12525=VERTEX_POINT('',#52585);
#12526=VERTEX_POINT('',#52587);
#12527=VERTEX_POINT('',#52591);
#12528=VERTEX_POINT('',#52593);
#12529=VERTEX_POINT('',#52597);
#12530=VERTEX_POINT('',#52599);
#12531=VERTEX_POINT('',#52603);
#12532=VERTEX_POINT('',#52605);
#12533=VERTEX_POINT('',#52609);
#12534=VERTEX_POINT('',#52611);
#12535=VERTEX_POINT('',#52615);
#12536=VERTEX_POINT('',#52617);
#12537=VERTEX_POINT('',#52621);
#12538=VERTEX_POINT('',#52623);
#12539=VERTEX_POINT('',#52627);
#12540=VERTEX_POINT('',#52629);
#12541=VERTEX_POINT('',#52633);
#12542=VERTEX_POINT('',#52635);
#12543=VERTEX_POINT('',#52639);
#12544=VERTEX_POINT('',#52641);
#12545=VERTEX_POINT('',#52645);
#12546=VERTEX_POINT('',#52647);
#12547=VERTEX_POINT('',#52651);
#12548=VERTEX_POINT('',#52653);
#12549=VERTEX_POINT('',#52657);
#12550=VERTEX_POINT('',#52659);
#12551=VERTEX_POINT('',#52663);
#12552=VERTEX_POINT('',#52665);
#12553=VERTEX_POINT('',#52669);
#12554=VERTEX_POINT('',#52671);
#12555=VERTEX_POINT('',#52675);
#12556=VERTEX_POINT('',#52677);
#12557=VERTEX_POINT('',#52681);
#12558=VERTEX_POINT('',#52683);
#12559=VERTEX_POINT('',#52687);
#12560=VERTEX_POINT('',#52689);
#12561=VERTEX_POINT('',#52693);
#12562=VERTEX_POINT('',#52695);
#12563=VERTEX_POINT('',#52699);
#12564=VERTEX_POINT('',#52701);
#12565=VERTEX_POINT('',#52705);
#12566=VERTEX_POINT('',#52707);
#12567=VERTEX_POINT('',#52711);
#12568=VERTEX_POINT('',#52713);
#12569=VERTEX_POINT('',#52717);
#12570=VERTEX_POINT('',#52719);
#12571=VERTEX_POINT('',#52723);
#12572=VERTEX_POINT('',#52725);
#12573=VERTEX_POINT('',#52729);
#12574=VERTEX_POINT('',#52731);
#12575=VERTEX_POINT('',#52735);
#12576=VERTEX_POINT('',#52737);
#12577=VERTEX_POINT('',#52741);
#12578=VERTEX_POINT('',#52743);
#15098=EDGE_CURVE('',#11979,#11980,#6115,.F.);
#15099=EDGE_CURVE('',#11980,#11981,#6116,.T.);
#15100=EDGE_CURVE('',#11981,#11982,#6117,.T.);
#15101=EDGE_CURVE('',#11982,#11979,#6118,.T.);
#15102=EDGE_CURVE('',#11983,#11984,#6119,.T.);
#15103=EDGE_CURVE('',#11984,#11982,#10688,.T.);
#15104=EDGE_CURVE('',#11981,#11983,#10689,.T.);
#15105=EDGE_CURVE('',#11985,#11986,#6120,.T.);
#15106=EDGE_CURVE('',#11986,#11984,#6121,.T.);
#15107=EDGE_CURVE('',#11983,#11985,#6122,.T.);
#15108=EDGE_CURVE('',#11987,#11988,#6123,.T.);
#15109=EDGE_CURVE('',#11988,#11986,#10690,.T.);
#15110=EDGE_CURVE('',#11985,#11987,#10691,.T.);
#15111=EDGE_CURVE('',#11989,#11990,#6124,.F.);
#15112=EDGE_CURVE('',#11990,#11988,#6125,.T.);
#15113=EDGE_CURVE('',#11987,#11989,#6126,.T.);
#15114=EDGE_CURVE('',#11991,#11987,#6127,.T.);
#15115=EDGE_CURVE('',#11992,#11991,#6128,.T.);
#15116=EDGE_CURVE('',#11992,#11989,#6129,.T.);
#15117=EDGE_CURVE('',#11993,#11985,#6130,.T.);
#15118=EDGE_CURVE('',#11991,#11993,#10692,.T.);
#15119=EDGE_CURVE('',#11994,#11983,#6131,.T.);
#15120=EDGE_CURVE('',#11993,#11994,#6132,.T.);
#15121=EDGE_CURVE('',#11995,#11981,#6133,.T.);
#15122=EDGE_CURVE('',#11994,#11995,#10693,.T.);
#15123=EDGE_CURVE('',#11996,#11980,#6134,.T.);
#15124=EDGE_CURVE('',#11995,#11996,#6135,.T.);
#15125=EDGE_CURVE('',#11997,#11992,#6136,.F.);
#15126=EDGE_CURVE('',#11991,#11998,#6137,.T.);
#15127=EDGE_CURVE('',#11998,#11997,#6138,.T.);
#15128=EDGE_CURVE('',#11993,#11999,#6139,.T.);
#15129=EDGE_CURVE('',#11999,#11998,#10694,.T.);
#15130=EDGE_CURVE('',#11994,#12000,#6140,.T.);
#15131=EDGE_CURVE('',#12000,#11999,#6141,.T.);
#15132=EDGE_CURVE('',#11995,#12001,#6142,.T.);
#15133=EDGE_CURVE('',#12001,#12000,#10695,.T.);
#15134=EDGE_CURVE('',#11996,#12002,#6143,.F.);
#15135=EDGE_CURVE('',#12002,#12001,#6144,.T.);
#15136=EDGE_CURVE('',#12003,#12003,#10696,.T.);
#15137=EDGE_CURVE('',#12003,#12004,#6145,.T.);
#15138=EDGE_CURVE('',#12004,#12004,#10697,.T.);
#15139=EDGE_CURVE('',#12005,#12005,#10698,.T.);
#15140=EDGE_CURVE('',#12005,#12006,#6146,.T.);
#15141=EDGE_CURVE('',#12006,#12006,#10699,.T.);
#15142=EDGE_CURVE('',#12007,#12007,#10700,.T.);
#15143=EDGE_CURVE('',#12007,#12008,#6147,.T.);
#15144=EDGE_CURVE('',#12008,#12008,#10701,.T.);
#15145=EDGE_CURVE('',#12009,#12009,#10702,.T.);
#15146=EDGE_CURVE('',#12009,#12010,#6148,.T.);
#15147=EDGE_CURVE('',#12010,#12010,#10703,.T.);
#15148=EDGE_CURVE('',#12011,#12011,#10704,.T.);
#15149=EDGE_CURVE('',#12011,#12012,#6149,.T.);
#15150=EDGE_CURVE('',#12012,#12012,#10705,.T.);
#15151=EDGE_CURVE('',#12013,#12013,#10706,.T.);
#15152=EDGE_CURVE('',#12013,#12014,#6150,.T.);
#15153=EDGE_CURVE('',#12014,#12014,#10707,.T.);
#15154=EDGE_CURVE('',#12015,#12015,#10708,.T.);
#15155=EDGE_CURVE('',#12015,#12016,#6151,.T.);
#15156=EDGE_CURVE('',#12016,#12016,#10709,.T.);
#15157=EDGE_CURVE('',#12017,#12017,#10710,.T.);
#15158=EDGE_CURVE('',#12017,#12018,#6152,.T.);
#15159=EDGE_CURVE('',#12018,#12018,#10711,.T.);
#15160=EDGE_CURVE('',#12019,#12019,#10712,.T.);
#15161=EDGE_CURVE('',#12019,#12020,#6153,.T.);
#15162=EDGE_CURVE('',#12020,#12020,#10713,.T.);
#15163=EDGE_CURVE('',#12021,#12021,#10714,.T.);
#15164=EDGE_CURVE('',#12021,#12022,#6154,.T.);
#15165=EDGE_CURVE('',#12022,#12022,#10715,.T.);
#15166=EDGE_CURVE('',#12002,#12023,#6155,.T.);
#15167=EDGE_CURVE('',#12024,#11979,#6156,.T.);
#15168=EDGE_CURVE('',#12023,#12024,#6157,.T.);
#15169=EDGE_CURVE('',#12023,#12025,#6158,.T.);
#15170=EDGE_CURVE('',#12026,#12024,#6159,.T.);
#15171=EDGE_CURVE('',#12025,#12026,#6160,.T.);
#15172=EDGE_CURVE('',#12025,#12027,#6161,.T.);
#15173=EDGE_CURVE('',#12028,#12026,#6162,.T.);
#15174=EDGE_CURVE('',#12027,#12028,#6163,.T.);
#15175=EDGE_CURVE('',#12027,#12029,#6164,.T.);
#15176=EDGE_CURVE('',#12030,#12028,#6165,.T.);
#15177=EDGE_CURVE('',#12029,#12030,#6166,.T.);
#15178=EDGE_CURVE('',#12029,#12031,#6167,.T.);
#15179=EDGE_CURVE('',#12032,#12030,#6168,.T.);
#15180=EDGE_CURVE('',#12031,#12032,#6169,.T.);
#15181=EDGE_CURVE('',#12031,#12033,#6170,.T.);
#15182=EDGE_CURVE('',#12034,#12032,#6171,.T.);
#15183=EDGE_CURVE('',#12033,#12034,#6172,.T.);
#15184=EDGE_CURVE('',#12033,#12035,#6173,.T.);
#15185=EDGE_CURVE('',#12036,#12034,#6174,.T.);
#15186=EDGE_CURVE('',#12035,#12036,#6175,.T.);
#15187=EDGE_CURVE('',#12035,#12037,#6176,.T.);
#15188=EDGE_CURVE('',#12038,#12036,#6177,.T.);
#15189=EDGE_CURVE('',#12037,#12038,#6178,.T.);
#15190=EDGE_CURVE('',#12037,#12039,#6179,.T.);
#15191=EDGE_CURVE('',#12040,#12038,#6180,.T.);
#15192=EDGE_CURVE('',#12039,#12040,#6181,.T.);
#15193=EDGE_CURVE('',#12039,#12041,#6182,.T.);
#15194=EDGE_CURVE('',#12042,#12040,#6183,.T.);
#15195=EDGE_CURVE('',#12041,#12042,#6184,.T.);
#15196=EDGE_CURVE('',#12041,#12043,#6185,.T.);
#15197=EDGE_CURVE('',#12044,#12042,#6186,.T.);
#15198=EDGE_CURVE('',#12043,#12044,#6187,.T.);
#15199=EDGE_CURVE('',#12043,#12045,#6188,.T.);
#15200=EDGE_CURVE('',#12046,#12044,#6189,.T.);
#15201=EDGE_CURVE('',#12045,#12046,#6190,.T.);
#15202=EDGE_CURVE('',#12045,#12047,#6191,.T.);
#15203=EDGE_CURVE('',#12048,#12046,#6192,.T.);
#15204=EDGE_CURVE('',#12047,#12048,#6193,.T.);
#15205=EDGE_CURVE('',#12047,#12049,#6194,.T.);
#15206=EDGE_CURVE('',#12050,#12048,#6195,.T.);
#15207=EDGE_CURVE('',#12049,#12050,#6196,.T.);
#15208=EDGE_CURVE('',#12049,#12051,#6197,.T.);
#15209=EDGE_CURVE('',#12052,#12050,#6198,.T.);
#15210=EDGE_CURVE('',#12051,#12052,#6199,.T.);
#15211=EDGE_CURVE('',#12051,#12053,#6200,.T.);
#15212=EDGE_CURVE('',#12054,#12052,#6201,.T.);
#15213=EDGE_CURVE('',#12053,#12054,#6202,.T.);
#15214=EDGE_CURVE('',#12053,#12055,#6203,.T.);
#15215=EDGE_CURVE('',#12056,#12054,#6204,.T.);
#15216=EDGE_CURVE('',#12055,#12056,#6205,.T.);
#15217=EDGE_CURVE('',#12055,#12057,#6206,.T.);
#15218=EDGE_CURVE('',#12058,#12056,#6207,.T.);
#15219=EDGE_CURVE('',#12057,#12058,#6208,.T.);
#15220=EDGE_CURVE('',#12057,#12059,#6209,.T.);
#15221=EDGE_CURVE('',#12060,#12058,#6210,.T.);
#15222=EDGE_CURVE('',#12059,#12060,#6211,.T.);
#15223=EDGE_CURVE('',#12059,#12061,#6212,.T.);
#15224=EDGE_CURVE('',#12062,#12060,#6213,.T.);
#15225=EDGE_CURVE('',#12061,#12062,#6214,.T.);
#15226=EDGE_CURVE('',#12061,#12063,#6215,.T.);
#15227=EDGE_CURVE('',#12064,#12062,#6216,.T.);
#15228=EDGE_CURVE('',#12063,#12064,#6217,.T.);
#15229=EDGE_CURVE('',#12063,#12065,#6218,.T.);
#15230=EDGE_CURVE('',#12066,#12064,#6219,.T.);
#15231=EDGE_CURVE('',#12065,#12066,#6220,.T.);
#15232=EDGE_CURVE('',#12065,#12067,#6221,.T.);
#15233=EDGE_CURVE('',#12068,#12066,#6222,.T.);
#15234=EDGE_CURVE('',#12067,#12068,#6223,.T.);
#15235=EDGE_CURVE('',#12067,#12069,#6224,.T.);
#15236=EDGE_CURVE('',#12070,#12068,#6225,.T.);
#15237=EDGE_CURVE('',#12069,#12070,#6226,.T.);
#15238=EDGE_CURVE('',#12069,#12071,#6227,.T.);
#15239=EDGE_CURVE('',#12072,#12070,#6228,.T.);
#15240=EDGE_CURVE('',#12071,#12072,#6229,.T.);
#15241=EDGE_CURVE('',#12071,#12073,#6230,.T.);
#15242=EDGE_CURVE('',#12074,#12072,#6231,.T.);
#15243=EDGE_CURVE('',#12073,#12074,#6232,.T.);
#15244=EDGE_CURVE('',#12073,#12075,#6233,.T.);
#15245=EDGE_CURVE('',#12076,#12074,#6234,.T.);
#15246=EDGE_CURVE('',#12075,#12076,#6235,.T.);
#15247=EDGE_CURVE('',#12075,#12077,#6236,.T.);
#15248=EDGE_CURVE('',#12078,#12076,#6237,.T.);
#15249=EDGE_CURVE('',#12077,#12078,#6238,.T.);
#15250=EDGE_CURVE('',#12077,#12079,#6239,.T.);
#15251=EDGE_CURVE('',#12080,#12078,#6240,.T.);
#15252=EDGE_CURVE('',#12079,#12080,#6241,.T.);
#15253=EDGE_CURVE('',#12079,#12081,#6242,.T.);
#15254=EDGE_CURVE('',#12082,#12080,#6243,.T.);
#15255=EDGE_CURVE('',#12081,#12082,#6244,.T.);
#15256=EDGE_CURVE('',#12081,#12083,#6245,.T.);
#15257=EDGE_CURVE('',#12084,#12082,#6246,.T.);
#15258=EDGE_CURVE('',#12083,#12084,#6247,.T.);
#15259=EDGE_CURVE('',#12083,#12085,#6248,.T.);
#15260=EDGE_CURVE('',#12086,#12084,#6249,.T.);
#15261=EDGE_CURVE('',#12085,#12086,#6250,.T.);
#15262=EDGE_CURVE('',#12085,#12087,#6251,.T.);
#15263=EDGE_CURVE('',#12088,#12086,#6252,.T.);
#15264=EDGE_CURVE('',#12087,#12088,#6253,.T.);
#15265=EDGE_CURVE('',#12087,#12089,#6254,.T.);
#15266=EDGE_CURVE('',#12090,#12088,#6255,.T.);
#15267=EDGE_CURVE('',#12089,#12090,#6256,.T.);
#15268=EDGE_CURVE('',#12089,#12091,#6257,.T.);
#15269=EDGE_CURVE('',#12092,#12090,#6258,.T.);
#15270=EDGE_CURVE('',#12091,#12092,#6259,.T.);
#15271=EDGE_CURVE('',#12091,#12093,#6260,.T.);
#15272=EDGE_CURVE('',#12094,#12092,#6261,.T.);
#15273=EDGE_CURVE('',#12093,#12094,#6262,.T.);
#15274=EDGE_CURVE('',#12093,#12095,#6263,.T.);
#15275=EDGE_CURVE('',#12096,#12094,#6264,.T.);
#15276=EDGE_CURVE('',#12095,#12096,#6265,.T.);
#15277=EDGE_CURVE('',#12095,#12097,#6266,.T.);
#15278=EDGE_CURVE('',#12098,#12096,#6267,.T.);
#15279=EDGE_CURVE('',#12097,#12098,#6268,.T.);
#15280=EDGE_CURVE('',#12097,#12099,#6269,.T.);
#15281=EDGE_CURVE('',#12100,#12098,#6270,.T.);
#15282=EDGE_CURVE('',#12099,#12100,#6271,.T.);
#15283=EDGE_CURVE('',#12099,#12101,#6272,.T.);
#15284=EDGE_CURVE('',#12102,#12100,#6273,.T.);
#15285=EDGE_CURVE('',#12101,#12102,#6274,.T.);
#15286=EDGE_CURVE('',#12101,#12103,#6275,.T.);
#15287=EDGE_CURVE('',#12104,#12102,#6276,.T.);
#15288=EDGE_CURVE('',#12103,#12104,#6277,.T.);
#15289=EDGE_CURVE('',#12103,#12105,#6278,.T.);
#15290=EDGE_CURVE('',#12106,#12104,#6279,.T.);
#15291=EDGE_CURVE('',#12105,#12106,#6280,.T.);
#15292=EDGE_CURVE('',#12105,#12107,#6281,.T.);
#15293=EDGE_CURVE('',#12108,#12106,#6282,.T.);
#15294=EDGE_CURVE('',#12107,#12108,#6283,.T.);
#15295=EDGE_CURVE('',#12107,#12109,#6284,.T.);
#15296=EDGE_CURVE('',#12110,#12108,#6285,.T.);
#15297=EDGE_CURVE('',#12109,#12110,#6286,.T.);
#15298=EDGE_CURVE('',#12109,#12111,#6287,.T.);
#15299=EDGE_CURVE('',#12112,#12110,#6288,.T.);
#15300=EDGE_CURVE('',#12111,#12112,#6289,.T.);
#15301=EDGE_CURVE('',#12111,#12113,#6290,.T.);
#15302=EDGE_CURVE('',#12114,#12112,#6291,.T.);
#15303=EDGE_CURVE('',#12113,#12114,#6292,.T.);
#15304=EDGE_CURVE('',#12113,#12115,#6293,.T.);
#15305=EDGE_CURVE('',#12116,#12114,#6294,.T.);
#15306=EDGE_CURVE('',#12115,#12116,#6295,.T.);
#15307=EDGE_CURVE('',#12115,#12117,#6296,.T.);
#15308=EDGE_CURVE('',#12118,#12116,#6297,.T.);
#15309=EDGE_CURVE('',#12117,#12118,#6298,.T.);
#15310=EDGE_CURVE('',#12117,#12119,#6299,.T.);
#15311=EDGE_CURVE('',#12120,#12118,#6300,.T.);
#15312=EDGE_CURVE('',#12119,#12120,#6301,.T.);
#15313=EDGE_CURVE('',#12119,#12121,#6302,.T.);
#15314=EDGE_CURVE('',#12122,#12120,#6303,.T.);
#15315=EDGE_CURVE('',#12121,#12122,#6304,.T.);
#15316=EDGE_CURVE('',#12121,#12123,#6305,.T.);
#15317=EDGE_CURVE('',#12124,#12122,#6306,.T.);
#15318=EDGE_CURVE('',#12123,#12124,#6307,.T.);
#15319=EDGE_CURVE('',#12123,#12125,#6308,.T.);
#15320=EDGE_CURVE('',#12126,#12124,#6309,.T.);
#15321=EDGE_CURVE('',#12125,#12126,#6310,.T.);
#15322=EDGE_CURVE('',#12125,#12127,#6311,.T.);
#15323=EDGE_CURVE('',#12128,#12126,#6312,.T.);
#15324=EDGE_CURVE('',#12127,#12128,#6313,.T.);
#15325=EDGE_CURVE('',#12127,#12129,#6314,.T.);
#15326=EDGE_CURVE('',#12130,#12128,#6315,.T.);
#15327=EDGE_CURVE('',#12129,#12130,#6316,.T.);
#15328=EDGE_CURVE('',#12129,#12131,#6317,.T.);
#15329=EDGE_CURVE('',#12132,#12130,#6318,.T.);
#15330=EDGE_CURVE('',#12131,#12132,#6319,.T.);
#15331=EDGE_CURVE('',#12131,#12133,#6320,.T.);
#15332=EDGE_CURVE('',#12134,#12132,#6321,.T.);
#15333=EDGE_CURVE('',#12133,#12134,#6322,.T.);
#15334=EDGE_CURVE('',#12133,#12135,#6323,.T.);
#15335=EDGE_CURVE('',#12136,#12134,#6324,.T.);
#15336=EDGE_CURVE('',#12135,#12136,#6325,.T.);
#15337=EDGE_CURVE('',#12135,#12137,#6326,.T.);
#15338=EDGE_CURVE('',#12138,#12136,#6327,.T.);
#15339=EDGE_CURVE('',#12137,#12138,#6328,.T.);
#15340=EDGE_CURVE('',#12137,#12139,#6329,.T.);
#15341=EDGE_CURVE('',#12140,#12138,#6330,.T.);
#15342=EDGE_CURVE('',#12139,#12140,#6331,.T.);
#15343=EDGE_CURVE('',#12139,#12141,#6332,.T.);
#15344=EDGE_CURVE('',#12142,#12140,#6333,.T.);
#15345=EDGE_CURVE('',#12141,#12142,#6334,.T.);
#15346=EDGE_CURVE('',#12141,#12143,#6335,.T.);
#15347=EDGE_CURVE('',#12144,#12142,#6336,.T.);
#15348=EDGE_CURVE('',#12143,#12144,#6337,.T.);
#15349=EDGE_CURVE('',#12143,#12145,#6338,.T.);
#15350=EDGE_CURVE('',#12146,#12144,#6339,.T.);
#15351=EDGE_CURVE('',#12145,#12146,#6340,.T.);
#15352=EDGE_CURVE('',#12145,#12147,#6341,.T.);
#15353=EDGE_CURVE('',#12148,#12146,#6342,.T.);
#15354=EDGE_CURVE('',#12147,#12148,#6343,.T.);
#15355=EDGE_CURVE('',#12147,#12149,#6344,.T.);
#15356=EDGE_CURVE('',#12150,#12148,#6345,.T.);
#15357=EDGE_CURVE('',#12149,#12150,#6346,.T.);
#15358=EDGE_CURVE('',#12149,#12151,#6347,.T.);
#15359=EDGE_CURVE('',#12152,#12150,#6348,.T.);
#15360=EDGE_CURVE('',#12151,#12152,#6349,.T.);
#15361=EDGE_CURVE('',#12151,#12153,#6350,.T.);
#15362=EDGE_CURVE('',#12154,#12152,#6351,.T.);
#15363=EDGE_CURVE('',#12153,#12154,#6352,.T.);
#15364=EDGE_CURVE('',#12153,#12155,#6353,.T.);
#15365=EDGE_CURVE('',#12156,#12154,#6354,.T.);
#15366=EDGE_CURVE('',#12155,#12156,#6355,.T.);
#15367=EDGE_CURVE('',#12155,#12157,#6356,.T.);
#15368=EDGE_CURVE('',#12158,#12156,#6357,.T.);
#15369=EDGE_CURVE('',#12157,#12158,#6358,.T.);
#15370=EDGE_CURVE('',#12157,#12159,#6359,.T.);
#15371=EDGE_CURVE('',#12160,#12158,#6360,.T.);
#15372=EDGE_CURVE('',#12159,#12160,#6361,.T.);
#15373=EDGE_CURVE('',#12159,#12161,#6362,.T.);
#15374=EDGE_CURVE('',#12162,#12160,#6363,.T.);
#15375=EDGE_CURVE('',#12161,#12162,#6364,.T.);
#15376=EDGE_CURVE('',#12161,#12163,#6365,.T.);
#15377=EDGE_CURVE('',#12164,#12162,#6366,.T.);
#15378=EDGE_CURVE('',#12163,#12164,#6367,.T.);
#15379=EDGE_CURVE('',#12163,#12165,#6368,.T.);
#15380=EDGE_CURVE('',#12166,#12164,#6369,.T.);
#15381=EDGE_CURVE('',#12165,#12166,#6370,.T.);
#15382=EDGE_CURVE('',#12165,#12167,#6371,.T.);
#15383=EDGE_CURVE('',#12168,#12166,#6372,.T.);
#15384=EDGE_CURVE('',#12167,#12168,#6373,.T.);
#15385=EDGE_CURVE('',#12167,#12169,#6374,.T.);
#15386=EDGE_CURVE('',#12170,#12168,#6375,.T.);
#15387=EDGE_CURVE('',#12169,#12170,#6376,.T.);
#15388=EDGE_CURVE('',#12169,#12171,#6377,.T.);
#15389=EDGE_CURVE('',#12172,#12170,#6378,.T.);
#15390=EDGE_CURVE('',#12171,#12172,#6379,.T.);
#15391=EDGE_CURVE('',#12171,#12173,#6380,.T.);
#15392=EDGE_CURVE('',#12174,#12172,#6381,.T.);
#15393=EDGE_CURVE('',#12173,#12174,#6382,.T.);
#15394=EDGE_CURVE('',#12173,#12175,#6383,.T.);
#15395=EDGE_CURVE('',#12176,#12174,#6384,.T.);
#15396=EDGE_CURVE('',#12175,#12176,#6385,.T.);
#15397=EDGE_CURVE('',#12175,#12177,#6386,.T.);
#15398=EDGE_CURVE('',#12178,#12176,#6387,.T.);
#15399=EDGE_CURVE('',#12177,#12178,#6388,.T.);
#15400=EDGE_CURVE('',#12177,#12179,#6389,.T.);
#15401=EDGE_CURVE('',#12180,#12178,#6390,.T.);
#15402=EDGE_CURVE('',#12179,#12180,#6391,.T.);
#15403=EDGE_CURVE('',#12179,#12181,#6392,.T.);
#15404=EDGE_CURVE('',#12182,#12180,#6393,.T.);
#15405=EDGE_CURVE('',#12181,#12182,#6394,.T.);
#15406=EDGE_CURVE('',#12181,#12183,#6395,.T.);
#15407=EDGE_CURVE('',#12184,#12182,#6396,.T.);
#15408=EDGE_CURVE('',#12183,#12184,#6397,.T.);
#15409=EDGE_CURVE('',#12183,#12185,#6398,.T.);
#15410=EDGE_CURVE('',#12186,#12184,#6399,.T.);
#15411=EDGE_CURVE('',#12185,#12186,#6400,.T.);
#15412=EDGE_CURVE('',#12185,#12187,#6401,.T.);
#15413=EDGE_CURVE('',#12188,#12186,#6402,.T.);
#15414=EDGE_CURVE('',#12187,#12188,#6403,.T.);
#15415=EDGE_CURVE('',#12187,#12189,#6404,.T.);
#15416=EDGE_CURVE('',#12190,#12188,#6405,.T.);
#15417=EDGE_CURVE('',#12189,#12190,#6406,.T.);
#15418=EDGE_CURVE('',#12189,#12191,#6407,.T.);
#15419=EDGE_CURVE('',#12192,#12190,#6408,.T.);
#15420=EDGE_CURVE('',#12191,#12192,#6409,.T.);
#15421=EDGE_CURVE('',#12191,#12193,#6410,.T.);
#15422=EDGE_CURVE('',#12194,#12192,#6411,.T.);
#15423=EDGE_CURVE('',#12193,#12194,#6412,.T.);
#15424=EDGE_CURVE('',#12193,#12195,#6413,.T.);
#15425=EDGE_CURVE('',#12196,#12194,#6414,.T.);
#15426=EDGE_CURVE('',#12195,#12196,#6415,.T.);
#15427=EDGE_CURVE('',#12195,#12197,#6416,.T.);
#15428=EDGE_CURVE('',#12198,#12196,#6417,.T.);
#15429=EDGE_CURVE('',#12197,#12198,#6418,.T.);
#15430=EDGE_CURVE('',#12197,#12199,#6419,.T.);
#15431=EDGE_CURVE('',#12200,#12198,#6420,.T.);
#15432=EDGE_CURVE('',#12199,#12200,#6421,.T.);
#15433=EDGE_CURVE('',#12199,#12201,#6422,.T.);
#15434=EDGE_CURVE('',#12202,#12200,#6423,.T.);
#15435=EDGE_CURVE('',#12201,#12202,#6424,.T.);
#15436=EDGE_CURVE('',#12201,#12203,#6425,.T.);
#15437=EDGE_CURVE('',#12204,#12202,#6426,.T.);
#15438=EDGE_CURVE('',#12203,#12204,#6427,.T.);
#15439=EDGE_CURVE('',#12203,#12205,#6428,.T.);
#15440=EDGE_CURVE('',#12206,#12204,#6429,.T.);
#15441=EDGE_CURVE('',#12205,#12206,#6430,.T.);
#15442=EDGE_CURVE('',#12205,#12207,#6431,.T.);
#15443=EDGE_CURVE('',#12208,#12206,#6432,.T.);
#15444=EDGE_CURVE('',#12207,#12208,#6433,.T.);
#15445=EDGE_CURVE('',#12207,#12209,#6434,.T.);
#15446=EDGE_CURVE('',#12210,#12208,#6435,.T.);
#15447=EDGE_CURVE('',#12209,#12210,#6436,.T.);
#15448=EDGE_CURVE('',#12209,#12211,#6437,.T.);
#15449=EDGE_CURVE('',#12212,#12210,#6438,.T.);
#15450=EDGE_CURVE('',#12211,#12212,#6439,.T.);
#15451=EDGE_CURVE('',#12211,#12213,#6440,.T.);
#15452=EDGE_CURVE('',#12214,#12212,#6441,.T.);
#15453=EDGE_CURVE('',#12213,#12214,#6442,.T.);
#15454=EDGE_CURVE('',#12213,#12215,#6443,.T.);
#15455=EDGE_CURVE('',#12216,#12214,#6444,.T.);
#15456=EDGE_CURVE('',#12215,#12216,#6445,.T.);
#15457=EDGE_CURVE('',#12215,#12217,#6446,.T.);
#15458=EDGE_CURVE('',#12218,#12216,#6447,.T.);
#15459=EDGE_CURVE('',#12217,#12218,#6448,.T.);
#15460=EDGE_CURVE('',#12217,#12219,#6449,.T.);
#15461=EDGE_CURVE('',#12220,#12218,#6450,.T.);
#15462=EDGE_CURVE('',#12219,#12220,#6451,.T.);
#15463=EDGE_CURVE('',#12219,#12221,#6452,.T.);
#15464=EDGE_CURVE('',#12222,#12220,#6453,.T.);
#15465=EDGE_CURVE('',#12221,#12222,#6454,.T.);
#15466=EDGE_CURVE('',#12221,#12223,#6455,.T.);
#15467=EDGE_CURVE('',#12224,#12222,#6456,.T.);
#15468=EDGE_CURVE('',#12223,#12224,#6457,.T.);
#15469=EDGE_CURVE('',#12223,#12225,#6458,.T.);
#15470=EDGE_CURVE('',#12226,#12224,#6459,.T.);
#15471=EDGE_CURVE('',#12225,#12226,#6460,.T.);
#15472=EDGE_CURVE('',#12225,#12227,#6461,.T.);
#15473=EDGE_CURVE('',#12228,#12226,#6462,.T.);
#15474=EDGE_CURVE('',#12227,#12228,#6463,.T.);
#15475=EDGE_CURVE('',#12227,#12229,#6464,.T.);
#15476=EDGE_CURVE('',#12230,#12228,#6465,.T.);
#15477=EDGE_CURVE('',#12229,#12230,#6466,.T.);
#15478=EDGE_CURVE('',#12229,#12231,#6467,.T.);
#15479=EDGE_CURVE('',#12232,#12230,#6468,.T.);
#15480=EDGE_CURVE('',#12231,#12232,#6469,.T.);
#15481=EDGE_CURVE('',#12231,#12233,#6470,.T.);
#15482=EDGE_CURVE('',#12234,#12232,#6471,.T.);
#15483=EDGE_CURVE('',#12233,#12234,#6472,.T.);
#15484=EDGE_CURVE('',#12233,#12235,#6473,.T.);
#15485=EDGE_CURVE('',#12236,#12234,#6474,.T.);
#15486=EDGE_CURVE('',#12235,#12236,#6475,.T.);
#15487=EDGE_CURVE('',#12235,#12237,#6476,.T.);
#15488=EDGE_CURVE('',#12238,#12236,#6477,.T.);
#15489=EDGE_CURVE('',#12237,#12238,#6478,.T.);
#15490=EDGE_CURVE('',#12237,#12239,#6479,.T.);
#15491=EDGE_CURVE('',#12240,#12238,#6480,.T.);
#15492=EDGE_CURVE('',#12239,#12240,#6481,.T.);
#15493=EDGE_CURVE('',#12239,#12241,#6482,.T.);
#15494=EDGE_CURVE('',#12242,#12240,#6483,.T.);
#15495=EDGE_CURVE('',#12241,#12242,#6484,.T.);
#15496=EDGE_CURVE('',#12241,#12243,#6485,.T.);
#15497=EDGE_CURVE('',#12244,#12242,#6486,.T.);
#15498=EDGE_CURVE('',#12243,#12244,#6487,.T.);
#15499=EDGE_CURVE('',#12243,#12245,#6488,.T.);
#15500=EDGE_CURVE('',#12246,#12244,#6489,.T.);
#15501=EDGE_CURVE('',#12245,#12246,#6490,.T.);
#15502=EDGE_CURVE('',#12245,#12247,#6491,.T.);
#15503=EDGE_CURVE('',#12248,#12246,#6492,.T.);
#15504=EDGE_CURVE('',#12247,#12248,#6493,.T.);
#15505=EDGE_CURVE('',#12247,#12249,#6494,.T.);
#15506=EDGE_CURVE('',#12250,#12248,#6495,.T.);
#15507=EDGE_CURVE('',#12249,#12250,#6496,.T.);
#15508=EDGE_CURVE('',#12249,#12251,#6497,.T.);
#15509=EDGE_CURVE('',#12252,#12250,#6498,.T.);
#15510=EDGE_CURVE('',#12251,#12252,#6499,.T.);
#15511=EDGE_CURVE('',#12251,#12253,#6500,.T.);
#15512=EDGE_CURVE('',#12254,#12252,#6501,.T.);
#15513=EDGE_CURVE('',#12253,#12254,#6502,.T.);
#15514=EDGE_CURVE('',#12253,#12255,#6503,.T.);
#15515=EDGE_CURVE('',#12256,#12254,#6504,.T.);
#15516=EDGE_CURVE('',#12255,#12256,#6505,.T.);
#15517=EDGE_CURVE('',#12255,#12257,#6506,.T.);
#15518=EDGE_CURVE('',#12258,#12256,#6507,.T.);
#15519=EDGE_CURVE('',#12257,#12258,#6508,.T.);
#15520=EDGE_CURVE('',#12257,#12259,#6509,.T.);
#15521=EDGE_CURVE('',#12260,#12258,#6510,.T.);
#15522=EDGE_CURVE('',#12259,#12260,#6511,.T.);
#15523=EDGE_CURVE('',#12259,#12261,#6512,.T.);
#15524=EDGE_CURVE('',#12262,#12260,#6513,.T.);
#15525=EDGE_CURVE('',#12261,#12262,#6514,.T.);
#15526=EDGE_CURVE('',#12261,#12263,#6515,.T.);
#15527=EDGE_CURVE('',#12264,#12262,#6516,.T.);
#15528=EDGE_CURVE('',#12263,#12264,#6517,.T.);
#15529=EDGE_CURVE('',#12263,#12265,#6518,.T.);
#15530=EDGE_CURVE('',#12266,#12264,#6519,.T.);
#15531=EDGE_CURVE('',#12265,#12266,#6520,.T.);
#15532=EDGE_CURVE('',#12265,#12267,#6521,.T.);
#15533=EDGE_CURVE('',#12268,#12266,#6522,.T.);
#15534=EDGE_CURVE('',#12267,#12268,#6523,.T.);
#15535=EDGE_CURVE('',#12267,#12269,#6524,.T.);
#15536=EDGE_CURVE('',#12270,#12268,#6525,.T.);
#15537=EDGE_CURVE('',#12269,#12270,#6526,.T.);
#15538=EDGE_CURVE('',#12269,#12271,#6527,.T.);
#15539=EDGE_CURVE('',#12272,#12270,#6528,.T.);
#15540=EDGE_CURVE('',#12271,#12272,#6529,.T.);
#15541=EDGE_CURVE('',#12271,#12273,#6530,.T.);
#15542=EDGE_CURVE('',#12274,#12272,#6531,.T.);
#15543=EDGE_CURVE('',#12273,#12274,#6532,.T.);
#15544=EDGE_CURVE('',#12273,#12275,#6533,.T.);
#15545=EDGE_CURVE('',#12276,#12274,#6534,.T.);
#15546=EDGE_CURVE('',#12275,#12276,#6535,.T.);
#15547=EDGE_CURVE('',#12275,#12277,#6536,.T.);
#15548=EDGE_CURVE('',#12278,#12276,#6537,.T.);
#15549=EDGE_CURVE('',#12277,#12278,#6538,.T.);
#15550=EDGE_CURVE('',#12277,#12279,#6539,.T.);
#15551=EDGE_CURVE('',#12280,#12278,#6540,.T.);
#15552=EDGE_CURVE('',#12279,#12280,#6541,.T.);
#15553=EDGE_CURVE('',#12279,#12281,#6542,.T.);
#15554=EDGE_CURVE('',#12282,#12280,#6543,.T.);
#15555=EDGE_CURVE('',#12281,#12282,#6544,.T.);
#15556=EDGE_CURVE('',#12281,#12283,#6545,.T.);
#15557=EDGE_CURVE('',#12284,#12282,#6546,.T.);
#15558=EDGE_CURVE('',#12283,#12284,#6547,.T.);
#15559=EDGE_CURVE('',#12283,#12285,#6548,.T.);
#15560=EDGE_CURVE('',#12286,#12284,#6549,.T.);
#15561=EDGE_CURVE('',#12285,#12286,#6550,.T.);
#15562=EDGE_CURVE('',#12285,#12287,#6551,.T.);
#15563=EDGE_CURVE('',#12288,#12286,#6552,.T.);
#15564=EDGE_CURVE('',#12287,#12288,#6553,.T.);
#15565=EDGE_CURVE('',#12287,#12289,#6554,.T.);
#15566=EDGE_CURVE('',#12290,#12288,#6555,.T.);
#15567=EDGE_CURVE('',#12289,#12290,#6556,.T.);
#15568=EDGE_CURVE('',#12289,#12291,#6557,.T.);
#15569=EDGE_CURVE('',#12292,#12290,#6558,.T.);
#15570=EDGE_CURVE('',#12291,#12292,#6559,.T.);
#15571=EDGE_CURVE('',#12291,#12293,#6560,.T.);
#15572=EDGE_CURVE('',#12294,#12292,#6561,.T.);
#15573=EDGE_CURVE('',#12293,#12294,#6562,.T.);
#15574=EDGE_CURVE('',#12293,#12295,#6563,.T.);
#15575=EDGE_CURVE('',#12296,#12294,#6564,.T.);
#15576=EDGE_CURVE('',#12295,#12296,#6565,.T.);
#15577=EDGE_CURVE('',#12295,#12297,#6566,.T.);
#15578=EDGE_CURVE('',#12298,#12296,#6567,.T.);
#15579=EDGE_CURVE('',#12297,#12298,#6568,.T.);
#15580=EDGE_CURVE('',#12297,#12299,#6569,.T.);
#15581=EDGE_CURVE('',#12300,#12298,#6570,.T.);
#15582=EDGE_CURVE('',#12299,#12300,#6571,.T.);
#15583=EDGE_CURVE('',#12299,#12301,#6572,.T.);
#15584=EDGE_CURVE('',#12302,#12300,#6573,.T.);
#15585=EDGE_CURVE('',#12301,#12302,#6574,.T.);
#15586=EDGE_CURVE('',#12301,#12303,#6575,.T.);
#15587=EDGE_CURVE('',#12304,#12302,#6576,.T.);
#15588=EDGE_CURVE('',#12303,#12304,#6577,.T.);
#15589=EDGE_CURVE('',#12303,#12305,#6578,.T.);
#15590=EDGE_CURVE('',#12306,#12304,#6579,.T.);
#15591=EDGE_CURVE('',#12305,#12306,#6580,.T.);
#15592=EDGE_CURVE('',#12305,#12307,#6581,.T.);
#15593=EDGE_CURVE('',#12308,#12306,#6582,.T.);
#15594=EDGE_CURVE('',#12307,#12308,#6583,.T.);
#15595=EDGE_CURVE('',#12307,#12309,#6584,.T.);
#15596=EDGE_CURVE('',#12310,#12308,#6585,.T.);
#15597=EDGE_CURVE('',#12309,#12310,#6586,.T.);
#15598=EDGE_CURVE('',#12309,#12311,#6587,.T.);
#15599=EDGE_CURVE('',#12312,#12310,#6588,.T.);
#15600=EDGE_CURVE('',#12311,#12312,#6589,.T.);
#15601=EDGE_CURVE('',#12311,#12313,#6590,.T.);
#15602=EDGE_CURVE('',#12314,#12312,#6591,.T.);
#15603=EDGE_CURVE('',#12313,#12314,#6592,.T.);
#15604=EDGE_CURVE('',#12313,#12315,#6593,.T.);
#15605=EDGE_CURVE('',#12316,#12314,#6594,.T.);
#15606=EDGE_CURVE('',#12315,#12316,#6595,.T.);
#15607=EDGE_CURVE('',#12315,#12317,#6596,.T.);
#15608=EDGE_CURVE('',#12318,#12316,#6597,.T.);
#15609=EDGE_CURVE('',#12317,#12318,#6598,.T.);
#15610=EDGE_CURVE('',#12317,#12319,#6599,.T.);
#15611=EDGE_CURVE('',#12320,#12318,#6600,.T.);
#15612=EDGE_CURVE('',#12319,#12320,#6601,.T.);
#15613=EDGE_CURVE('',#12319,#12321,#6602,.T.);
#15614=EDGE_CURVE('',#12322,#12320,#6603,.T.);
#15615=EDGE_CURVE('',#12321,#12322,#6604,.T.);
#15616=EDGE_CURVE('',#12321,#12323,#6605,.T.);
#15617=EDGE_CURVE('',#12324,#12322,#6606,.T.);
#15618=EDGE_CURVE('',#12323,#12324,#6607,.T.);
#15619=EDGE_CURVE('',#12323,#12325,#6608,.T.);
#15620=EDGE_CURVE('',#12326,#12324,#6609,.T.);
#15621=EDGE_CURVE('',#12325,#12326,#6610,.T.);
#15622=EDGE_CURVE('',#12325,#12327,#6611,.T.);
#15623=EDGE_CURVE('',#12328,#12326,#6612,.T.);
#15624=EDGE_CURVE('',#12327,#12328,#6613,.T.);
#15625=EDGE_CURVE('',#12327,#12329,#6614,.T.);
#15626=EDGE_CURVE('',#12330,#12328,#6615,.T.);
#15627=EDGE_CURVE('',#12329,#12330,#6616,.T.);
#15628=EDGE_CURVE('',#12329,#12331,#6617,.T.);
#15629=EDGE_CURVE('',#12332,#12330,#6618,.T.);
#15630=EDGE_CURVE('',#12331,#12332,#6619,.T.);
#15631=EDGE_CURVE('',#12331,#12333,#6620,.T.);
#15632=EDGE_CURVE('',#12334,#12332,#6621,.T.);
#15633=EDGE_CURVE('',#12333,#12334,#6622,.T.);
#15634=EDGE_CURVE('',#12333,#12335,#6623,.T.);
#15635=EDGE_CURVE('',#12336,#12334,#6624,.T.);
#15636=EDGE_CURVE('',#12335,#12336,#6625,.T.);
#15637=EDGE_CURVE('',#12335,#12337,#6626,.T.);
#15638=EDGE_CURVE('',#12338,#12336,#6627,.T.);
#15639=EDGE_CURVE('',#12337,#12338,#6628,.T.);
#15640=EDGE_CURVE('',#12337,#12339,#6629,.T.);
#15641=EDGE_CURVE('',#12340,#12338,#6630,.T.);
#15642=EDGE_CURVE('',#12339,#12340,#6631,.T.);
#15643=EDGE_CURVE('',#12339,#12341,#6632,.T.);
#15644=EDGE_CURVE('',#12342,#12340,#6633,.T.);
#15645=EDGE_CURVE('',#12341,#12342,#6634,.T.);
#15646=EDGE_CURVE('',#12341,#12343,#6635,.T.);
#15647=EDGE_CURVE('',#12344,#12342,#6636,.T.);
#15648=EDGE_CURVE('',#12343,#12344,#6637,.T.);
#15649=EDGE_CURVE('',#12343,#12345,#6638,.T.);
#15650=EDGE_CURVE('',#12346,#12344,#6639,.T.);
#15651=EDGE_CURVE('',#12345,#12346,#6640,.T.);
#15652=EDGE_CURVE('',#12345,#12347,#6641,.T.);
#15653=EDGE_CURVE('',#12348,#12346,#6642,.T.);
#15654=EDGE_CURVE('',#12347,#12348,#6643,.T.);
#15655=EDGE_CURVE('',#12347,#12349,#6644,.T.);
#15656=EDGE_CURVE('',#12350,#12348,#6645,.T.);
#15657=EDGE_CURVE('',#12349,#12350,#6646,.T.);
#15658=EDGE_CURVE('',#12349,#12351,#6647,.T.);
#15659=EDGE_CURVE('',#12352,#12350,#6648,.T.);
#15660=EDGE_CURVE('',#12351,#12352,#6649,.T.);
#15661=EDGE_CURVE('',#12351,#12353,#6650,.T.);
#15662=EDGE_CURVE('',#12354,#12352,#6651,.T.);
#15663=EDGE_CURVE('',#12353,#12354,#6652,.T.);
#15664=EDGE_CURVE('',#12353,#12355,#6653,.T.);
#15665=EDGE_CURVE('',#12356,#12354,#6654,.T.);
#15666=EDGE_CURVE('',#12355,#12356,#6655,.T.);
#15667=EDGE_CURVE('',#12355,#12357,#6656,.T.);
#15668=EDGE_CURVE('',#12358,#12356,#6657,.T.);
#15669=EDGE_CURVE('',#12357,#12358,#6658,.T.);
#15670=EDGE_CURVE('',#12357,#12359,#6659,.T.);
#15671=EDGE_CURVE('',#12360,#12358,#6660,.T.);
#15672=EDGE_CURVE('',#12359,#12360,#6661,.T.);
#15673=EDGE_CURVE('',#12359,#12361,#6662,.T.);
#15674=EDGE_CURVE('',#12362,#12360,#6663,.T.);
#15675=EDGE_CURVE('',#12361,#12362,#6664,.T.);
#15676=EDGE_CURVE('',#12361,#12363,#6665,.T.);
#15677=EDGE_CURVE('',#12364,#12362,#6666,.T.);
#15678=EDGE_CURVE('',#12363,#12364,#6667,.T.);
#15679=EDGE_CURVE('',#12363,#12365,#6668,.T.);
#15680=EDGE_CURVE('',#12366,#12364,#6669,.T.);
#15681=EDGE_CURVE('',#12365,#12366,#6670,.T.);
#15682=EDGE_CURVE('',#12365,#12367,#6671,.T.);
#15683=EDGE_CURVE('',#12368,#12366,#6672,.T.);
#15684=EDGE_CURVE('',#12367,#12368,#6673,.T.);
#15685=EDGE_CURVE('',#12367,#12369,#6674,.T.);
#15686=EDGE_CURVE('',#12370,#12368,#6675,.T.);
#15687=EDGE_CURVE('',#12369,#12370,#6676,.T.);
#15688=EDGE_CURVE('',#12369,#12371,#6677,.T.);
#15689=EDGE_CURVE('',#12372,#12370,#6678,.T.);
#15690=EDGE_CURVE('',#12371,#12372,#6679,.T.);
#15691=EDGE_CURVE('',#12371,#12373,#6680,.T.);
#15692=EDGE_CURVE('',#12374,#12372,#6681,.T.);
#15693=EDGE_CURVE('',#12373,#12374,#6682,.T.);
#15694=EDGE_CURVE('',#12373,#12375,#6683,.T.);
#15695=EDGE_CURVE('',#12376,#12374,#6684,.T.);
#15696=EDGE_CURVE('',#12375,#12376,#6685,.T.);
#15697=EDGE_CURVE('',#12375,#12377,#6686,.T.);
#15698=EDGE_CURVE('',#12378,#12376,#6687,.T.);
#15699=EDGE_CURVE('',#12377,#12378,#6688,.T.);
#15700=EDGE_CURVE('',#12377,#12379,#6689,.T.);
#15701=EDGE_CURVE('',#12380,#12378,#6690,.T.);
#15702=EDGE_CURVE('',#12379,#12380,#6691,.T.);
#15703=EDGE_CURVE('',#12379,#12381,#6692,.T.);
#15704=EDGE_CURVE('',#12382,#12380,#6693,.T.);
#15705=EDGE_CURVE('',#12381,#12382,#6694,.T.);
#15706=EDGE_CURVE('',#12381,#12383,#6695,.T.);
#15707=EDGE_CURVE('',#12384,#12382,#6696,.T.);
#15708=EDGE_CURVE('',#12383,#12384,#6697,.T.);
#15709=EDGE_CURVE('',#12383,#12385,#6698,.T.);
#15710=EDGE_CURVE('',#12386,#12384,#6699,.T.);
#15711=EDGE_CURVE('',#12385,#12386,#6700,.T.);
#15712=EDGE_CURVE('',#12385,#12387,#6701,.T.);
#15713=EDGE_CURVE('',#12388,#12386,#6702,.T.);
#15714=EDGE_CURVE('',#12387,#12388,#6703,.T.);
#15715=EDGE_CURVE('',#12387,#12389,#6704,.T.);
#15716=EDGE_CURVE('',#12390,#12388,#6705,.T.);
#15717=EDGE_CURVE('',#12389,#12390,#6706,.T.);
#15718=EDGE_CURVE('',#12389,#12391,#6707,.T.);
#15719=EDGE_CURVE('',#12392,#12390,#6708,.T.);
#15720=EDGE_CURVE('',#12391,#12392,#6709,.T.);
#15721=EDGE_CURVE('',#12391,#12393,#6710,.T.);
#15722=EDGE_CURVE('',#12394,#12392,#6711,.T.);
#15723=EDGE_CURVE('',#12393,#12394,#6712,.T.);
#15724=EDGE_CURVE('',#12393,#12395,#6713,.T.);
#15725=EDGE_CURVE('',#12396,#12394,#6714,.T.);
#15726=EDGE_CURVE('',#12395,#12396,#6715,.T.);
#15727=EDGE_CURVE('',#12395,#12397,#6716,.T.);
#15728=EDGE_CURVE('',#12398,#12396,#6717,.T.);
#15729=EDGE_CURVE('',#12397,#12398,#6718,.T.);
#15730=EDGE_CURVE('',#12397,#12399,#6719,.T.);
#15731=EDGE_CURVE('',#12400,#12398,#6720,.T.);
#15732=EDGE_CURVE('',#12399,#12400,#6721,.T.);
#15733=EDGE_CURVE('',#12399,#12401,#6722,.T.);
#15734=EDGE_CURVE('',#12402,#12400,#6723,.T.);
#15735=EDGE_CURVE('',#12401,#12402,#6724,.T.);
#15736=EDGE_CURVE('',#12401,#12403,#6725,.T.);
#15737=EDGE_CURVE('',#12404,#12402,#6726,.T.);
#15738=EDGE_CURVE('',#12403,#12404,#6727,.T.);
#15739=EDGE_CURVE('',#12403,#12405,#6728,.T.);
#15740=EDGE_CURVE('',#12406,#12404,#6729,.T.);
#15741=EDGE_CURVE('',#12405,#12406,#6730,.T.);
#15742=EDGE_CURVE('',#12405,#12407,#6731,.T.);
#15743=EDGE_CURVE('',#12408,#12406,#6732,.T.);
#15744=EDGE_CURVE('',#12407,#12408,#6733,.T.);
#15745=EDGE_CURVE('',#12407,#12409,#6734,.T.);
#15746=EDGE_CURVE('',#12410,#12408,#6735,.T.);
#15747=EDGE_CURVE('',#12409,#12410,#6736,.T.);
#15748=EDGE_CURVE('',#12409,#12411,#6737,.T.);
#15749=EDGE_CURVE('',#12412,#12410,#6738,.T.);
#15750=EDGE_CURVE('',#12411,#12412,#6739,.T.);
#15751=EDGE_CURVE('',#12411,#12413,#6740,.T.);
#15752=EDGE_CURVE('',#12414,#12412,#6741,.T.);
#15753=EDGE_CURVE('',#12413,#12414,#6742,.T.);
#15754=EDGE_CURVE('',#12413,#12415,#6743,.T.);
#15755=EDGE_CURVE('',#12416,#12414,#6744,.T.);
#15756=EDGE_CURVE('',#12415,#12416,#6745,.T.);
#15757=EDGE_CURVE('',#12415,#12417,#6746,.T.);
#15758=EDGE_CURVE('',#12418,#12416,#6747,.T.);
#15759=EDGE_CURVE('',#12417,#12418,#6748,.T.);
#15760=EDGE_CURVE('',#12417,#12419,#6749,.T.);
#15761=EDGE_CURVE('',#12420,#12418,#6750,.T.);
#15762=EDGE_CURVE('',#12419,#12420,#6751,.T.);
#15763=EDGE_CURVE('',#12419,#12421,#6752,.T.);
#15764=EDGE_CURVE('',#12422,#12420,#6753,.T.);
#15765=EDGE_CURVE('',#12421,#12422,#6754,.T.);
#15766=EDGE_CURVE('',#12421,#12423,#6755,.T.);
#15767=EDGE_CURVE('',#12424,#12422,#6756,.T.);
#15768=EDGE_CURVE('',#12423,#12424,#6757,.T.);
#15769=EDGE_CURVE('',#12423,#12425,#6758,.T.);
#15770=EDGE_CURVE('',#12426,#12424,#6759,.T.);
#15771=EDGE_CURVE('',#12425,#12426,#6760,.T.);
#15772=EDGE_CURVE('',#12425,#12427,#6761,.T.);
#15773=EDGE_CURVE('',#12428,#12426,#6762,.T.);
#15774=EDGE_CURVE('',#12427,#12428,#6763,.T.);
#15775=EDGE_CURVE('',#12427,#12429,#6764,.T.);
#15776=EDGE_CURVE('',#12430,#12428,#6765,.T.);
#15777=EDGE_CURVE('',#12429,#12430,#6766,.T.);
#15778=EDGE_CURVE('',#12429,#12431,#6767,.T.);
#15779=EDGE_CURVE('',#12432,#12430,#6768,.T.);
#15780=EDGE_CURVE('',#12431,#12432,#6769,.T.);
#15781=EDGE_CURVE('',#12431,#12433,#6770,.T.);
#15782=EDGE_CURVE('',#12434,#12432,#6771,.T.);
#15783=EDGE_CURVE('',#12433,#12434,#6772,.T.);
#15784=EDGE_CURVE('',#12433,#12435,#6773,.T.);
#15785=EDGE_CURVE('',#12436,#12434,#6774,.T.);
#15786=EDGE_CURVE('',#12435,#12436,#6775,.T.);
#15787=EDGE_CURVE('',#12435,#12437,#6776,.T.);
#15788=EDGE_CURVE('',#12438,#12436,#6777,.T.);
#15789=EDGE_CURVE('',#12437,#12438,#6778,.T.);
#15790=EDGE_CURVE('',#12437,#12439,#6779,.T.);
#15791=EDGE_CURVE('',#12440,#12438,#6780,.T.);
#15792=EDGE_CURVE('',#12439,#12440,#6781,.T.);
#15793=EDGE_CURVE('',#12439,#12441,#6782,.T.);
#15794=EDGE_CURVE('',#12442,#12440,#6783,.T.);
#15795=EDGE_CURVE('',#12441,#12442,#6784,.T.);
#15796=EDGE_CURVE('',#12441,#12443,#6785,.T.);
#15797=EDGE_CURVE('',#12444,#12442,#6786,.T.);
#15798=EDGE_CURVE('',#12443,#12444,#6787,.T.);
#15799=EDGE_CURVE('',#12443,#12445,#6788,.T.);
#15800=EDGE_CURVE('',#12446,#12444,#6789,.T.);
#15801=EDGE_CURVE('',#12445,#12446,#6790,.T.);
#15802=EDGE_CURVE('',#12445,#12447,#6791,.T.);
#15803=EDGE_CURVE('',#12448,#12446,#6792,.T.);
#15804=EDGE_CURVE('',#12447,#12448,#6793,.T.);
#15805=EDGE_CURVE('',#12447,#12449,#6794,.T.);
#15806=EDGE_CURVE('',#12450,#12448,#6795,.T.);
#15807=EDGE_CURVE('',#12449,#12450,#6796,.T.);
#15808=EDGE_CURVE('',#12449,#12451,#6797,.T.);
#15809=EDGE_CURVE('',#12452,#12450,#6798,.T.);
#15810=EDGE_CURVE('',#12451,#12452,#6799,.T.);
#15811=EDGE_CURVE('',#12451,#12453,#6800,.T.);
#15812=EDGE_CURVE('',#12454,#12452,#6801,.T.);
#15813=EDGE_CURVE('',#12453,#12454,#6802,.T.);
#15814=EDGE_CURVE('',#12453,#12455,#6803,.T.);
#15815=EDGE_CURVE('',#12456,#12454,#6804,.T.);
#15816=EDGE_CURVE('',#12455,#12456,#6805,.T.);
#15817=EDGE_CURVE('',#12455,#12457,#6806,.T.);
#15818=EDGE_CURVE('',#12458,#12456,#6807,.T.);
#15819=EDGE_CURVE('',#12457,#12458,#6808,.T.);
#15820=EDGE_CURVE('',#12457,#12459,#6809,.T.);
#15821=EDGE_CURVE('',#12460,#12458,#6810,.T.);
#15822=EDGE_CURVE('',#12459,#12460,#6811,.T.);
#15823=EDGE_CURVE('',#12459,#12461,#6812,.T.);
#15824=EDGE_CURVE('',#12462,#12460,#6813,.T.);
#15825=EDGE_CURVE('',#12461,#12462,#6814,.T.);
#15826=EDGE_CURVE('',#12461,#12463,#6815,.T.);
#15827=EDGE_CURVE('',#12464,#12462,#6816,.T.);
#15828=EDGE_CURVE('',#12463,#12464,#6817,.T.);
#15829=EDGE_CURVE('',#12463,#12465,#6818,.T.);
#15830=EDGE_CURVE('',#12466,#12464,#6819,.T.);
#15831=EDGE_CURVE('',#12465,#12466,#6820,.T.);
#15832=EDGE_CURVE('',#12465,#12467,#6821,.T.);
#15833=EDGE_CURVE('',#12468,#12466,#6822,.T.);
#15834=EDGE_CURVE('',#12467,#12468,#6823,.T.);
#15835=EDGE_CURVE('',#12467,#12469,#6824,.T.);
#15836=EDGE_CURVE('',#12470,#12468,#6825,.T.);
#15837=EDGE_CURVE('',#12469,#12470,#6826,.T.);
#15838=EDGE_CURVE('',#12469,#12471,#6827,.T.);
#15839=EDGE_CURVE('',#12472,#12470,#6828,.T.);
#15840=EDGE_CURVE('',#12471,#12472,#6829,.T.);
#15841=EDGE_CURVE('',#12471,#12473,#6830,.T.);
#15842=EDGE_CURVE('',#12474,#12472,#6831,.T.);
#15843=EDGE_CURVE('',#12473,#12474,#6832,.T.);
#15844=EDGE_CURVE('',#12473,#12475,#6833,.T.);
#15845=EDGE_CURVE('',#12476,#12474,#6834,.T.);
#15846=EDGE_CURVE('',#12475,#12476,#6835,.T.);
#15847=EDGE_CURVE('',#12475,#12477,#6836,.T.);
#15848=EDGE_CURVE('',#12478,#12476,#6837,.T.);
#15849=EDGE_CURVE('',#12477,#12478,#6838,.T.);
#15850=EDGE_CURVE('',#12477,#12479,#6839,.T.);
#15851=EDGE_CURVE('',#12480,#12478,#6840,.T.);
#15852=EDGE_CURVE('',#12479,#12480,#6841,.T.);
#15853=EDGE_CURVE('',#12479,#12481,#6842,.T.);
#15854=EDGE_CURVE('',#12482,#12480,#6843,.T.);
#15855=EDGE_CURVE('',#12481,#12482,#6844,.T.);
#15856=EDGE_CURVE('',#12481,#12483,#6845,.T.);
#15857=EDGE_CURVE('',#12484,#12482,#6846,.T.);
#15858=EDGE_CURVE('',#12483,#12484,#6847,.T.);
#15859=EDGE_CURVE('',#12483,#12485,#6848,.T.);
#15860=EDGE_CURVE('',#12486,#12484,#6849,.T.);
#15861=EDGE_CURVE('',#12485,#12486,#6850,.T.);
#15862=EDGE_CURVE('',#12485,#12487,#6851,.T.);
#15863=EDGE_CURVE('',#12488,#12486,#6852,.T.);
#15864=EDGE_CURVE('',#12487,#12488,#6853,.T.);
#15865=EDGE_CURVE('',#12487,#12489,#6854,.T.);
#15866=EDGE_CURVE('',#12490,#12488,#6855,.T.);
#15867=EDGE_CURVE('',#12489,#12490,#6856,.T.);
#15868=EDGE_CURVE('',#12489,#12491,#6857,.T.);
#15869=EDGE_CURVE('',#12492,#12490,#6858,.T.);
#15870=EDGE_CURVE('',#12491,#12492,#6859,.T.);
#15871=EDGE_CURVE('',#12491,#12493,#6860,.T.);
#15872=EDGE_CURVE('',#12494,#12492,#6861,.T.);
#15873=EDGE_CURVE('',#12493,#12494,#6862,.T.);
#15874=EDGE_CURVE('',#12493,#12495,#6863,.T.);
#15875=EDGE_CURVE('',#12496,#12494,#6864,.T.);
#15876=EDGE_CURVE('',#12495,#12496,#6865,.T.);
#15877=EDGE_CURVE('',#12495,#12497,#6866,.T.);
#15878=EDGE_CURVE('',#12498,#12496,#6867,.T.);
#15879=EDGE_CURVE('',#12497,#12498,#6868,.T.);
#15880=EDGE_CURVE('',#12497,#12499,#6869,.T.);
#15881=EDGE_CURVE('',#12500,#12498,#6870,.T.);
#15882=EDGE_CURVE('',#12499,#12500,#6871,.T.);
#15883=EDGE_CURVE('',#12499,#12501,#6872,.T.);
#15884=EDGE_CURVE('',#12502,#12500,#6873,.T.);
#15885=EDGE_CURVE('',#12501,#12502,#6874,.T.);
#15886=EDGE_CURVE('',#12501,#12503,#6875,.T.);
#15887=EDGE_CURVE('',#12504,#12502,#6876,.T.);
#15888=EDGE_CURVE('',#12503,#12504,#6877,.T.);
#15889=EDGE_CURVE('',#12503,#12505,#6878,.T.);
#15890=EDGE_CURVE('',#12506,#12504,#6879,.T.);
#15891=EDGE_CURVE('',#12505,#12506,#6880,.T.);
#15892=EDGE_CURVE('',#12505,#12507,#6881,.T.);
#15893=EDGE_CURVE('',#12508,#12506,#6882,.T.);
#15894=EDGE_CURVE('',#12507,#12508,#6883,.T.);
#15895=EDGE_CURVE('',#12507,#12509,#6884,.T.);
#15896=EDGE_CURVE('',#12510,#12508,#6885,.T.);
#15897=EDGE_CURVE('',#12509,#12510,#6886,.T.);
#15898=EDGE_CURVE('',#12509,#12511,#6887,.T.);
#15899=EDGE_CURVE('',#12512,#12510,#6888,.T.);
#15900=EDGE_CURVE('',#12511,#12512,#6889,.T.);
#15901=EDGE_CURVE('',#12511,#12513,#6890,.T.);
#15902=EDGE_CURVE('',#12514,#12512,#6891,.T.);
#15903=EDGE_CURVE('',#12513,#12514,#6892,.T.);
#15904=EDGE_CURVE('',#12513,#12515,#6893,.T.);
#15905=EDGE_CURVE('',#12516,#12514,#6894,.T.);
#15906=EDGE_CURVE('',#12515,#12516,#6895,.T.);
#15907=EDGE_CURVE('',#12515,#12517,#6896,.T.);
#15908=EDGE_CURVE('',#12518,#12516,#6897,.T.);
#15909=EDGE_CURVE('',#12517,#12518,#6898,.T.);
#15910=EDGE_CURVE('',#12517,#12519,#6899,.T.);
#15911=EDGE_CURVE('',#12520,#12518,#6900,.T.);
#15912=EDGE_CURVE('',#12519,#12520,#6901,.T.);
#15913=EDGE_CURVE('',#12519,#12521,#6902,.T.);
#15914=EDGE_CURVE('',#12522,#12520,#6903,.T.);
#15915=EDGE_CURVE('',#12521,#12522,#6904,.T.);
#15916=EDGE_CURVE('',#12521,#12523,#6905,.T.);
#15917=EDGE_CURVE('',#12524,#12522,#6906,.T.);
#15918=EDGE_CURVE('',#12523,#12524,#6907,.T.);
#15919=EDGE_CURVE('',#12523,#12525,#6908,.T.);
#15920=EDGE_CURVE('',#12526,#12524,#6909,.T.);
#15921=EDGE_CURVE('',#12525,#12526,#6910,.T.);
#15922=EDGE_CURVE('',#12525,#12527,#6911,.T.);
#15923=EDGE_CURVE('',#12528,#12526,#6912,.T.);
#15924=EDGE_CURVE('',#12527,#12528,#6913,.T.);
#15925=EDGE_CURVE('',#12527,#12529,#6914,.T.);
#15926=EDGE_CURVE('',#12530,#12528,#6915,.T.);
#15927=EDGE_CURVE('',#12529,#12530,#6916,.T.);
#15928=EDGE_CURVE('',#12529,#12531,#6917,.T.);
#15929=EDGE_CURVE('',#12532,#12530,#6918,.T.);
#15930=EDGE_CURVE('',#12531,#12532,#6919,.T.);
#15931=EDGE_CURVE('',#12531,#12533,#6920,.T.);
#15932=EDGE_CURVE('',#12534,#12532,#6921,.T.);
#15933=EDGE_CURVE('',#12533,#12534,#6922,.T.);
#15934=EDGE_CURVE('',#12533,#12535,#6923,.T.);
#15935=EDGE_CURVE('',#12536,#12534,#6924,.T.);
#15936=EDGE_CURVE('',#12535,#12536,#6925,.T.);
#15937=EDGE_CURVE('',#12535,#12537,#6926,.T.);
#15938=EDGE_CURVE('',#12538,#12536,#6927,.T.);
#15939=EDGE_CURVE('',#12537,#12538,#6928,.T.);
#15940=EDGE_CURVE('',#12537,#12539,#6929,.T.);
#15941=EDGE_CURVE('',#12540,#12538,#6930,.T.);
#15942=EDGE_CURVE('',#12539,#12540,#6931,.T.);
#15943=EDGE_CURVE('',#12539,#12541,#6932,.T.);
#15944=EDGE_CURVE('',#12542,#12540,#6933,.T.);
#15945=EDGE_CURVE('',#12541,#12542,#6934,.T.);
#15946=EDGE_CURVE('',#12541,#12543,#6935,.T.);
#15947=EDGE_CURVE('',#12544,#12542,#6936,.T.);
#15948=EDGE_CURVE('',#12543,#12544,#6937,.T.);
#15949=EDGE_CURVE('',#12543,#12545,#6938,.T.);
#15950=EDGE_CURVE('',#12546,#12544,#6939,.T.);
#15951=EDGE_CURVE('',#12545,#12546,#6940,.T.);
#15952=EDGE_CURVE('',#12545,#12547,#6941,.T.);
#15953=EDGE_CURVE('',#12548,#12546,#6942,.T.);
#15954=EDGE_CURVE('',#12547,#12548,#6943,.T.);
#15955=EDGE_CURVE('',#12547,#12549,#6944,.T.);
#15956=EDGE_CURVE('',#12550,#12548,#6945,.T.);
#15957=EDGE_CURVE('',#12549,#12550,#6946,.T.);
#15958=EDGE_CURVE('',#12549,#12551,#6947,.T.);
#15959=EDGE_CURVE('',#12552,#12550,#6948,.T.);
#15960=EDGE_CURVE('',#12551,#12552,#6949,.T.);
#15961=EDGE_CURVE('',#12551,#12553,#6950,.T.);
#15962=EDGE_CURVE('',#12554,#12552,#6951,.T.);
#15963=EDGE_CURVE('',#12553,#12554,#6952,.T.);
#15964=EDGE_CURVE('',#12553,#12555,#6953,.T.);
#15965=EDGE_CURVE('',#12556,#12554,#6954,.T.);
#15966=EDGE_CURVE('',#12555,#12556,#6955,.T.);
#15967=EDGE_CURVE('',#12555,#12557,#6956,.T.);
#15968=EDGE_CURVE('',#12558,#12556,#6957,.T.);
#15969=EDGE_CURVE('',#12557,#12558,#6958,.T.);
#15970=EDGE_CURVE('',#12557,#12559,#6959,.T.);
#15971=EDGE_CURVE('',#12560,#12558,#6960,.T.);
#15972=EDGE_CURVE('',#12559,#12560,#6961,.T.);
#15973=EDGE_CURVE('',#12559,#12561,#6962,.T.);
#15974=EDGE_CURVE('',#12562,#12560,#6963,.T.);
#15975=EDGE_CURVE('',#12561,#12562,#6964,.T.);
#15976=EDGE_CURVE('',#12561,#12563,#6965,.T.);
#15977=EDGE_CURVE('',#12564,#12562,#6966,.T.);
#15978=EDGE_CURVE('',#12563,#12564,#6967,.T.);
#15979=EDGE_CURVE('',#12563,#12565,#6968,.T.);
#15980=EDGE_CURVE('',#12566,#12564,#6969,.T.);
#15981=EDGE_CURVE('',#12565,#12566,#6970,.T.);
#15982=EDGE_CURVE('',#12565,#12567,#6971,.T.);
#15983=EDGE_CURVE('',#12568,#12566,#6972,.T.);
#15984=EDGE_CURVE('',#12567,#12568,#6973,.T.);
#15985=EDGE_CURVE('',#12567,#12569,#6974,.T.);
#15986=EDGE_CURVE('',#12570,#12568,#6975,.T.);
#15987=EDGE_CURVE('',#12569,#12570,#6976,.T.);
#15988=EDGE_CURVE('',#12569,#12571,#6977,.T.);
#15989=EDGE_CURVE('',#12572,#12570,#6978,.T.);
#15990=EDGE_CURVE('',#12571,#12572,#6979,.T.);
#15991=EDGE_CURVE('',#12571,#12573,#6980,.T.);
#15992=EDGE_CURVE('',#12574,#12572,#6981,.T.);
#15993=EDGE_CURVE('',#12573,#12574,#6982,.T.);
#15994=EDGE_CURVE('',#12573,#12575,#6983,.T.);
#15995=EDGE_CURVE('',#12576,#12574,#6984,.T.);
#15996=EDGE_CURVE('',#12575,#12576,#6985,.T.);
#15997=EDGE_CURVE('',#12575,#12577,#6986,.T.);
#15998=EDGE_CURVE('',#12578,#12576,#6987,.T.);
#15999=EDGE_CURVE('',#12577,#12578,#6988,.T.);
#16000=EDGE_CURVE('',#12577,#11997,#6989,.T.);
#16001=EDGE_CURVE('',#11990,#12578,#6990,.T.);
#20474=ORIENTED_EDGE('',*,*,#15098,.T.);
#20475=ORIENTED_EDGE('',*,*,#15099,.T.);
#20476=ORIENTED_EDGE('',*,*,#15100,.T.);
#20477=ORIENTED_EDGE('',*,*,#15101,.T.);
#20478=ORIENTED_EDGE('',*,*,#15102,.T.);
#20479=ORIENTED_EDGE('',*,*,#15103,.T.);
#20480=ORIENTED_EDGE('',*,*,#15100,.F.);
#20481=ORIENTED_EDGE('',*,*,#15104,.T.);
#20482=ORIENTED_EDGE('',*,*,#15105,.T.);
#20483=ORIENTED_EDGE('',*,*,#15106,.T.);
#20484=ORIENTED_EDGE('',*,*,#15102,.F.);
#20485=ORIENTED_EDGE('',*,*,#15107,.T.);
#20486=ORIENTED_EDGE('',*,*,#15108,.T.);
#20487=ORIENTED_EDGE('',*,*,#15109,.T.);
#20488=ORIENTED_EDGE('',*,*,#15105,.F.);
#20489=ORIENTED_EDGE('',*,*,#15110,.T.);
#20490=ORIENTED_EDGE('',*,*,#15111,.T.);
#20491=ORIENTED_EDGE('',*,*,#15112,.T.);
#20492=ORIENTED_EDGE('',*,*,#15108,.F.);
#20493=ORIENTED_EDGE('',*,*,#15113,.T.);
#20494=ORIENTED_EDGE('',*,*,#15113,.F.);
#20495=ORIENTED_EDGE('',*,*,#15114,.F.);
#20496=ORIENTED_EDGE('',*,*,#15115,.F.);
#20497=ORIENTED_EDGE('',*,*,#15116,.T.);
#20498=ORIENTED_EDGE('',*,*,#15110,.F.);
#20499=ORIENTED_EDGE('',*,*,#15117,.F.);
#20500=ORIENTED_EDGE('',*,*,#15118,.F.);
#20501=ORIENTED_EDGE('',*,*,#15114,.T.);
#20502=ORIENTED_EDGE('',*,*,#15107,.F.);
#20503=ORIENTED_EDGE('',*,*,#15119,.F.);
#20504=ORIENTED_EDGE('',*,*,#15120,.F.);
#20505=ORIENTED_EDGE('',*,*,#15117,.T.);
#20506=ORIENTED_EDGE('',*,*,#15104,.F.);
#20507=ORIENTED_EDGE('',*,*,#15121,.F.);
#20508=ORIENTED_EDGE('',*,*,#15122,.F.);
#20509=ORIENTED_EDGE('',*,*,#15119,.T.);
#20510=ORIENTED_EDGE('',*,*,#15099,.F.);
#20511=ORIENTED_EDGE('',*,*,#15123,.F.);
#20512=ORIENTED_EDGE('',*,*,#15124,.F.);
#20513=ORIENTED_EDGE('',*,*,#15121,.T.);
#20514=ORIENTED_EDGE('',*,*,#15125,.T.);
#20515=ORIENTED_EDGE('',*,*,#15115,.T.);
#20516=ORIENTED_EDGE('',*,*,#15126,.T.);
#20517=ORIENTED_EDGE('',*,*,#15127,.T.);
#20518=ORIENTED_EDGE('',*,*,#15126,.F.);
#20519=ORIENTED_EDGE('',*,*,#15118,.T.);
#20520=ORIENTED_EDGE('',*,*,#15128,.T.);
#20521=ORIENTED_EDGE('',*,*,#15129,.T.);
#20522=ORIENTED_EDGE('',*,*,#15130,.T.);
#20523=ORIENTED_EDGE('',*,*,#15131,.T.);
#20524=ORIENTED_EDGE('',*,*,#15128,.F.);
#20525=ORIENTED_EDGE('',*,*,#15120,.T.);
#20526=ORIENTED_EDGE('',*,*,#15130,.F.);
#20527=ORIENTED_EDGE('',*,*,#15122,.T.);
#20528=ORIENTED_EDGE('',*,*,#15132,.T.);
#20529=ORIENTED_EDGE('',*,*,#15133,.T.);
#20530=ORIENTED_EDGE('',*,*,#15134,.T.);
#20531=ORIENTED_EDGE('',*,*,#15135,.T.);
#20532=ORIENTED_EDGE('',*,*,#15132,.F.);
#20533=ORIENTED_EDGE('',*,*,#15124,.T.);
#20534=ORIENTED_EDGE('',*,*,#15136,.F.);
#20535=ORIENTED_EDGE('',*,*,#15137,.T.);
#20536=ORIENTED_EDGE('',*,*,#15138,.F.);
#20537=ORIENTED_EDGE('',*,*,#15137,.F.);
#20538=ORIENTED_EDGE('',*,*,#15139,.F.);
#20539=ORIENTED_EDGE('',*,*,#15140,.T.);
#20540=ORIENTED_EDGE('',*,*,#15141,.F.);
#20541=ORIENTED_EDGE('',*,*,#15140,.F.);
#20542=ORIENTED_EDGE('',*,*,#15142,.F.);
#20543=ORIENTED_EDGE('',*,*,#15143,.T.);
#20544=ORIENTED_EDGE('',*,*,#15144,.F.);
#20545=ORIENTED_EDGE('',*,*,#15143,.F.);
#20546=ORIENTED_EDGE('',*,*,#15145,.F.);
#20547=ORIENTED_EDGE('',*,*,#15146,.T.);
#20548=ORIENTED_EDGE('',*,*,#15147,.F.);
#20549=ORIENTED_EDGE('',*,*,#15146,.F.);
#20550=ORIENTED_EDGE('',*,*,#15148,.F.);
#20551=ORIENTED_EDGE('',*,*,#15149,.T.);
#20552=ORIENTED_EDGE('',*,*,#15150,.F.);
#20553=ORIENTED_EDGE('',*,*,#15149,.F.);
#20554=ORIENTED_EDGE('',*,*,#15151,.F.);
#20555=ORIENTED_EDGE('',*,*,#15152,.T.);
#20556=ORIENTED_EDGE('',*,*,#15153,.F.);
#20557=ORIENTED_EDGE('',*,*,#15152,.F.);
#20558=ORIENTED_EDGE('',*,*,#15154,.F.);
#20559=ORIENTED_EDGE('',*,*,#15155,.T.);
#20560=ORIENTED_EDGE('',*,*,#15156,.F.);
#20561=ORIENTED_EDGE('',*,*,#15155,.F.);
#20562=ORIENTED_EDGE('',*,*,#15157,.F.);
#20563=ORIENTED_EDGE('',*,*,#15158,.T.);
#20564=ORIENTED_EDGE('',*,*,#15159,.F.);
#20565=ORIENTED_EDGE('',*,*,#15158,.F.);
#20566=ORIENTED_EDGE('',*,*,#15160,.F.);
#20567=ORIENTED_EDGE('',*,*,#15161,.T.);
#20568=ORIENTED_EDGE('',*,*,#15162,.F.);
#20569=ORIENTED_EDGE('',*,*,#15161,.F.);
#20570=ORIENTED_EDGE('',*,*,#15163,.F.);
#20571=ORIENTED_EDGE('',*,*,#15164,.T.);
#20572=ORIENTED_EDGE('',*,*,#15165,.F.);
#20573=ORIENTED_EDGE('',*,*,#15164,.F.);
#20574=ORIENTED_EDGE('',*,*,#15166,.F.);
#20575=ORIENTED_EDGE('',*,*,#15134,.F.);
#20576=ORIENTED_EDGE('',*,*,#15123,.T.);
#20577=ORIENTED_EDGE('',*,*,#15098,.F.);
#20578=ORIENTED_EDGE('',*,*,#15167,.F.);
#20579=ORIENTED_EDGE('',*,*,#15168,.F.);
#20580=ORIENTED_EDGE('',*,*,#15169,.F.);
#20581=ORIENTED_EDGE('',*,*,#15168,.T.);
#20582=ORIENTED_EDGE('',*,*,#15170,.F.);
#20583=ORIENTED_EDGE('',*,*,#15171,.F.);
#20584=ORIENTED_EDGE('',*,*,#15172,.F.);
#20585=ORIENTED_EDGE('',*,*,#15171,.T.);
#20586=ORIENTED_EDGE('',*,*,#15173,.F.);
#20587=ORIENTED_EDGE('',*,*,#15174,.F.);
#20588=ORIENTED_EDGE('',*,*,#15175,.F.);
#20589=ORIENTED_EDGE('',*,*,#15174,.T.);
#20590=ORIENTED_EDGE('',*,*,#15176,.F.);
#20591=ORIENTED_EDGE('',*,*,#15177,.F.);
#20592=ORIENTED_EDGE('',*,*,#15178,.F.);
#20593=ORIENTED_EDGE('',*,*,#15177,.T.);
#20594=ORIENTED_EDGE('',*,*,#15179,.F.);
#20595=ORIENTED_EDGE('',*,*,#15180,.F.);
#20596=ORIENTED_EDGE('',*,*,#15181,.F.);
#20597=ORIENTED_EDGE('',*,*,#15180,.T.);
#20598=ORIENTED_EDGE('',*,*,#15182,.F.);
#20599=ORIENTED_EDGE('',*,*,#15183,.F.);
#20600=ORIENTED_EDGE('',*,*,#15184,.F.);
#20601=ORIENTED_EDGE('',*,*,#15183,.T.);
#20602=ORIENTED_EDGE('',*,*,#15185,.F.);
#20603=ORIENTED_EDGE('',*,*,#15186,.F.);
#20604=ORIENTED_EDGE('',*,*,#15187,.F.);
#20605=ORIENTED_EDGE('',*,*,#15186,.T.);
#20606=ORIENTED_EDGE('',*,*,#15188,.F.);
#20607=ORIENTED_EDGE('',*,*,#15189,.F.);
#20608=ORIENTED_EDGE('',*,*,#15190,.F.);
#20609=ORIENTED_EDGE('',*,*,#15189,.T.);
#20610=ORIENTED_EDGE('',*,*,#15191,.F.);
#20611=ORIENTED_EDGE('',*,*,#15192,.F.);
#20612=ORIENTED_EDGE('',*,*,#15193,.F.);
#20613=ORIENTED_EDGE('',*,*,#15192,.T.);
#20614=ORIENTED_EDGE('',*,*,#15194,.F.);
#20615=ORIENTED_EDGE('',*,*,#15195,.F.);
#20616=ORIENTED_EDGE('',*,*,#15196,.F.);
#20617=ORIENTED_EDGE('',*,*,#15195,.T.);
#20618=ORIENTED_EDGE('',*,*,#15197,.F.);
#20619=ORIENTED_EDGE('',*,*,#15198,.F.);
#20620=ORIENTED_EDGE('',*,*,#15199,.F.);
#20621=ORIENTED_EDGE('',*,*,#15198,.T.);
#20622=ORIENTED_EDGE('',*,*,#15200,.F.);
#20623=ORIENTED_EDGE('',*,*,#15201,.F.);
#20624=ORIENTED_EDGE('',*,*,#15202,.F.);
#20625=ORIENTED_EDGE('',*,*,#15201,.T.);
#20626=ORIENTED_EDGE('',*,*,#15203,.F.);
#20627=ORIENTED_EDGE('',*,*,#15204,.F.);
#20628=ORIENTED_EDGE('',*,*,#15205,.F.);
#20629=ORIENTED_EDGE('',*,*,#15204,.T.);
#20630=ORIENTED_EDGE('',*,*,#15206,.F.);
#20631=ORIENTED_EDGE('',*,*,#15207,.F.);
#20632=ORIENTED_EDGE('',*,*,#15208,.F.);
#20633=ORIENTED_EDGE('',*,*,#15207,.T.);
#20634=ORIENTED_EDGE('',*,*,#15209,.F.);
#20635=ORIENTED_EDGE('',*,*,#15210,.F.);
#20636=ORIENTED_EDGE('',*,*,#15211,.F.);
#20637=ORIENTED_EDGE('',*,*,#15210,.T.);
#20638=ORIENTED_EDGE('',*,*,#15212,.F.);
#20639=ORIENTED_EDGE('',*,*,#15213,.F.);
#20640=ORIENTED_EDGE('',*,*,#15214,.F.);
#20641=ORIENTED_EDGE('',*,*,#15213,.T.);
#20642=ORIENTED_EDGE('',*,*,#15215,.F.);
#20643=ORIENTED_EDGE('',*,*,#15216,.F.);
#20644=ORIENTED_EDGE('',*,*,#15217,.F.);
#20645=ORIENTED_EDGE('',*,*,#15216,.T.);
#20646=ORIENTED_EDGE('',*,*,#15218,.F.);
#20647=ORIENTED_EDGE('',*,*,#15219,.F.);
#20648=ORIENTED_EDGE('',*,*,#15220,.F.);
#20649=ORIENTED_EDGE('',*,*,#15219,.T.);
#20650=ORIENTED_EDGE('',*,*,#15221,.F.);
#20651=ORIENTED_EDGE('',*,*,#15222,.F.);
#20652=ORIENTED_EDGE('',*,*,#15223,.F.);
#20653=ORIENTED_EDGE('',*,*,#15222,.T.);
#20654=ORIENTED_EDGE('',*,*,#15224,.F.);
#20655=ORIENTED_EDGE('',*,*,#15225,.F.);
#20656=ORIENTED_EDGE('',*,*,#15226,.F.);
#20657=ORIENTED_EDGE('',*,*,#15225,.T.);
#20658=ORIENTED_EDGE('',*,*,#15227,.F.);
#20659=ORIENTED_EDGE('',*,*,#15228,.F.);
#20660=ORIENTED_EDGE('',*,*,#15229,.F.);
#20661=ORIENTED_EDGE('',*,*,#15228,.T.);
#20662=ORIENTED_EDGE('',*,*,#15230,.F.);
#20663=ORIENTED_EDGE('',*,*,#15231,.F.);
#20664=ORIENTED_EDGE('',*,*,#15232,.F.);
#20665=ORIENTED_EDGE('',*,*,#15231,.T.);
#20666=ORIENTED_EDGE('',*,*,#15233,.F.);
#20667=ORIENTED_EDGE('',*,*,#15234,.F.);
#20668=ORIENTED_EDGE('',*,*,#15235,.F.);
#20669=ORIENTED_EDGE('',*,*,#15234,.T.);
#20670=ORIENTED_EDGE('',*,*,#15236,.F.);
#20671=ORIENTED_EDGE('',*,*,#15237,.F.);
#20672=ORIENTED_EDGE('',*,*,#15238,.F.);
#20673=ORIENTED_EDGE('',*,*,#15237,.T.);
#20674=ORIENTED_EDGE('',*,*,#15239,.F.);
#20675=ORIENTED_EDGE('',*,*,#15240,.F.);
#20676=ORIENTED_EDGE('',*,*,#15241,.F.);
#20677=ORIENTED_EDGE('',*,*,#15240,.T.);
#20678=ORIENTED_EDGE('',*,*,#15242,.F.);
#20679=ORIENTED_EDGE('',*,*,#15243,.F.);
#20680=ORIENTED_EDGE('',*,*,#15244,.F.);
#20681=ORIENTED_EDGE('',*,*,#15243,.T.);
#20682=ORIENTED_EDGE('',*,*,#15245,.F.);
#20683=ORIENTED_EDGE('',*,*,#15246,.F.);
#20684=ORIENTED_EDGE('',*,*,#15247,.F.);
#20685=ORIENTED_EDGE('',*,*,#15246,.T.);
#20686=ORIENTED_EDGE('',*,*,#15248,.F.);
#20687=ORIENTED_EDGE('',*,*,#15249,.F.);
#20688=ORIENTED_EDGE('',*,*,#15250,.F.);
#20689=ORIENTED_EDGE('',*,*,#15249,.T.);
#20690=ORIENTED_EDGE('',*,*,#15251,.F.);
#20691=ORIENTED_EDGE('',*,*,#15252,.F.);
#20692=ORIENTED_EDGE('',*,*,#15253,.F.);
#20693=ORIENTED_EDGE('',*,*,#15252,.T.);
#20694=ORIENTED_EDGE('',*,*,#15254,.F.);
#20695=ORIENTED_EDGE('',*,*,#15255,.F.);
#20696=ORIENTED_EDGE('',*,*,#15256,.F.);
#20697=ORIENTED_EDGE('',*,*,#15255,.T.);
#20698=ORIENTED_EDGE('',*,*,#15257,.F.);
#20699=ORIENTED_EDGE('',*,*,#15258,.F.);
#20700=ORIENTED_EDGE('',*,*,#15259,.F.);
#20701=ORIENTED_EDGE('',*,*,#15258,.T.);
#20702=ORIENTED_EDGE('',*,*,#15260,.F.);
#20703=ORIENTED_EDGE('',*,*,#15261,.F.);
#20704=ORIENTED_EDGE('',*,*,#15262,.F.);
#20705=ORIENTED_EDGE('',*,*,#15261,.T.);
#20706=ORIENTED_EDGE('',*,*,#15263,.F.);
#20707=ORIENTED_EDGE('',*,*,#15264,.F.);
#20708=ORIENTED_EDGE('',*,*,#15265,.F.);
#20709=ORIENTED_EDGE('',*,*,#15264,.T.);
#20710=ORIENTED_EDGE('',*,*,#15266,.F.);
#20711=ORIENTED_EDGE('',*,*,#15267,.F.);
#20712=ORIENTED_EDGE('',*,*,#15268,.F.);
#20713=ORIENTED_EDGE('',*,*,#15267,.T.);
#20714=ORIENTED_EDGE('',*,*,#15269,.F.);
#20715=ORIENTED_EDGE('',*,*,#15270,.F.);
#20716=ORIENTED_EDGE('',*,*,#15271,.F.);
#20717=ORIENTED_EDGE('',*,*,#15270,.T.);
#20718=ORIENTED_EDGE('',*,*,#15272,.F.);
#20719=ORIENTED_EDGE('',*,*,#15273,.F.);
#20720=ORIENTED_EDGE('',*,*,#15274,.F.);
#20721=ORIENTED_EDGE('',*,*,#15273,.T.);
#20722=ORIENTED_EDGE('',*,*,#15275,.F.);
#20723=ORIENTED_EDGE('',*,*,#15276,.F.);
#20724=ORIENTED_EDGE('',*,*,#15277,.F.);
#20725=ORIENTED_EDGE('',*,*,#15276,.T.);
#20726=ORIENTED_EDGE('',*,*,#15278,.F.);
#20727=ORIENTED_EDGE('',*,*,#15279,.F.);
#20728=ORIENTED_EDGE('',*,*,#15280,.F.);
#20729=ORIENTED_EDGE('',*,*,#15279,.T.);
#20730=ORIENTED_EDGE('',*,*,#15281,.F.);
#20731=ORIENTED_EDGE('',*,*,#15282,.F.);
#20732=ORIENTED_EDGE('',*,*,#15283,.F.);
#20733=ORIENTED_EDGE('',*,*,#15282,.T.);
#20734=ORIENTED_EDGE('',*,*,#15284,.F.);
#20735=ORIENTED_EDGE('',*,*,#15285,.F.);
#20736=ORIENTED_EDGE('',*,*,#15286,.F.);
#20737=ORIENTED_EDGE('',*,*,#15285,.T.);
#20738=ORIENTED_EDGE('',*,*,#15287,.F.);
#20739=ORIENTED_EDGE('',*,*,#15288,.F.);
#20740=ORIENTED_EDGE('',*,*,#15289,.F.);
#20741=ORIENTED_EDGE('',*,*,#15288,.T.);
#20742=ORIENTED_EDGE('',*,*,#15290,.F.);
#20743=ORIENTED_EDGE('',*,*,#15291,.F.);
#20744=ORIENTED_EDGE('',*,*,#15292,.F.);
#20745=ORIENTED_EDGE('',*,*,#15291,.T.);
#20746=ORIENTED_EDGE('',*,*,#15293,.F.);
#20747=ORIENTED_EDGE('',*,*,#15294,.F.);
#20748=ORIENTED_EDGE('',*,*,#15295,.F.);
#20749=ORIENTED_EDGE('',*,*,#15294,.T.);
#20750=ORIENTED_EDGE('',*,*,#15296,.F.);
#20751=ORIENTED_EDGE('',*,*,#15297,.F.);
#20752=ORIENTED_EDGE('',*,*,#15298,.F.);
#20753=ORIENTED_EDGE('',*,*,#15297,.T.);
#20754=ORIENTED_EDGE('',*,*,#15299,.F.);
#20755=ORIENTED_EDGE('',*,*,#15300,.F.);
#20756=ORIENTED_EDGE('',*,*,#15301,.F.);
#20757=ORIENTED_EDGE('',*,*,#15300,.T.);
#20758=ORIENTED_EDGE('',*,*,#15302,.F.);
#20759=ORIENTED_EDGE('',*,*,#15303,.F.);
#20760=ORIENTED_EDGE('',*,*,#15304,.F.);
#20761=ORIENTED_EDGE('',*,*,#15303,.T.);
#20762=ORIENTED_EDGE('',*,*,#15305,.F.);
#20763=ORIENTED_EDGE('',*,*,#15306,.F.);
#20764=ORIENTED_EDGE('',*,*,#15307,.F.);
#20765=ORIENTED_EDGE('',*,*,#15306,.T.);
#20766=ORIENTED_EDGE('',*,*,#15308,.F.);
#20767=ORIENTED_EDGE('',*,*,#15309,.F.);
#20768=ORIENTED_EDGE('',*,*,#15310,.F.);
#20769=ORIENTED_EDGE('',*,*,#15309,.T.);
#20770=ORIENTED_EDGE('',*,*,#15311,.F.);
#20771=ORIENTED_EDGE('',*,*,#15312,.F.);
#20772=ORIENTED_EDGE('',*,*,#15313,.F.);
#20773=ORIENTED_EDGE('',*,*,#15312,.T.);
#20774=ORIENTED_EDGE('',*,*,#15314,.F.);
#20775=ORIENTED_EDGE('',*,*,#15315,.F.);
#20776=ORIENTED_EDGE('',*,*,#15316,.F.);
#20777=ORIENTED_EDGE('',*,*,#15315,.T.);
#20778=ORIENTED_EDGE('',*,*,#15317,.F.);
#20779=ORIENTED_EDGE('',*,*,#15318,.F.);
#20780=ORIENTED_EDGE('',*,*,#15319,.F.);
#20781=ORIENTED_EDGE('',*,*,#15318,.T.);
#20782=ORIENTED_EDGE('',*,*,#15320,.F.);
#20783=ORIENTED_EDGE('',*,*,#15321,.F.);
#20784=ORIENTED_EDGE('',*,*,#15322,.F.);
#20785=ORIENTED_EDGE('',*,*,#15321,.T.);
#20786=ORIENTED_EDGE('',*,*,#15323,.F.);
#20787=ORIENTED_EDGE('',*,*,#15324,.F.);
#20788=ORIENTED_EDGE('',*,*,#15325,.F.);
#20789=ORIENTED_EDGE('',*,*,#15324,.T.);
#20790=ORIENTED_EDGE('',*,*,#15326,.F.);
#20791=ORIENTED_EDGE('',*,*,#15327,.F.);
#20792=ORIENTED_EDGE('',*,*,#15328,.F.);
#20793=ORIENTED_EDGE('',*,*,#15327,.T.);
#20794=ORIENTED_EDGE('',*,*,#15329,.F.);
#20795=ORIENTED_EDGE('',*,*,#15330,.F.);
#20796=ORIENTED_EDGE('',*,*,#15331,.F.);
#20797=ORIENTED_EDGE('',*,*,#15330,.T.);
#20798=ORIENTED_EDGE('',*,*,#15332,.F.);
#20799=ORIENTED_EDGE('',*,*,#15333,.F.);
#20800=ORIENTED_EDGE('',*,*,#15334,.F.);
#20801=ORIENTED_EDGE('',*,*,#15333,.T.);
#20802=ORIENTED_EDGE('',*,*,#15335,.F.);
#20803=ORIENTED_EDGE('',*,*,#15336,.F.);
#20804=ORIENTED_EDGE('',*,*,#15337,.F.);
#20805=ORIENTED_EDGE('',*,*,#15336,.T.);
#20806=ORIENTED_EDGE('',*,*,#15338,.F.);
#20807=ORIENTED_EDGE('',*,*,#15339,.F.);
#20808=ORIENTED_EDGE('',*,*,#15340,.F.);
#20809=ORIENTED_EDGE('',*,*,#15339,.T.);
#20810=ORIENTED_EDGE('',*,*,#15341,.F.);
#20811=ORIENTED_EDGE('',*,*,#15342,.F.);
#20812=ORIENTED_EDGE('',*,*,#15343,.F.);
#20813=ORIENTED_EDGE('',*,*,#15342,.T.);
#20814=ORIENTED_EDGE('',*,*,#15344,.F.);
#20815=ORIENTED_EDGE('',*,*,#15345,.F.);
#20816=ORIENTED_EDGE('',*,*,#15346,.F.);
#20817=ORIENTED_EDGE('',*,*,#15345,.T.);
#20818=ORIENTED_EDGE('',*,*,#15347,.F.);
#20819=ORIENTED_EDGE('',*,*,#15348,.F.);
#20820=ORIENTED_EDGE('',*,*,#15349,.F.);
#20821=ORIENTED_EDGE('',*,*,#15348,.T.);
#20822=ORIENTED_EDGE('',*,*,#15350,.F.);
#20823=ORIENTED_EDGE('',*,*,#15351,.F.);
#20824=ORIENTED_EDGE('',*,*,#15352,.F.);
#20825=ORIENTED_EDGE('',*,*,#15351,.T.);
#20826=ORIENTED_EDGE('',*,*,#15353,.F.);
#20827=ORIENTED_EDGE('',*,*,#15354,.F.);
#20828=ORIENTED_EDGE('',*,*,#15355,.F.);
#20829=ORIENTED_EDGE('',*,*,#15354,.T.);
#20830=ORIENTED_EDGE('',*,*,#15356,.F.);
#20831=ORIENTED_EDGE('',*,*,#15357,.F.);
#20832=ORIENTED_EDGE('',*,*,#15358,.F.);
#20833=ORIENTED_EDGE('',*,*,#15357,.T.);
#20834=ORIENTED_EDGE('',*,*,#15359,.F.);
#20835=ORIENTED_EDGE('',*,*,#15360,.F.);
#20836=ORIENTED_EDGE('',*,*,#15361,.F.);
#20837=ORIENTED_EDGE('',*,*,#15360,.T.);
#20838=ORIENTED_EDGE('',*,*,#15362,.F.);
#20839=ORIENTED_EDGE('',*,*,#15363,.F.);
#20840=ORIENTED_EDGE('',*,*,#15364,.F.);
#20841=ORIENTED_EDGE('',*,*,#15363,.T.);
#20842=ORIENTED_EDGE('',*,*,#15365,.F.);
#20843=ORIENTED_EDGE('',*,*,#15366,.F.);
#20844=ORIENTED_EDGE('',*,*,#15367,.F.);
#20845=ORIENTED_EDGE('',*,*,#15366,.T.);
#20846=ORIENTED_EDGE('',*,*,#15368,.F.);
#20847=ORIENTED_EDGE('',*,*,#15369,.F.);
#20848=ORIENTED_EDGE('',*,*,#15370,.F.);
#20849=ORIENTED_EDGE('',*,*,#15369,.T.);
#20850=ORIENTED_EDGE('',*,*,#15371,.F.);
#20851=ORIENTED_EDGE('',*,*,#15372,.F.);
#20852=ORIENTED_EDGE('',*,*,#15373,.F.);
#20853=ORIENTED_EDGE('',*,*,#15372,.T.);
#20854=ORIENTED_EDGE('',*,*,#15374,.F.);
#20855=ORIENTED_EDGE('',*,*,#15375,.F.);
#20856=ORIENTED_EDGE('',*,*,#15376,.F.);
#20857=ORIENTED_EDGE('',*,*,#15375,.T.);
#20858=ORIENTED_EDGE('',*,*,#15377,.F.);
#20859=ORIENTED_EDGE('',*,*,#15378,.F.);
#20860=ORIENTED_EDGE('',*,*,#15379,.F.);
#20861=ORIENTED_EDGE('',*,*,#15378,.T.);
#20862=ORIENTED_EDGE('',*,*,#15380,.F.);
#20863=ORIENTED_EDGE('',*,*,#15381,.F.);
#20864=ORIENTED_EDGE('',*,*,#15382,.F.);
#20865=ORIENTED_EDGE('',*,*,#15381,.T.);
#20866=ORIENTED_EDGE('',*,*,#15383,.F.);
#20867=ORIENTED_EDGE('',*,*,#15384,.F.);
#20868=ORIENTED_EDGE('',*,*,#15385,.F.);
#20869=ORIENTED_EDGE('',*,*,#15384,.T.);
#20870=ORIENTED_EDGE('',*,*,#15386,.F.);
#20871=ORIENTED_EDGE('',*,*,#15387,.F.);
#20872=ORIENTED_EDGE('',*,*,#15388,.F.);
#20873=ORIENTED_EDGE('',*,*,#15387,.T.);
#20874=ORIENTED_EDGE('',*,*,#15389,.F.);
#20875=ORIENTED_EDGE('',*,*,#15390,.F.);
#20876=ORIENTED_EDGE('',*,*,#15391,.F.);
#20877=ORIENTED_EDGE('',*,*,#15390,.T.);
#20878=ORIENTED_EDGE('',*,*,#15392,.F.);
#20879=ORIENTED_EDGE('',*,*,#15393,.F.);
#20880=ORIENTED_EDGE('',*,*,#15394,.F.);
#20881=ORIENTED_EDGE('',*,*,#15393,.T.);
#20882=ORIENTED_EDGE('',*,*,#15395,.F.);
#20883=ORIENTED_EDGE('',*,*,#15396,.F.);
#20884=ORIENTED_EDGE('',*,*,#15397,.F.);
#20885=ORIENTED_EDGE('',*,*,#15396,.T.);
#20886=ORIENTED_EDGE('',*,*,#15398,.F.);
#20887=ORIENTED_EDGE('',*,*,#15399,.F.);
#20888=ORIENTED_EDGE('',*,*,#15400,.F.);
#20889=ORIENTED_EDGE('',*,*,#15399,.T.);
#20890=ORIENTED_EDGE('',*,*,#15401,.F.);
#20891=ORIENTED_EDGE('',*,*,#15402,.F.);
#20892=ORIENTED_EDGE('',*,*,#15403,.F.);
#20893=ORIENTED_EDGE('',*,*,#15402,.T.);
#20894=ORIENTED_EDGE('',*,*,#15404,.F.);
#20895=ORIENTED_EDGE('',*,*,#15405,.F.);
#20896=ORIENTED_EDGE('',*,*,#15406,.F.);
#20897=ORIENTED_EDGE('',*,*,#15405,.T.);
#20898=ORIENTED_EDGE('',*,*,#15407,.F.);
#20899=ORIENTED_EDGE('',*,*,#15408,.F.);
#20900=ORIENTED_EDGE('',*,*,#15409,.F.);
#20901=ORIENTED_EDGE('',*,*,#15408,.T.);
#20902=ORIENTED_EDGE('',*,*,#15410,.F.);
#20903=ORIENTED_EDGE('',*,*,#15411,.F.);
#20904=ORIENTED_EDGE('',*,*,#15412,.F.);
#20905=ORIENTED_EDGE('',*,*,#15411,.T.);
#20906=ORIENTED_EDGE('',*,*,#15413,.F.);
#20907=ORIENTED_EDGE('',*,*,#15414,.F.);
#20908=ORIENTED_EDGE('',*,*,#15415,.F.);
#20909=ORIENTED_EDGE('',*,*,#15414,.T.);
#20910=ORIENTED_EDGE('',*,*,#15416,.F.);
#20911=ORIENTED_EDGE('',*,*,#15417,.F.);
#20912=ORIENTED_EDGE('',*,*,#15418,.F.);
#20913=ORIENTED_EDGE('',*,*,#15417,.T.);
#20914=ORIENTED_EDGE('',*,*,#15419,.F.);
#20915=ORIENTED_EDGE('',*,*,#15420,.F.);
#20916=ORIENTED_EDGE('',*,*,#15421,.F.);
#20917=ORIENTED_EDGE('',*,*,#15420,.T.);
#20918=ORIENTED_EDGE('',*,*,#15422,.F.);
#20919=ORIENTED_EDGE('',*,*,#15423,.F.);
#20920=ORIENTED_EDGE('',*,*,#15424,.F.);
#20921=ORIENTED_EDGE('',*,*,#15423,.T.);
#20922=ORIENTED_EDGE('',*,*,#15425,.F.);
#20923=ORIENTED_EDGE('',*,*,#15426,.F.);
#20924=ORIENTED_EDGE('',*,*,#15427,.F.);
#20925=ORIENTED_EDGE('',*,*,#15426,.T.);
#20926=ORIENTED_EDGE('',*,*,#15428,.F.);
#20927=ORIENTED_EDGE('',*,*,#15429,.F.);
#20928=ORIENTED_EDGE('',*,*,#15430,.F.);
#20929=ORIENTED_EDGE('',*,*,#15429,.T.);
#20930=ORIENTED_EDGE('',*,*,#15431,.F.);
#20931=ORIENTED_EDGE('',*,*,#15432,.F.);
#20932=ORIENTED_EDGE('',*,*,#15433,.F.);
#20933=ORIENTED_EDGE('',*,*,#15432,.T.);
#20934=ORIENTED_EDGE('',*,*,#15434,.F.);
#20935=ORIENTED_EDGE('',*,*,#15435,.F.);
#20936=ORIENTED_EDGE('',*,*,#15436,.F.);
#20937=ORIENTED_EDGE('',*,*,#15435,.T.);
#20938=ORIENTED_EDGE('',*,*,#15437,.F.);
#20939=ORIENTED_EDGE('',*,*,#15438,.F.);
#20940=ORIENTED_EDGE('',*,*,#15439,.F.);
#20941=ORIENTED_EDGE('',*,*,#15438,.T.);
#20942=ORIENTED_EDGE('',*,*,#15440,.F.);
#20943=ORIENTED_EDGE('',*,*,#15441,.F.);
#20944=ORIENTED_EDGE('',*,*,#15442,.F.);
#20945=ORIENTED_EDGE('',*,*,#15441,.T.);
#20946=ORIENTED_EDGE('',*,*,#15443,.F.);
#20947=ORIENTED_EDGE('',*,*,#15444,.F.);
#20948=ORIENTED_EDGE('',*,*,#15445,.F.);
#20949=ORIENTED_EDGE('',*,*,#15444,.T.);
#20950=ORIENTED_EDGE('',*,*,#15446,.F.);
#20951=ORIENTED_EDGE('',*,*,#15447,.F.);
#20952=ORIENTED_EDGE('',*,*,#15448,.F.);
#20953=ORIENTED_EDGE('',*,*,#15447,.T.);
#20954=ORIENTED_EDGE('',*,*,#15449,.F.);
#20955=ORIENTED_EDGE('',*,*,#15450,.F.);
#20956=ORIENTED_EDGE('',*,*,#15451,.F.);
#20957=ORIENTED_EDGE('',*,*,#15450,.T.);
#20958=ORIENTED_EDGE('',*,*,#15452,.F.);
#20959=ORIENTED_EDGE('',*,*,#15453,.F.);
#20960=ORIENTED_EDGE('',*,*,#15454,.F.);
#20961=ORIENTED_EDGE('',*,*,#15453,.T.);
#20962=ORIENTED_EDGE('',*,*,#15455,.F.);
#20963=ORIENTED_EDGE('',*,*,#15456,.F.);
#20964=ORIENTED_EDGE('',*,*,#15457,.F.);
#20965=ORIENTED_EDGE('',*,*,#15456,.T.);
#20966=ORIENTED_EDGE('',*,*,#15458,.F.);
#20967=ORIENTED_EDGE('',*,*,#15459,.F.);
#20968=ORIENTED_EDGE('',*,*,#15460,.F.);
#20969=ORIENTED_EDGE('',*,*,#15459,.T.);
#20970=ORIENTED_EDGE('',*,*,#15461,.F.);
#20971=ORIENTED_EDGE('',*,*,#15462,.F.);
#20972=ORIENTED_EDGE('',*,*,#15463,.F.);
#20973=ORIENTED_EDGE('',*,*,#15462,.T.);
#20974=ORIENTED_EDGE('',*,*,#15464,.F.);
#20975=ORIENTED_EDGE('',*,*,#15465,.F.);
#20976=ORIENTED_EDGE('',*,*,#15466,.F.);
#20977=ORIENTED_EDGE('',*,*,#15465,.T.);
#20978=ORIENTED_EDGE('',*,*,#15467,.F.);
#20979=ORIENTED_EDGE('',*,*,#15468,.F.);
#20980=ORIENTED_EDGE('',*,*,#15469,.F.);
#20981=ORIENTED_EDGE('',*,*,#15468,.T.);
#20982=ORIENTED_EDGE('',*,*,#15470,.F.);
#20983=ORIENTED_EDGE('',*,*,#15471,.F.);
#20984=ORIENTED_EDGE('',*,*,#15472,.F.);
#20985=ORIENTED_EDGE('',*,*,#15471,.T.);
#20986=ORIENTED_EDGE('',*,*,#15473,.F.);
#20987=ORIENTED_EDGE('',*,*,#15474,.F.);
#20988=ORIENTED_EDGE('',*,*,#15475,.F.);
#20989=ORIENTED_EDGE('',*,*,#15474,.T.);
#20990=ORIENTED_EDGE('',*,*,#15476,.F.);
#20991=ORIENTED_EDGE('',*,*,#15477,.F.);
#20992=ORIENTED_EDGE('',*,*,#15478,.F.);
#20993=ORIENTED_EDGE('',*,*,#15477,.T.);
#20994=ORIENTED_EDGE('',*,*,#15479,.F.);
#20995=ORIENTED_EDGE('',*,*,#15480,.F.);
#20996=ORIENTED_EDGE('',*,*,#15481,.F.);
#20997=ORIENTED_EDGE('',*,*,#15480,.T.);
#20998=ORIENTED_EDGE('',*,*,#15482,.F.);
#20999=ORIENTED_EDGE('',*,*,#15483,.F.);
#21000=ORIENTED_EDGE('',*,*,#15484,.F.);
#21001=ORIENTED_EDGE('',*,*,#15483,.T.);
#21002=ORIENTED_EDGE('',*,*,#15485,.F.);
#21003=ORIENTED_EDGE('',*,*,#15486,.F.);
#21004=ORIENTED_EDGE('',*,*,#15487,.F.);
#21005=ORIENTED_EDGE('',*,*,#15486,.T.);
#21006=ORIENTED_EDGE('',*,*,#15488,.F.);
#21007=ORIENTED_EDGE('',*,*,#15489,.F.);
#21008=ORIENTED_EDGE('',*,*,#15490,.F.);
#21009=ORIENTED_EDGE('',*,*,#15489,.T.);
#21010=ORIENTED_EDGE('',*,*,#15491,.F.);
#21011=ORIENTED_EDGE('',*,*,#15492,.F.);
#21012=ORIENTED_EDGE('',*,*,#15493,.F.);
#21013=ORIENTED_EDGE('',*,*,#15492,.T.);
#21014=ORIENTED_EDGE('',*,*,#15494,.F.);
#21015=ORIENTED_EDGE('',*,*,#15495,.F.);
#21016=ORIENTED_EDGE('',*,*,#15496,.F.);
#21017=ORIENTED_EDGE('',*,*,#15495,.T.);
#21018=ORIENTED_EDGE('',*,*,#15497,.F.);
#21019=ORIENTED_EDGE('',*,*,#15498,.F.);
#21020=ORIENTED_EDGE('',*,*,#15499,.F.);
#21021=ORIENTED_EDGE('',*,*,#15498,.T.);
#21022=ORIENTED_EDGE('',*,*,#15500,.F.);
#21023=ORIENTED_EDGE('',*,*,#15501,.F.);
#21024=ORIENTED_EDGE('',*,*,#15502,.F.);
#21025=ORIENTED_EDGE('',*,*,#15501,.T.);
#21026=ORIENTED_EDGE('',*,*,#15503,.F.);
#21027=ORIENTED_EDGE('',*,*,#15504,.F.);
#21028=ORIENTED_EDGE('',*,*,#15505,.F.);
#21029=ORIENTED_EDGE('',*,*,#15504,.T.);
#21030=ORIENTED_EDGE('',*,*,#15506,.F.);
#21031=ORIENTED_EDGE('',*,*,#15507,.F.);
#21032=ORIENTED_EDGE('',*,*,#15508,.F.);
#21033=ORIENTED_EDGE('',*,*,#15507,.T.);
#21034=ORIENTED_EDGE('',*,*,#15509,.F.);
#21035=ORIENTED_EDGE('',*,*,#15510,.F.);
#21036=ORIENTED_EDGE('',*,*,#15511,.F.);
#21037=ORIENTED_EDGE('',*,*,#15510,.T.);
#21038=ORIENTED_EDGE('',*,*,#15512,.F.);
#21039=ORIENTED_EDGE('',*,*,#15513,.F.);
#21040=ORIENTED_EDGE('',*,*,#15514,.F.);
#21041=ORIENTED_EDGE('',*,*,#15513,.T.);
#21042=ORIENTED_EDGE('',*,*,#15515,.F.);
#21043=ORIENTED_EDGE('',*,*,#15516,.F.);
#21044=ORIENTED_EDGE('',*,*,#15517,.F.);
#21045=ORIENTED_EDGE('',*,*,#15516,.T.);
#21046=ORIENTED_EDGE('',*,*,#15518,.F.);
#21047=ORIENTED_EDGE('',*,*,#15519,.F.);
#21048=ORIENTED_EDGE('',*,*,#15520,.F.);
#21049=ORIENTED_EDGE('',*,*,#15519,.T.);
#21050=ORIENTED_EDGE('',*,*,#15521,.F.);
#21051=ORIENTED_EDGE('',*,*,#15522,.F.);
#21052=ORIENTED_EDGE('',*,*,#15523,.F.);
#21053=ORIENTED_EDGE('',*,*,#15522,.T.);
#21054=ORIENTED_EDGE('',*,*,#15524,.F.);
#21055=ORIENTED_EDGE('',*,*,#15525,.F.);
#21056=ORIENTED_EDGE('',*,*,#15526,.F.);
#21057=ORIENTED_EDGE('',*,*,#15525,.T.);
#21058=ORIENTED_EDGE('',*,*,#15527,.F.);
#21059=ORIENTED_EDGE('',*,*,#15528,.F.);
#21060=ORIENTED_EDGE('',*,*,#15529,.F.);
#21061=ORIENTED_EDGE('',*,*,#15528,.T.);
#21062=ORIENTED_EDGE('',*,*,#15530,.F.);
#21063=ORIENTED_EDGE('',*,*,#15531,.F.);
#21064=ORIENTED_EDGE('',*,*,#15532,.F.);
#21065=ORIENTED_EDGE('',*,*,#15531,.T.);
#21066=ORIENTED_EDGE('',*,*,#15533,.F.);
#21067=ORIENTED_EDGE('',*,*,#15534,.F.);
#21068=ORIENTED_EDGE('',*,*,#15535,.F.);
#21069=ORIENTED_EDGE('',*,*,#15534,.T.);
#21070=ORIENTED_EDGE('',*,*,#15536,.F.);
#21071=ORIENTED_EDGE('',*,*,#15537,.F.);
#21072=ORIENTED_EDGE('',*,*,#15538,.F.);
#21073=ORIENTED_EDGE('',*,*,#15537,.T.);
#21074=ORIENTED_EDGE('',*,*,#15539,.F.);
#21075=ORIENTED_EDGE('',*,*,#15540,.F.);
#21076=ORIENTED_EDGE('',*,*,#15541,.F.);
#21077=ORIENTED_EDGE('',*,*,#15540,.T.);
#21078=ORIENTED_EDGE('',*,*,#15542,.F.);
#21079=ORIENTED_EDGE('',*,*,#15543,.F.);
#21080=ORIENTED_EDGE('',*,*,#15544,.F.);
#21081=ORIENTED_EDGE('',*,*,#15543,.T.);
#21082=ORIENTED_EDGE('',*,*,#15545,.F.);
#21083=ORIENTED_EDGE('',*,*,#15546,.F.);
#21084=ORIENTED_EDGE('',*,*,#15547,.F.);
#21085=ORIENTED_EDGE('',*,*,#15546,.T.);
#21086=ORIENTED_EDGE('',*,*,#15548,.F.);
#21087=ORIENTED_EDGE('',*,*,#15549,.F.);
#21088=ORIENTED_EDGE('',*,*,#15550,.F.);
#21089=ORIENTED_EDGE('',*,*,#15549,.T.);
#21090=ORIENTED_EDGE('',*,*,#15551,.F.);
#21091=ORIENTED_EDGE('',*,*,#15552,.F.);
#21092=ORIENTED_EDGE('',*,*,#15553,.F.);
#21093=ORIENTED_EDGE('',*,*,#15552,.T.);
#21094=ORIENTED_EDGE('',*,*,#15554,.F.);
#21095=ORIENTED_EDGE('',*,*,#15555,.F.);
#21096=ORIENTED_EDGE('',*,*,#15556,.F.);
#21097=ORIENTED_EDGE('',*,*,#15555,.T.);
#21098=ORIENTED_EDGE('',*,*,#15557,.F.);
#21099=ORIENTED_EDGE('',*,*,#15558,.F.);
#21100=ORIENTED_EDGE('',*,*,#15559,.F.);
#21101=ORIENTED_EDGE('',*,*,#15558,.T.);
#21102=ORIENTED_EDGE('',*,*,#15560,.F.);
#21103=ORIENTED_EDGE('',*,*,#15561,.F.);
#21104=ORIENTED_EDGE('',*,*,#15562,.F.);
#21105=ORIENTED_EDGE('',*,*,#15561,.T.);
#21106=ORIENTED_EDGE('',*,*,#15563,.F.);
#21107=ORIENTED_EDGE('',*,*,#15564,.F.);
#21108=ORIENTED_EDGE('',*,*,#15565,.F.);
#21109=ORIENTED_EDGE('',*,*,#15564,.T.);
#21110=ORIENTED_EDGE('',*,*,#15566,.F.);
#21111=ORIENTED_EDGE('',*,*,#15567,.F.);
#21112=ORIENTED_EDGE('',*,*,#15568,.F.);
#21113=ORIENTED_EDGE('',*,*,#15567,.T.);
#21114=ORIENTED_EDGE('',*,*,#15569,.F.);
#21115=ORIENTED_EDGE('',*,*,#15570,.F.);
#21116=ORIENTED_EDGE('',*,*,#15571,.F.);
#21117=ORIENTED_EDGE('',*,*,#15570,.T.);
#21118=ORIENTED_EDGE('',*,*,#15572,.F.);
#21119=ORIENTED_EDGE('',*,*,#15573,.F.);
#21120=ORIENTED_EDGE('',*,*,#15574,.F.);
#21121=ORIENTED_EDGE('',*,*,#15573,.T.);
#21122=ORIENTED_EDGE('',*,*,#15575,.F.);
#21123=ORIENTED_EDGE('',*,*,#15576,.F.);
#21124=ORIENTED_EDGE('',*,*,#15577,.F.);
#21125=ORIENTED_EDGE('',*,*,#15576,.T.);
#21126=ORIENTED_EDGE('',*,*,#15578,.F.);
#21127=ORIENTED_EDGE('',*,*,#15579,.F.);
#21128=ORIENTED_EDGE('',*,*,#15580,.F.);
#21129=ORIENTED_EDGE('',*,*,#15579,.T.);
#21130=ORIENTED_EDGE('',*,*,#15581,.F.);
#21131=ORIENTED_EDGE('',*,*,#15582,.F.);
#21132=ORIENTED_EDGE('',*,*,#15583,.F.);
#21133=ORIENTED_EDGE('',*,*,#15582,.T.);
#21134=ORIENTED_EDGE('',*,*,#15584,.F.);
#21135=ORIENTED_EDGE('',*,*,#15585,.F.);
#21136=ORIENTED_EDGE('',*,*,#15586,.F.);
#21137=ORIENTED_EDGE('',*,*,#15585,.T.);
#21138=ORIENTED_EDGE('',*,*,#15587,.F.);
#21139=ORIENTED_EDGE('',*,*,#15588,.F.);
#21140=ORIENTED_EDGE('',*,*,#15589,.F.);
#21141=ORIENTED_EDGE('',*,*,#15588,.T.);
#21142=ORIENTED_EDGE('',*,*,#15590,.F.);
#21143=ORIENTED_EDGE('',*,*,#15591,.F.);
#21144=ORIENTED_EDGE('',*,*,#15592,.F.);
#21145=ORIENTED_EDGE('',*,*,#15591,.T.);
#21146=ORIENTED_EDGE('',*,*,#15593,.F.);
#21147=ORIENTED_EDGE('',*,*,#15594,.F.);
#21148=ORIENTED_EDGE('',*,*,#15595,.F.);
#21149=ORIENTED_EDGE('',*,*,#15594,.T.);
#21150=ORIENTED_EDGE('',*,*,#15596,.F.);
#21151=ORIENTED_EDGE('',*,*,#15597,.F.);
#21152=ORIENTED_EDGE('',*,*,#15598,.F.);
#21153=ORIENTED_EDGE('',*,*,#15597,.T.);
#21154=ORIENTED_EDGE('',*,*,#15599,.F.);
#21155=ORIENTED_EDGE('',*,*,#15600,.F.);
#21156=ORIENTED_EDGE('',*,*,#15601,.F.);
#21157=ORIENTED_EDGE('',*,*,#15600,.T.);
#21158=ORIENTED_EDGE('',*,*,#15602,.F.);
#21159=ORIENTED_EDGE('',*,*,#15603,.F.);
#21160=ORIENTED_EDGE('',*,*,#15604,.F.);
#21161=ORIENTED_EDGE('',*,*,#15603,.T.);
#21162=ORIENTED_EDGE('',*,*,#15605,.F.);
#21163=ORIENTED_EDGE('',*,*,#15606,.F.);
#21164=ORIENTED_EDGE('',*,*,#15607,.F.);
#21165=ORIENTED_EDGE('',*,*,#15606,.T.);
#21166=ORIENTED_EDGE('',*,*,#15608,.F.);
#21167=ORIENTED_EDGE('',*,*,#15609,.F.);
#21168=ORIENTED_EDGE('',*,*,#15610,.F.);
#21169=ORIENTED_EDGE('',*,*,#15609,.T.);
#21170=ORIENTED_EDGE('',*,*,#15611,.F.);
#21171=ORIENTED_EDGE('',*,*,#15612,.F.);
#21172=ORIENTED_EDGE('',*,*,#15613,.F.);
#21173=ORIENTED_EDGE('',*,*,#15612,.T.);
#21174=ORIENTED_EDGE('',*,*,#15614,.F.);
#21175=ORIENTED_EDGE('',*,*,#15615,.F.);
#21176=ORIENTED_EDGE('',*,*,#15616,.F.);
#21177=ORIENTED_EDGE('',*,*,#15615,.T.);
#21178=ORIENTED_EDGE('',*,*,#15617,.F.);
#21179=ORIENTED_EDGE('',*,*,#15618,.F.);
#21180=ORIENTED_EDGE('',*,*,#15619,.F.);
#21181=ORIENTED_EDGE('',*,*,#15618,.T.);
#21182=ORIENTED_EDGE('',*,*,#15620,.F.);
#21183=ORIENTED_EDGE('',*,*,#15621,.F.);
#21184=ORIENTED_EDGE('',*,*,#15622,.F.);
#21185=ORIENTED_EDGE('',*,*,#15621,.T.);
#21186=ORIENTED_EDGE('',*,*,#15623,.F.);
#21187=ORIENTED_EDGE('',*,*,#15624,.F.);
#21188=ORIENTED_EDGE('',*,*,#15625,.F.);
#21189=ORIENTED_EDGE('',*,*,#15624,.T.);
#21190=ORIENTED_EDGE('',*,*,#15626,.F.);
#21191=ORIENTED_EDGE('',*,*,#15627,.F.);
#21192=ORIENTED_EDGE('',*,*,#15628,.F.);
#21193=ORIENTED_EDGE('',*,*,#15627,.T.);
#21194=ORIENTED_EDGE('',*,*,#15629,.F.);
#21195=ORIENTED_EDGE('',*,*,#15630,.F.);
#21196=ORIENTED_EDGE('',*,*,#15631,.F.);
#21197=ORIENTED_EDGE('',*,*,#15630,.T.);
#21198=ORIENTED_EDGE('',*,*,#15632,.F.);
#21199=ORIENTED_EDGE('',*,*,#15633,.F.);
#21200=ORIENTED_EDGE('',*,*,#15634,.F.);
#21201=ORIENTED_EDGE('',*,*,#15633,.T.);
#21202=ORIENTED_EDGE('',*,*,#15635,.F.);
#21203=ORIENTED_EDGE('',*,*,#15636,.F.);
#21204=ORIENTED_EDGE('',*,*,#15637,.F.);
#21205=ORIENTED_EDGE('',*,*,#15636,.T.);
#21206=ORIENTED_EDGE('',*,*,#15638,.F.);
#21207=ORIENTED_EDGE('',*,*,#15639,.F.);
#21208=ORIENTED_EDGE('',*,*,#15640,.F.);
#21209=ORIENTED_EDGE('',*,*,#15639,.T.);
#21210=ORIENTED_EDGE('',*,*,#15641,.F.);
#21211=ORIENTED_EDGE('',*,*,#15642,.F.);
#21212=ORIENTED_EDGE('',*,*,#15643,.F.);
#21213=ORIENTED_EDGE('',*,*,#15642,.T.);
#21214=ORIENTED_EDGE('',*,*,#15644,.F.);
#21215=ORIENTED_EDGE('',*,*,#15645,.F.);
#21216=ORIENTED_EDGE('',*,*,#15646,.F.);
#21217=ORIENTED_EDGE('',*,*,#15645,.T.);
#21218=ORIENTED_EDGE('',*,*,#15647,.F.);
#21219=ORIENTED_EDGE('',*,*,#15648,.F.);
#21220=ORIENTED_EDGE('',*,*,#15649,.F.);
#21221=ORIENTED_EDGE('',*,*,#15648,.T.);
#21222=ORIENTED_EDGE('',*,*,#15650,.F.);
#21223=ORIENTED_EDGE('',*,*,#15651,.F.);
#21224=ORIENTED_EDGE('',*,*,#15652,.F.);
#21225=ORIENTED_EDGE('',*,*,#15651,.T.);
#21226=ORIENTED_EDGE('',*,*,#15653,.F.);
#21227=ORIENTED_EDGE('',*,*,#15654,.F.);
#21228=ORIENTED_EDGE('',*,*,#15655,.F.);
#21229=ORIENTED_EDGE('',*,*,#15654,.T.);
#21230=ORIENTED_EDGE('',*,*,#15656,.F.);
#21231=ORIENTED_EDGE('',*,*,#15657,.F.);
#21232=ORIENTED_EDGE('',*,*,#15658,.F.);
#21233=ORIENTED_EDGE('',*,*,#15657,.T.);
#21234=ORIENTED_EDGE('',*,*,#15659,.F.);
#21235=ORIENTED_EDGE('',*,*,#15660,.F.);
#21236=ORIENTED_EDGE('',*,*,#15661,.F.);
#21237=ORIENTED_EDGE('',*,*,#15660,.T.);
#21238=ORIENTED_EDGE('',*,*,#15662,.F.);
#21239=ORIENTED_EDGE('',*,*,#15663,.F.);
#21240=ORIENTED_EDGE('',*,*,#15664,.F.);
#21241=ORIENTED_EDGE('',*,*,#15663,.T.);
#21242=ORIENTED_EDGE('',*,*,#15665,.F.);
#21243=ORIENTED_EDGE('',*,*,#15666,.F.);
#21244=ORIENTED_EDGE('',*,*,#15667,.F.);
#21245=ORIENTED_EDGE('',*,*,#15666,.T.);
#21246=ORIENTED_EDGE('',*,*,#15668,.F.);
#21247=ORIENTED_EDGE('',*,*,#15669,.F.);
#21248=ORIENTED_EDGE('',*,*,#15670,.F.);
#21249=ORIENTED_EDGE('',*,*,#15669,.T.);
#21250=ORIENTED_EDGE('',*,*,#15671,.F.);
#21251=ORIENTED_EDGE('',*,*,#15672,.F.);
#21252=ORIENTED_EDGE('',*,*,#15673,.F.);
#21253=ORIENTED_EDGE('',*,*,#15672,.T.);
#21254=ORIENTED_EDGE('',*,*,#15674,.F.);
#21255=ORIENTED_EDGE('',*,*,#15675,.F.);
#21256=ORIENTED_EDGE('',*,*,#15676,.F.);
#21257=ORIENTED_EDGE('',*,*,#15675,.T.);
#21258=ORIENTED_EDGE('',*,*,#15677,.F.);
#21259=ORIENTED_EDGE('',*,*,#15678,.F.);
#21260=ORIENTED_EDGE('',*,*,#15679,.F.);
#21261=ORIENTED_EDGE('',*,*,#15678,.T.);
#21262=ORIENTED_EDGE('',*,*,#15680,.F.);
#21263=ORIENTED_EDGE('',*,*,#15681,.F.);
#21264=ORIENTED_EDGE('',*,*,#15682,.F.);
#21265=ORIENTED_EDGE('',*,*,#15681,.T.);
#21266=ORIENTED_EDGE('',*,*,#15683,.F.);
#21267=ORIENTED_EDGE('',*,*,#15684,.F.);
#21268=ORIENTED_EDGE('',*,*,#15685,.F.);
#21269=ORIENTED_EDGE('',*,*,#15684,.T.);
#21270=ORIENTED_EDGE('',*,*,#15686,.F.);
#21271=ORIENTED_EDGE('',*,*,#15687,.F.);
#21272=ORIENTED_EDGE('',*,*,#15688,.F.);
#21273=ORIENTED_EDGE('',*,*,#15687,.T.);
#21274=ORIENTED_EDGE('',*,*,#15689,.F.);
#21275=ORIENTED_EDGE('',*,*,#15690,.F.);
#21276=ORIENTED_EDGE('',*,*,#15691,.F.);
#21277=ORIENTED_EDGE('',*,*,#15690,.T.);
#21278=ORIENTED_EDGE('',*,*,#15692,.F.);
#21279=ORIENTED_EDGE('',*,*,#15693,.F.);
#21280=ORIENTED_EDGE('',*,*,#15694,.F.);
#21281=ORIENTED_EDGE('',*,*,#15693,.T.);
#21282=ORIENTED_EDGE('',*,*,#15695,.F.);
#21283=ORIENTED_EDGE('',*,*,#15696,.F.);
#21284=ORIENTED_EDGE('',*,*,#15697,.F.);
#21285=ORIENTED_EDGE('',*,*,#15696,.T.);
#21286=ORIENTED_EDGE('',*,*,#15698,.F.);
#21287=ORIENTED_EDGE('',*,*,#15699,.F.);
#21288=ORIENTED_EDGE('',*,*,#15700,.F.);
#21289=ORIENTED_EDGE('',*,*,#15699,.T.);
#21290=ORIENTED_EDGE('',*,*,#15701,.F.);
#21291=ORIENTED_EDGE('',*,*,#15702,.F.);
#21292=ORIENTED_EDGE('',*,*,#15703,.F.);
#21293=ORIENTED_EDGE('',*,*,#15702,.T.);
#21294=ORIENTED_EDGE('',*,*,#15704,.F.);
#21295=ORIENTED_EDGE('',*,*,#15705,.F.);
#21296=ORIENTED_EDGE('',*,*,#15706,.F.);
#21297=ORIENTED_EDGE('',*,*,#15705,.T.);
#21298=ORIENTED_EDGE('',*,*,#15707,.F.);
#21299=ORIENTED_EDGE('',*,*,#15708,.F.);
#21300=ORIENTED_EDGE('',*,*,#15709,.F.);
#21301=ORIENTED_EDGE('',*,*,#15708,.T.);
#21302=ORIENTED_EDGE('',*,*,#15710,.F.);
#21303=ORIENTED_EDGE('',*,*,#15711,.F.);
#21304=ORIENTED_EDGE('',*,*,#15712,.F.);
#21305=ORIENTED_EDGE('',*,*,#15711,.T.);
#21306=ORIENTED_EDGE('',*,*,#15713,.F.);
#21307=ORIENTED_EDGE('',*,*,#15714,.F.);
#21308=ORIENTED_EDGE('',*,*,#15715,.F.);
#21309=ORIENTED_EDGE('',*,*,#15714,.T.);
#21310=ORIENTED_EDGE('',*,*,#15716,.F.);
#21311=ORIENTED_EDGE('',*,*,#15717,.F.);
#21312=ORIENTED_EDGE('',*,*,#15718,.F.);
#21313=ORIENTED_EDGE('',*,*,#15717,.T.);
#21314=ORIENTED_EDGE('',*,*,#15719,.F.);
#21315=ORIENTED_EDGE('',*,*,#15720,.F.);
#21316=ORIENTED_EDGE('',*,*,#15721,.F.);
#21317=ORIENTED_EDGE('',*,*,#15720,.T.);
#21318=ORIENTED_EDGE('',*,*,#15722,.F.);
#21319=ORIENTED_EDGE('',*,*,#15723,.F.);
#21320=ORIENTED_EDGE('',*,*,#15724,.F.);
#21321=ORIENTED_EDGE('',*,*,#15723,.T.);
#21322=ORIENTED_EDGE('',*,*,#15725,.F.);
#21323=ORIENTED_EDGE('',*,*,#15726,.F.);
#21324=ORIENTED_EDGE('',*,*,#15727,.F.);
#21325=ORIENTED_EDGE('',*,*,#15726,.T.);
#21326=ORIENTED_EDGE('',*,*,#15728,.F.);
#21327=ORIENTED_EDGE('',*,*,#15729,.F.);
#21328=ORIENTED_EDGE('',*,*,#15730,.F.);
#21329=ORIENTED_EDGE('',*,*,#15729,.T.);
#21330=ORIENTED_EDGE('',*,*,#15731,.F.);
#21331=ORIENTED_EDGE('',*,*,#15732,.F.);
#21332=ORIENTED_EDGE('',*,*,#15733,.F.);
#21333=ORIENTED_EDGE('',*,*,#15732,.T.);
#21334=ORIENTED_EDGE('',*,*,#15734,.F.);
#21335=ORIENTED_EDGE('',*,*,#15735,.F.);
#21336=ORIENTED_EDGE('',*,*,#15736,.F.);
#21337=ORIENTED_EDGE('',*,*,#15735,.T.);
#21338=ORIENTED_EDGE('',*,*,#15737,.F.);
#21339=ORIENTED_EDGE('',*,*,#15738,.F.);
#21340=ORIENTED_EDGE('',*,*,#15739,.F.);
#21341=ORIENTED_EDGE('',*,*,#15738,.T.);
#21342=ORIENTED_EDGE('',*,*,#15740,.F.);
#21343=ORIENTED_EDGE('',*,*,#15741,.F.);
#21344=ORIENTED_EDGE('',*,*,#15742,.F.);
#21345=ORIENTED_EDGE('',*,*,#15741,.T.);
#21346=ORIENTED_EDGE('',*,*,#15743,.F.);
#21347=ORIENTED_EDGE('',*,*,#15744,.F.);
#21348=ORIENTED_EDGE('',*,*,#15745,.F.);
#21349=ORIENTED_EDGE('',*,*,#15744,.T.);
#21350=ORIENTED_EDGE('',*,*,#15746,.F.);
#21351=ORIENTED_EDGE('',*,*,#15747,.F.);
#21352=ORIENTED_EDGE('',*,*,#15748,.F.);
#21353=ORIENTED_EDGE('',*,*,#15747,.T.);
#21354=ORIENTED_EDGE('',*,*,#15749,.F.);
#21355=ORIENTED_EDGE('',*,*,#15750,.F.);
#21356=ORIENTED_EDGE('',*,*,#15751,.F.);
#21357=ORIENTED_EDGE('',*,*,#15750,.T.);
#21358=ORIENTED_EDGE('',*,*,#15752,.F.);
#21359=ORIENTED_EDGE('',*,*,#15753,.F.);
#21360=ORIENTED_EDGE('',*,*,#15754,.F.);
#21361=ORIENTED_EDGE('',*,*,#15753,.T.);
#21362=ORIENTED_EDGE('',*,*,#15755,.F.);
#21363=ORIENTED_EDGE('',*,*,#15756,.F.);
#21364=ORIENTED_EDGE('',*,*,#15757,.F.);
#21365=ORIENTED_EDGE('',*,*,#15756,.T.);
#21366=ORIENTED_EDGE('',*,*,#15758,.F.);
#21367=ORIENTED_EDGE('',*,*,#15759,.F.);
#21368=ORIENTED_EDGE('',*,*,#15760,.F.);
#21369=ORIENTED_EDGE('',*,*,#15759,.T.);
#21370=ORIENTED_EDGE('',*,*,#15761,.F.);
#21371=ORIENTED_EDGE('',*,*,#15762,.F.);
#21372=ORIENTED_EDGE('',*,*,#15763,.F.);
#21373=ORIENTED_EDGE('',*,*,#15762,.T.);
#21374=ORIENTED_EDGE('',*,*,#15764,.F.);
#21375=ORIENTED_EDGE('',*,*,#15765,.F.);
#21376=ORIENTED_EDGE('',*,*,#15766,.F.);
#21377=ORIENTED_EDGE('',*,*,#15765,.T.);
#21378=ORIENTED_EDGE('',*,*,#15767,.F.);
#21379=ORIENTED_EDGE('',*,*,#15768,.F.);
#21380=ORIENTED_EDGE('',*,*,#15769,.F.);
#21381=ORIENTED_EDGE('',*,*,#15768,.T.);
#21382=ORIENTED_EDGE('',*,*,#15770,.F.);
#21383=ORIENTED_EDGE('',*,*,#15771,.F.);
#21384=ORIENTED_EDGE('',*,*,#15772,.F.);
#21385=ORIENTED_EDGE('',*,*,#15771,.T.);
#21386=ORIENTED_EDGE('',*,*,#15773,.F.);
#21387=ORIENTED_EDGE('',*,*,#15774,.F.);
#21388=ORIENTED_EDGE('',*,*,#15775,.F.);
#21389=ORIENTED_EDGE('',*,*,#15774,.T.);
#21390=ORIENTED_EDGE('',*,*,#15776,.F.);
#21391=ORIENTED_EDGE('',*,*,#15777,.F.);
#21392=ORIENTED_EDGE('',*,*,#15778,.F.);
#21393=ORIENTED_EDGE('',*,*,#15777,.T.);
#21394=ORIENTED_EDGE('',*,*,#15779,.F.);
#21395=ORIENTED_EDGE('',*,*,#15780,.F.);
#21396=ORIENTED_EDGE('',*,*,#15781,.F.);
#21397=ORIENTED_EDGE('',*,*,#15780,.T.);
#21398=ORIENTED_EDGE('',*,*,#15782,.F.);
#21399=ORIENTED_EDGE('',*,*,#15783,.F.);
#21400=ORIENTED_EDGE('',*,*,#15784,.F.);
#21401=ORIENTED_EDGE('',*,*,#15783,.T.);
#21402=ORIENTED_EDGE('',*,*,#15785,.F.);
#21403=ORIENTED_EDGE('',*,*,#15786,.F.);
#21404=ORIENTED_EDGE('',*,*,#15787,.F.);
#21405=ORIENTED_EDGE('',*,*,#15786,.T.);
#21406=ORIENTED_EDGE('',*,*,#15788,.F.);
#21407=ORIENTED_EDGE('',*,*,#15789,.F.);
#21408=ORIENTED_EDGE('',*,*,#15790,.F.);
#21409=ORIENTED_EDGE('',*,*,#15789,.T.);
#21410=ORIENTED_EDGE('',*,*,#15791,.F.);
#21411=ORIENTED_EDGE('',*,*,#15792,.F.);
#21412=ORIENTED_EDGE('',*,*,#15793,.F.);
#21413=ORIENTED_EDGE('',*,*,#15792,.T.);
#21414=ORIENTED_EDGE('',*,*,#15794,.F.);
#21415=ORIENTED_EDGE('',*,*,#15795,.F.);
#21416=ORIENTED_EDGE('',*,*,#15796,.F.);
#21417=ORIENTED_EDGE('',*,*,#15795,.T.);
#21418=ORIENTED_EDGE('',*,*,#15797,.F.);
#21419=ORIENTED_EDGE('',*,*,#15798,.F.);
#21420=ORIENTED_EDGE('',*,*,#15799,.F.);
#21421=ORIENTED_EDGE('',*,*,#15798,.T.);
#21422=ORIENTED_EDGE('',*,*,#15800,.F.);
#21423=ORIENTED_EDGE('',*,*,#15801,.F.);
#21424=ORIENTED_EDGE('',*,*,#15802,.F.);
#21425=ORIENTED_EDGE('',*,*,#15801,.T.);
#21426=ORIENTED_EDGE('',*,*,#15803,.F.);
#21427=ORIENTED_EDGE('',*,*,#15804,.F.);
#21428=ORIENTED_EDGE('',*,*,#15805,.F.);
#21429=ORIENTED_EDGE('',*,*,#15804,.T.);
#21430=ORIENTED_EDGE('',*,*,#15806,.F.);
#21431=ORIENTED_EDGE('',*,*,#15807,.F.);
#21432=ORIENTED_EDGE('',*,*,#15808,.F.);
#21433=ORIENTED_EDGE('',*,*,#15807,.T.);
#21434=ORIENTED_EDGE('',*,*,#15809,.F.);
#21435=ORIENTED_EDGE('',*,*,#15810,.F.);
#21436=ORIENTED_EDGE('',*,*,#15811,.F.);
#21437=ORIENTED_EDGE('',*,*,#15810,.T.);
#21438=ORIENTED_EDGE('',*,*,#15812,.F.);
#21439=ORIENTED_EDGE('',*,*,#15813,.F.);
#21440=ORIENTED_EDGE('',*,*,#15814,.F.);
#21441=ORIENTED_EDGE('',*,*,#15813,.T.);
#21442=ORIENTED_EDGE('',*,*,#15815,.F.);
#21443=ORIENTED_EDGE('',*,*,#15816,.F.);
#21444=ORIENTED_EDGE('',*,*,#15817,.F.);
#21445=ORIENTED_EDGE('',*,*,#15816,.T.);
#21446=ORIENTED_EDGE('',*,*,#15818,.F.);
#21447=ORIENTED_EDGE('',*,*,#15819,.F.);
#21448=ORIENTED_EDGE('',*,*,#15820,.F.);
#21449=ORIENTED_EDGE('',*,*,#15819,.T.);
#21450=ORIENTED_EDGE('',*,*,#15821,.F.);
#21451=ORIENTED_EDGE('',*,*,#15822,.F.);
#21452=ORIENTED_EDGE('',*,*,#15823,.F.);
#21453=ORIENTED_EDGE('',*,*,#15822,.T.);
#21454=ORIENTED_EDGE('',*,*,#15824,.F.);
#21455=ORIENTED_EDGE('',*,*,#15825,.F.);
#21456=ORIENTED_EDGE('',*,*,#15826,.F.);
#21457=ORIENTED_EDGE('',*,*,#15825,.T.);
#21458=ORIENTED_EDGE('',*,*,#15827,.F.);
#21459=ORIENTED_EDGE('',*,*,#15828,.F.);
#21460=ORIENTED_EDGE('',*,*,#15829,.F.);
#21461=ORIENTED_EDGE('',*,*,#15828,.T.);
#21462=ORIENTED_EDGE('',*,*,#15830,.F.);
#21463=ORIENTED_EDGE('',*,*,#15831,.F.);
#21464=ORIENTED_EDGE('',*,*,#15832,.F.);
#21465=ORIENTED_EDGE('',*,*,#15831,.T.);
#21466=ORIENTED_EDGE('',*,*,#15833,.F.);
#21467=ORIENTED_EDGE('',*,*,#15834,.F.);
#21468=ORIENTED_EDGE('',*,*,#15835,.F.);
#21469=ORIENTED_EDGE('',*,*,#15834,.T.);
#21470=ORIENTED_EDGE('',*,*,#15836,.F.);
#21471=ORIENTED_EDGE('',*,*,#15837,.F.);
#21472=ORIENTED_EDGE('',*,*,#15838,.F.);
#21473=ORIENTED_EDGE('',*,*,#15837,.T.);
#21474=ORIENTED_EDGE('',*,*,#15839,.F.);
#21475=ORIENTED_EDGE('',*,*,#15840,.F.);
#21476=ORIENTED_EDGE('',*,*,#15841,.F.);
#21477=ORIENTED_EDGE('',*,*,#15840,.T.);
#21478=ORIENTED_EDGE('',*,*,#15842,.F.);
#21479=ORIENTED_EDGE('',*,*,#15843,.F.);
#21480=ORIENTED_EDGE('',*,*,#15844,.F.);
#21481=ORIENTED_EDGE('',*,*,#15843,.T.);
#21482=ORIENTED_EDGE('',*,*,#15845,.F.);
#21483=ORIENTED_EDGE('',*,*,#15846,.F.);
#21484=ORIENTED_EDGE('',*,*,#15847,.F.);
#21485=ORIENTED_EDGE('',*,*,#15846,.T.);
#21486=ORIENTED_EDGE('',*,*,#15848,.F.);
#21487=ORIENTED_EDGE('',*,*,#15849,.F.);
#21488=ORIENTED_EDGE('',*,*,#15850,.F.);
#21489=ORIENTED_EDGE('',*,*,#15849,.T.);
#21490=ORIENTED_EDGE('',*,*,#15851,.F.);
#21491=ORIENTED_EDGE('',*,*,#15852,.F.);
#21492=ORIENTED_EDGE('',*,*,#15853,.F.);
#21493=ORIENTED_EDGE('',*,*,#15852,.T.);
#21494=ORIENTED_EDGE('',*,*,#15854,.F.);
#21495=ORIENTED_EDGE('',*,*,#15855,.F.);
#21496=ORIENTED_EDGE('',*,*,#15856,.F.);
#21497=ORIENTED_EDGE('',*,*,#15855,.T.);
#21498=ORIENTED_EDGE('',*,*,#15857,.F.);
#21499=ORIENTED_EDGE('',*,*,#15858,.F.);
#21500=ORIENTED_EDGE('',*,*,#15859,.F.);
#21501=ORIENTED_EDGE('',*,*,#15858,.T.);
#21502=ORIENTED_EDGE('',*,*,#15860,.F.);
#21503=ORIENTED_EDGE('',*,*,#15861,.F.);
#21504=ORIENTED_EDGE('',*,*,#15862,.F.);
#21505=ORIENTED_EDGE('',*,*,#15861,.T.);
#21506=ORIENTED_EDGE('',*,*,#15863,.F.);
#21507=ORIENTED_EDGE('',*,*,#15864,.F.);
#21508=ORIENTED_EDGE('',*,*,#15865,.F.);
#21509=ORIENTED_EDGE('',*,*,#15864,.T.);
#21510=ORIENTED_EDGE('',*,*,#15866,.F.);
#21511=ORIENTED_EDGE('',*,*,#15867,.F.);
#21512=ORIENTED_EDGE('',*,*,#15868,.F.);
#21513=ORIENTED_EDGE('',*,*,#15867,.T.);
#21514=ORIENTED_EDGE('',*,*,#15869,.F.);
#21515=ORIENTED_EDGE('',*,*,#15870,.F.);
#21516=ORIENTED_EDGE('',*,*,#15871,.F.);
#21517=ORIENTED_EDGE('',*,*,#15870,.T.);
#21518=ORIENTED_EDGE('',*,*,#15872,.F.);
#21519=ORIENTED_EDGE('',*,*,#15873,.F.);
#21520=ORIENTED_EDGE('',*,*,#15874,.F.);
#21521=ORIENTED_EDGE('',*,*,#15873,.T.);
#21522=ORIENTED_EDGE('',*,*,#15875,.F.);
#21523=ORIENTED_EDGE('',*,*,#15876,.F.);
#21524=ORIENTED_EDGE('',*,*,#15877,.F.);
#21525=ORIENTED_EDGE('',*,*,#15876,.T.);
#21526=ORIENTED_EDGE('',*,*,#15878,.F.);
#21527=ORIENTED_EDGE('',*,*,#15879,.F.);
#21528=ORIENTED_EDGE('',*,*,#15880,.F.);
#21529=ORIENTED_EDGE('',*,*,#15879,.T.);
#21530=ORIENTED_EDGE('',*,*,#15881,.F.);
#21531=ORIENTED_EDGE('',*,*,#15882,.F.);
#21532=ORIENTED_EDGE('',*,*,#15883,.F.);
#21533=ORIENTED_EDGE('',*,*,#15882,.T.);
#21534=ORIENTED_EDGE('',*,*,#15884,.F.);
#21535=ORIENTED_EDGE('',*,*,#15885,.F.);
#21536=ORIENTED_EDGE('',*,*,#15886,.F.);
#21537=ORIENTED_EDGE('',*,*,#15885,.T.);
#21538=ORIENTED_EDGE('',*,*,#15887,.F.);
#21539=ORIENTED_EDGE('',*,*,#15888,.F.);
#21540=ORIENTED_EDGE('',*,*,#15889,.F.);
#21541=ORIENTED_EDGE('',*,*,#15888,.T.);
#21542=ORIENTED_EDGE('',*,*,#15890,.F.);
#21543=ORIENTED_EDGE('',*,*,#15891,.F.);
#21544=ORIENTED_EDGE('',*,*,#15892,.F.);
#21545=ORIENTED_EDGE('',*,*,#15891,.T.);
#21546=ORIENTED_EDGE('',*,*,#15893,.F.);
#21547=ORIENTED_EDGE('',*,*,#15894,.F.);
#21548=ORIENTED_EDGE('',*,*,#15895,.F.);
#21549=ORIENTED_EDGE('',*,*,#15894,.T.);
#21550=ORIENTED_EDGE('',*,*,#15896,.F.);
#21551=ORIENTED_EDGE('',*,*,#15897,.F.);
#21552=ORIENTED_EDGE('',*,*,#15898,.F.);
#21553=ORIENTED_EDGE('',*,*,#15897,.T.);
#21554=ORIENTED_EDGE('',*,*,#15899,.F.);
#21555=ORIENTED_EDGE('',*,*,#15900,.F.);
#21556=ORIENTED_EDGE('',*,*,#15901,.F.);
#21557=ORIENTED_EDGE('',*,*,#15900,.T.);
#21558=ORIENTED_EDGE('',*,*,#15902,.F.);
#21559=ORIENTED_EDGE('',*,*,#15903,.F.);
#21560=ORIENTED_EDGE('',*,*,#15904,.F.);
#21561=ORIENTED_EDGE('',*,*,#15903,.T.);
#21562=ORIENTED_EDGE('',*,*,#15905,.F.);
#21563=ORIENTED_EDGE('',*,*,#15906,.F.);
#21564=ORIENTED_EDGE('',*,*,#15907,.F.);
#21565=ORIENTED_EDGE('',*,*,#15906,.T.);
#21566=ORIENTED_EDGE('',*,*,#15908,.F.);
#21567=ORIENTED_EDGE('',*,*,#15909,.F.);
#21568=ORIENTED_EDGE('',*,*,#15910,.F.);
#21569=ORIENTED_EDGE('',*,*,#15909,.T.);
#21570=ORIENTED_EDGE('',*,*,#15911,.F.);
#21571=ORIENTED_EDGE('',*,*,#15912,.F.);
#21572=ORIENTED_EDGE('',*,*,#15913,.F.);
#21573=ORIENTED_EDGE('',*,*,#15912,.T.);
#21574=ORIENTED_EDGE('',*,*,#15914,.F.);
#21575=ORIENTED_EDGE('',*,*,#15915,.F.);
#21576=ORIENTED_EDGE('',*,*,#15916,.F.);
#21577=ORIENTED_EDGE('',*,*,#15915,.T.);
#21578=ORIENTED_EDGE('',*,*,#15917,.F.);
#21579=ORIENTED_EDGE('',*,*,#15918,.F.);
#21580=ORIENTED_EDGE('',*,*,#15919,.F.);
#21581=ORIENTED_EDGE('',*,*,#15918,.T.);
#21582=ORIENTED_EDGE('',*,*,#15920,.F.);
#21583=ORIENTED_EDGE('',*,*,#15921,.F.);
#21584=ORIENTED_EDGE('',*,*,#15922,.F.);
#21585=ORIENTED_EDGE('',*,*,#15921,.T.);
#21586=ORIENTED_EDGE('',*,*,#15923,.F.);
#21587=ORIENTED_EDGE('',*,*,#15924,.F.);
#21588=ORIENTED_EDGE('',*,*,#15925,.F.);
#21589=ORIENTED_EDGE('',*,*,#15924,.T.);
#21590=ORIENTED_EDGE('',*,*,#15926,.F.);
#21591=ORIENTED_EDGE('',*,*,#15927,.F.);
#21592=ORIENTED_EDGE('',*,*,#15928,.F.);
#21593=ORIENTED_EDGE('',*,*,#15927,.T.);
#21594=ORIENTED_EDGE('',*,*,#15929,.F.);
#21595=ORIENTED_EDGE('',*,*,#15930,.F.);
#21596=ORIENTED_EDGE('',*,*,#15931,.F.);
#21597=ORIENTED_EDGE('',*,*,#15930,.T.);
#21598=ORIENTED_EDGE('',*,*,#15932,.F.);
#21599=ORIENTED_EDGE('',*,*,#15933,.F.);
#21600=ORIENTED_EDGE('',*,*,#15934,.F.);
#21601=ORIENTED_EDGE('',*,*,#15933,.T.);
#21602=ORIENTED_EDGE('',*,*,#15935,.F.);
#21603=ORIENTED_EDGE('',*,*,#15936,.F.);
#21604=ORIENTED_EDGE('',*,*,#15937,.F.);
#21605=ORIENTED_EDGE('',*,*,#15936,.T.);
#21606=ORIENTED_EDGE('',*,*,#15938,.F.);
#21607=ORIENTED_EDGE('',*,*,#15939,.F.);
#21608=ORIENTED_EDGE('',*,*,#15940,.F.);
#21609=ORIENTED_EDGE('',*,*,#15939,.T.);
#21610=ORIENTED_EDGE('',*,*,#15941,.F.);
#21611=ORIENTED_EDGE('',*,*,#15942,.F.);
#21612=ORIENTED_EDGE('',*,*,#15943,.F.);
#21613=ORIENTED_EDGE('',*,*,#15942,.T.);
#21614=ORIENTED_EDGE('',*,*,#15944,.F.);
#21615=ORIENTED_EDGE('',*,*,#15945,.F.);
#21616=ORIENTED_EDGE('',*,*,#15946,.F.);
#21617=ORIENTED_EDGE('',*,*,#15945,.T.);
#21618=ORIENTED_EDGE('',*,*,#15947,.F.);
#21619=ORIENTED_EDGE('',*,*,#15948,.F.);
#21620=ORIENTED_EDGE('',*,*,#15949,.F.);
#21621=ORIENTED_EDGE('',*,*,#15948,.T.);
#21622=ORIENTED_EDGE('',*,*,#15950,.F.);
#21623=ORIENTED_EDGE('',*,*,#15951,.F.);
#21624=ORIENTED_EDGE('',*,*,#15952,.F.);
#21625=ORIENTED_EDGE('',*,*,#15951,.T.);
#21626=ORIENTED_EDGE('',*,*,#15953,.F.);
#21627=ORIENTED_EDGE('',*,*,#15954,.F.);
#21628=ORIENTED_EDGE('',*,*,#15955,.F.);
#21629=ORIENTED_EDGE('',*,*,#15954,.T.);
#21630=ORIENTED_EDGE('',*,*,#15956,.F.);
#21631=ORIENTED_EDGE('',*,*,#15957,.F.);
#21632=ORIENTED_EDGE('',*,*,#15958,.F.);
#21633=ORIENTED_EDGE('',*,*,#15957,.T.);
#21634=ORIENTED_EDGE('',*,*,#15959,.F.);
#21635=ORIENTED_EDGE('',*,*,#15960,.F.);
#21636=ORIENTED_EDGE('',*,*,#15961,.F.);
#21637=ORIENTED_EDGE('',*,*,#15960,.T.);
#21638=ORIENTED_EDGE('',*,*,#15962,.F.);
#21639=ORIENTED_EDGE('',*,*,#15963,.F.);
#21640=ORIENTED_EDGE('',*,*,#15964,.F.);
#21641=ORIENTED_EDGE('',*,*,#15963,.T.);
#21642=ORIENTED_EDGE('',*,*,#15965,.F.);
#21643=ORIENTED_EDGE('',*,*,#15966,.F.);
#21644=ORIENTED_EDGE('',*,*,#15967,.F.);
#21645=ORIENTED_EDGE('',*,*,#15966,.T.);
#21646=ORIENTED_EDGE('',*,*,#15968,.F.);
#21647=ORIENTED_EDGE('',*,*,#15969,.F.);
#21648=ORIENTED_EDGE('',*,*,#15970,.F.);
#21649=ORIENTED_EDGE('',*,*,#15969,.T.);
#21650=ORIENTED_EDGE('',*,*,#15971,.F.);
#21651=ORIENTED_EDGE('',*,*,#15972,.F.);
#21652=ORIENTED_EDGE('',*,*,#15973,.F.);
#21653=ORIENTED_EDGE('',*,*,#15972,.T.);
#21654=ORIENTED_EDGE('',*,*,#15974,.F.);
#21655=ORIENTED_EDGE('',*,*,#15975,.F.);
#21656=ORIENTED_EDGE('',*,*,#15976,.F.);
#21657=ORIENTED_EDGE('',*,*,#15975,.T.);
#21658=ORIENTED_EDGE('',*,*,#15977,.F.);
#21659=ORIENTED_EDGE('',*,*,#15978,.F.);
#21660=ORIENTED_EDGE('',*,*,#15979,.F.);
#21661=ORIENTED_EDGE('',*,*,#15978,.T.);
#21662=ORIENTED_EDGE('',*,*,#15980,.F.);
#21663=ORIENTED_EDGE('',*,*,#15981,.F.);
#21664=ORIENTED_EDGE('',*,*,#15982,.F.);
#21665=ORIENTED_EDGE('',*,*,#15981,.T.);
#21666=ORIENTED_EDGE('',*,*,#15983,.F.);
#21667=ORIENTED_EDGE('',*,*,#15984,.F.);
#21668=ORIENTED_EDGE('',*,*,#15985,.F.);
#21669=ORIENTED_EDGE('',*,*,#15984,.T.);
#21670=ORIENTED_EDGE('',*,*,#15986,.F.);
#21671=ORIENTED_EDGE('',*,*,#15987,.F.);
#21672=ORIENTED_EDGE('',*,*,#15988,.F.);
#21673=ORIENTED_EDGE('',*,*,#15987,.T.);
#21674=ORIENTED_EDGE('',*,*,#15989,.F.);
#21675=ORIENTED_EDGE('',*,*,#15990,.F.);
#21676=ORIENTED_EDGE('',*,*,#15991,.F.);
#21677=ORIENTED_EDGE('',*,*,#15990,.T.);
#21678=ORIENTED_EDGE('',*,*,#15992,.F.);
#21679=ORIENTED_EDGE('',*,*,#15993,.F.);
#21680=ORIENTED_EDGE('',*,*,#15994,.F.);
#21681=ORIENTED_EDGE('',*,*,#15993,.T.);
#21682=ORIENTED_EDGE('',*,*,#15995,.F.);
#21683=ORIENTED_EDGE('',*,*,#15996,.F.);
#21684=ORIENTED_EDGE('',*,*,#15997,.F.);
#21685=ORIENTED_EDGE('',*,*,#15996,.T.);
#21686=ORIENTED_EDGE('',*,*,#15998,.F.);
#21687=ORIENTED_EDGE('',*,*,#15999,.F.);
#21688=ORIENTED_EDGE('',*,*,#16000,.F.);
#21689=ORIENTED_EDGE('',*,*,#15999,.T.);
#21690=ORIENTED_EDGE('',*,*,#16001,.F.);
#21691=ORIENTED_EDGE('',*,*,#15111,.F.);
#21692=ORIENTED_EDGE('',*,*,#15116,.F.);
#21693=ORIENTED_EDGE('',*,*,#15125,.F.);
#21694=ORIENTED_EDGE('',*,*,#16001,.T.);
#21695=ORIENTED_EDGE('',*,*,#15998,.T.);
#21696=ORIENTED_EDGE('',*,*,#15995,.T.);
#21697=ORIENTED_EDGE('',*,*,#15992,.T.);
#21698=ORIENTED_EDGE('',*,*,#15989,.T.);
#21699=ORIENTED_EDGE('',*,*,#15986,.T.);
#21700=ORIENTED_EDGE('',*,*,#15983,.T.);
#21701=ORIENTED_EDGE('',*,*,#15980,.T.);
#21702=ORIENTED_EDGE('',*,*,#15977,.T.);
#21703=ORIENTED_EDGE('',*,*,#15974,.T.);
#21704=ORIENTED_EDGE('',*,*,#15971,.T.);
#21705=ORIENTED_EDGE('',*,*,#15968,.T.);
#21706=ORIENTED_EDGE('',*,*,#15965,.T.);
#21707=ORIENTED_EDGE('',*,*,#15962,.T.);
#21708=ORIENTED_EDGE('',*,*,#15959,.T.);
#21709=ORIENTED_EDGE('',*,*,#15956,.T.);
#21710=ORIENTED_EDGE('',*,*,#15953,.T.);
#21711=ORIENTED_EDGE('',*,*,#15950,.T.);
#21712=ORIENTED_EDGE('',*,*,#15947,.T.);
#21713=ORIENTED_EDGE('',*,*,#15944,.T.);
#21714=ORIENTED_EDGE('',*,*,#15941,.T.);
#21715=ORIENTED_EDGE('',*,*,#15938,.T.);
#21716=ORIENTED_EDGE('',*,*,#15935,.T.);
#21717=ORIENTED_EDGE('',*,*,#15932,.T.);
#21718=ORIENTED_EDGE('',*,*,#15929,.T.);
#21719=ORIENTED_EDGE('',*,*,#15926,.T.);
#21720=ORIENTED_EDGE('',*,*,#15923,.T.);
#21721=ORIENTED_EDGE('',*,*,#15920,.T.);
#21722=ORIENTED_EDGE('',*,*,#15917,.T.);
#21723=ORIENTED_EDGE('',*,*,#15914,.T.);
#21724=ORIENTED_EDGE('',*,*,#15911,.T.);
#21725=ORIENTED_EDGE('',*,*,#15908,.T.);
#21726=ORIENTED_EDGE('',*,*,#15905,.T.);
#21727=ORIENTED_EDGE('',*,*,#15902,.T.);
#21728=ORIENTED_EDGE('',*,*,#15899,.T.);
#21729=ORIENTED_EDGE('',*,*,#15896,.T.);
#21730=ORIENTED_EDGE('',*,*,#15893,.T.);
#21731=ORIENTED_EDGE('',*,*,#15890,.T.);
#21732=ORIENTED_EDGE('',*,*,#15887,.T.);
#21733=ORIENTED_EDGE('',*,*,#15884,.T.);
#21734=ORIENTED_EDGE('',*,*,#15881,.T.);
#21735=ORIENTED_EDGE('',*,*,#15878,.T.);
#21736=ORIENTED_EDGE('',*,*,#15875,.T.);
#21737=ORIENTED_EDGE('',*,*,#15872,.T.);
#21738=ORIENTED_EDGE('',*,*,#15869,.T.);
#21739=ORIENTED_EDGE('',*,*,#15866,.T.);
#21740=ORIENTED_EDGE('',*,*,#15863,.T.);
#21741=ORIENTED_EDGE('',*,*,#15860,.T.);
#21742=ORIENTED_EDGE('',*,*,#15857,.T.);
#21743=ORIENTED_EDGE('',*,*,#15854,.T.);
#21744=ORIENTED_EDGE('',*,*,#15851,.T.);
#21745=ORIENTED_EDGE('',*,*,#15848,.T.);
#21746=ORIENTED_EDGE('',*,*,#15845,.T.);
#21747=ORIENTED_EDGE('',*,*,#15842,.T.);
#21748=ORIENTED_EDGE('',*,*,#15839,.T.);
#21749=ORIENTED_EDGE('',*,*,#15836,.T.);
#21750=ORIENTED_EDGE('',*,*,#15833,.T.);
#21751=ORIENTED_EDGE('',*,*,#15830,.T.);
#21752=ORIENTED_EDGE('',*,*,#15827,.T.);
#21753=ORIENTED_EDGE('',*,*,#15824,.T.);
#21754=ORIENTED_EDGE('',*,*,#15821,.T.);
#21755=ORIENTED_EDGE('',*,*,#15818,.T.);
#21756=ORIENTED_EDGE('',*,*,#15815,.T.);
#21757=ORIENTED_EDGE('',*,*,#15812,.T.);
#21758=ORIENTED_EDGE('',*,*,#15809,.T.);
#21759=ORIENTED_EDGE('',*,*,#15806,.T.);
#21760=ORIENTED_EDGE('',*,*,#15803,.T.);
#21761=ORIENTED_EDGE('',*,*,#15800,.T.);
#21762=ORIENTED_EDGE('',*,*,#15797,.T.);
#21763=ORIENTED_EDGE('',*,*,#15794,.T.);
#21764=ORIENTED_EDGE('',*,*,#15791,.T.);
#21765=ORIENTED_EDGE('',*,*,#15788,.T.);
#21766=ORIENTED_EDGE('',*,*,#15785,.T.);
#21767=ORIENTED_EDGE('',*,*,#15782,.T.);
#21768=ORIENTED_EDGE('',*,*,#15779,.T.);
#21769=ORIENTED_EDGE('',*,*,#15776,.T.);
#21770=ORIENTED_EDGE('',*,*,#15773,.T.);
#21771=ORIENTED_EDGE('',*,*,#15770,.T.);
#21772=ORIENTED_EDGE('',*,*,#15767,.T.);
#21773=ORIENTED_EDGE('',*,*,#15764,.T.);
#21774=ORIENTED_EDGE('',*,*,#15761,.T.);
#21775=ORIENTED_EDGE('',*,*,#15758,.T.);
#21776=ORIENTED_EDGE('',*,*,#15755,.T.);
#21777=ORIENTED_EDGE('',*,*,#15752,.T.);
#21778=ORIENTED_EDGE('',*,*,#15749,.T.);
#21779=ORIENTED_EDGE('',*,*,#15746,.T.);
#21780=ORIENTED_EDGE('',*,*,#15743,.T.);
#21781=ORIENTED_EDGE('',*,*,#15740,.T.);
#21782=ORIENTED_EDGE('',*,*,#15737,.T.);
#21783=ORIENTED_EDGE('',*,*,#15734,.T.);
#21784=ORIENTED_EDGE('',*,*,#15731,.T.);
#21785=ORIENTED_EDGE('',*,*,#15728,.T.);
#21786=ORIENTED_EDGE('',*,*,#15725,.T.);
#21787=ORIENTED_EDGE('',*,*,#15722,.T.);
#21788=ORIENTED_EDGE('',*,*,#15719,.T.);
#21789=ORIENTED_EDGE('',*,*,#15716,.T.);
#21790=ORIENTED_EDGE('',*,*,#15713,.T.);
#21791=ORIENTED_EDGE('',*,*,#15710,.T.);
#21792=ORIENTED_EDGE('',*,*,#15707,.T.);
#21793=ORIENTED_EDGE('',*,*,#15704,.T.);
#21794=ORIENTED_EDGE('',*,*,#15701,.T.);
#21795=ORIENTED_EDGE('',*,*,#15698,.T.);
#21796=ORIENTED_EDGE('',*,*,#15695,.T.);
#21797=ORIENTED_EDGE('',*,*,#15692,.T.);
#21798=ORIENTED_EDGE('',*,*,#15689,.T.);
#21799=ORIENTED_EDGE('',*,*,#15686,.T.);
#21800=ORIENTED_EDGE('',*,*,#15683,.T.);
#21801=ORIENTED_EDGE('',*,*,#15680,.T.);
#21802=ORIENTED_EDGE('',*,*,#15677,.T.);
#21803=ORIENTED_EDGE('',*,*,#15674,.T.);
#21804=ORIENTED_EDGE('',*,*,#15671,.T.);
#21805=ORIENTED_EDGE('',*,*,#15668,.T.);
#21806=ORIENTED_EDGE('',*,*,#15665,.T.);
#21807=ORIENTED_EDGE('',*,*,#15662,.T.);
#21808=ORIENTED_EDGE('',*,*,#15659,.T.);
#21809=ORIENTED_EDGE('',*,*,#15656,.T.);
#21810=ORIENTED_EDGE('',*,*,#15653,.T.);
#21811=ORIENTED_EDGE('',*,*,#15650,.T.);
#21812=ORIENTED_EDGE('',*,*,#15647,.T.);
#21813=ORIENTED_EDGE('',*,*,#15644,.T.);
#21814=ORIENTED_EDGE('',*,*,#15641,.T.);
#21815=ORIENTED_EDGE('',*,*,#15638,.T.);
#21816=ORIENTED_EDGE('',*,*,#15635,.T.);
#21817=ORIENTED_EDGE('',*,*,#15632,.T.);
#21818=ORIENTED_EDGE('',*,*,#15629,.T.);
#21819=ORIENTED_EDGE('',*,*,#15626,.T.);
#21820=ORIENTED_EDGE('',*,*,#15623,.T.);
#21821=ORIENTED_EDGE('',*,*,#15620,.T.);
#21822=ORIENTED_EDGE('',*,*,#15617,.T.);
#21823=ORIENTED_EDGE('',*,*,#15614,.T.);
#21824=ORIENTED_EDGE('',*,*,#15611,.T.);
#21825=ORIENTED_EDGE('',*,*,#15608,.T.);
#21826=ORIENTED_EDGE('',*,*,#15605,.T.);
#21827=ORIENTED_EDGE('',*,*,#15602,.T.);
#21828=ORIENTED_EDGE('',*,*,#15599,.T.);
#21829=ORIENTED_EDGE('',*,*,#15596,.T.);
#21830=ORIENTED_EDGE('',*,*,#15593,.T.);
#21831=ORIENTED_EDGE('',*,*,#15590,.T.);
#21832=ORIENTED_EDGE('',*,*,#15587,.T.);
#21833=ORIENTED_EDGE('',*,*,#15584,.T.);
#21834=ORIENTED_EDGE('',*,*,#15581,.T.);
#21835=ORIENTED_EDGE('',*,*,#15578,.T.);
#21836=ORIENTED_EDGE('',*,*,#15575,.T.);
#21837=ORIENTED_EDGE('',*,*,#15572,.T.);
#21838=ORIENTED_EDGE('',*,*,#15569,.T.);
#21839=ORIENTED_EDGE('',*,*,#15566,.T.);
#21840=ORIENTED_EDGE('',*,*,#15563,.T.);
#21841=ORIENTED_EDGE('',*,*,#15560,.T.);
#21842=ORIENTED_EDGE('',*,*,#15557,.T.);
#21843=ORIENTED_EDGE('',*,*,#15554,.T.);
#21844=ORIENTED_EDGE('',*,*,#15551,.T.);
#21845=ORIENTED_EDGE('',*,*,#15548,.T.);
#21846=ORIENTED_EDGE('',*,*,#15545,.T.);
#21847=ORIENTED_EDGE('',*,*,#15542,.T.);
#21848=ORIENTED_EDGE('',*,*,#15539,.T.);
#21849=ORIENTED_EDGE('',*,*,#15536,.T.);
#21850=ORIENTED_EDGE('',*,*,#15533,.T.);
#21851=ORIENTED_EDGE('',*,*,#15530,.T.);
#21852=ORIENTED_EDGE('',*,*,#15527,.T.);
#21853=ORIENTED_EDGE('',*,*,#15524,.T.);
#21854=ORIENTED_EDGE('',*,*,#15521,.T.);
#21855=ORIENTED_EDGE('',*,*,#15518,.T.);
#21856=ORIENTED_EDGE('',*,*,#15515,.T.);
#21857=ORIENTED_EDGE('',*,*,#15512,.T.);
#21858=ORIENTED_EDGE('',*,*,#15509,.T.);
#21859=ORIENTED_EDGE('',*,*,#15506,.T.);
#21860=ORIENTED_EDGE('',*,*,#15503,.T.);
#21861=ORIENTED_EDGE('',*,*,#15500,.T.);
#21862=ORIENTED_EDGE('',*,*,#15497,.T.);
#21863=ORIENTED_EDGE('',*,*,#15494,.T.);
#21864=ORIENTED_EDGE('',*,*,#15491,.T.);
#21865=ORIENTED_EDGE('',*,*,#15488,.T.);
#21866=ORIENTED_EDGE('',*,*,#15485,.T.);
#21867=ORIENTED_EDGE('',*,*,#15482,.T.);
#21868=ORIENTED_EDGE('',*,*,#15479,.T.);
#21869=ORIENTED_EDGE('',*,*,#15476,.T.);
#21870=ORIENTED_EDGE('',*,*,#15473,.T.);
#21871=ORIENTED_EDGE('',*,*,#15470,.T.);
#21872=ORIENTED_EDGE('',*,*,#15467,.T.);
#21873=ORIENTED_EDGE('',*,*,#15464,.T.);
#21874=ORIENTED_EDGE('',*,*,#15461,.T.);
#21875=ORIENTED_EDGE('',*,*,#15458,.T.);
#21876=ORIENTED_EDGE('',*,*,#15455,.T.);
#21877=ORIENTED_EDGE('',*,*,#15452,.T.);
#21878=ORIENTED_EDGE('',*,*,#15449,.T.);
#21879=ORIENTED_EDGE('',*,*,#15446,.T.);
#21880=ORIENTED_EDGE('',*,*,#15443,.T.);
#21881=ORIENTED_EDGE('',*,*,#15440,.T.);
#21882=ORIENTED_EDGE('',*,*,#15437,.T.);
#21883=ORIENTED_EDGE('',*,*,#15434,.T.);
#21884=ORIENTED_EDGE('',*,*,#15431,.T.);
#21885=ORIENTED_EDGE('',*,*,#15428,.T.);
#21886=ORIENTED_EDGE('',*,*,#15425,.T.);
#21887=ORIENTED_EDGE('',*,*,#15422,.T.);
#21888=ORIENTED_EDGE('',*,*,#15419,.T.);
#21889=ORIENTED_EDGE('',*,*,#15416,.T.);
#21890=ORIENTED_EDGE('',*,*,#15413,.T.);
#21891=ORIENTED_EDGE('',*,*,#15410,.T.);
#21892=ORIENTED_EDGE('',*,*,#15407,.T.);
#21893=ORIENTED_EDGE('',*,*,#15404,.T.);
#21894=ORIENTED_EDGE('',*,*,#15401,.T.);
#21895=ORIENTED_EDGE('',*,*,#15398,.T.);
#21896=ORIENTED_EDGE('',*,*,#15395,.T.);
#21897=ORIENTED_EDGE('',*,*,#15392,.T.);
#21898=ORIENTED_EDGE('',*,*,#15389,.T.);
#21899=ORIENTED_EDGE('',*,*,#15386,.T.);
#21900=ORIENTED_EDGE('',*,*,#15383,.T.);
#21901=ORIENTED_EDGE('',*,*,#15380,.T.);
#21902=ORIENTED_EDGE('',*,*,#15377,.T.);
#21903=ORIENTED_EDGE('',*,*,#15374,.T.);
#21904=ORIENTED_EDGE('',*,*,#15371,.T.);
#21905=ORIENTED_EDGE('',*,*,#15368,.T.);
#21906=ORIENTED_EDGE('',*,*,#15365,.T.);
#21907=ORIENTED_EDGE('',*,*,#15362,.T.);
#21908=ORIENTED_EDGE('',*,*,#15359,.T.);
#21909=ORIENTED_EDGE('',*,*,#15356,.T.);
#21910=ORIENTED_EDGE('',*,*,#15353,.T.);
#21911=ORIENTED_EDGE('',*,*,#15350,.T.);
#21912=ORIENTED_EDGE('',*,*,#15347,.T.);
#21913=ORIENTED_EDGE('',*,*,#15344,.T.);
#21914=ORIENTED_EDGE('',*,*,#15341,.T.);
#21915=ORIENTED_EDGE('',*,*,#15338,.T.);
#21916=ORIENTED_EDGE('',*,*,#15335,.T.);
#21917=ORIENTED_EDGE('',*,*,#15332,.T.);
#21918=ORIENTED_EDGE('',*,*,#15329,.T.);
#21919=ORIENTED_EDGE('',*,*,#15326,.T.);
#21920=ORIENTED_EDGE('',*,*,#15323,.T.);
#21921=ORIENTED_EDGE('',*,*,#15320,.T.);
#21922=ORIENTED_EDGE('',*,*,#15317,.T.);
#21923=ORIENTED_EDGE('',*,*,#15314,.T.);
#21924=ORIENTED_EDGE('',*,*,#15311,.T.);
#21925=ORIENTED_EDGE('',*,*,#15308,.T.);
#21926=ORIENTED_EDGE('',*,*,#15305,.T.);
#21927=ORIENTED_EDGE('',*,*,#15302,.T.);
#21928=ORIENTED_EDGE('',*,*,#15299,.T.);
#21929=ORIENTED_EDGE('',*,*,#15296,.T.);
#21930=ORIENTED_EDGE('',*,*,#15293,.T.);
#21931=ORIENTED_EDGE('',*,*,#15290,.T.);
#21932=ORIENTED_EDGE('',*,*,#15287,.T.);
#21933=ORIENTED_EDGE('',*,*,#15284,.T.);
#21934=ORIENTED_EDGE('',*,*,#15281,.T.);
#21935=ORIENTED_EDGE('',*,*,#15278,.T.);
#21936=ORIENTED_EDGE('',*,*,#15275,.T.);
#21937=ORIENTED_EDGE('',*,*,#15272,.T.);
#21938=ORIENTED_EDGE('',*,*,#15269,.T.);
#21939=ORIENTED_EDGE('',*,*,#15266,.T.);
#21940=ORIENTED_EDGE('',*,*,#15263,.T.);
#21941=ORIENTED_EDGE('',*,*,#15260,.T.);
#21942=ORIENTED_EDGE('',*,*,#15257,.T.);
#21943=ORIENTED_EDGE('',*,*,#15254,.T.);
#21944=ORIENTED_EDGE('',*,*,#15251,.T.);
#21945=ORIENTED_EDGE('',*,*,#15248,.T.);
#21946=ORIENTED_EDGE('',*,*,#15245,.T.);
#21947=ORIENTED_EDGE('',*,*,#15242,.T.);
#21948=ORIENTED_EDGE('',*,*,#15239,.T.);
#21949=ORIENTED_EDGE('',*,*,#15236,.T.);
#21950=ORIENTED_EDGE('',*,*,#15233,.T.);
#21951=ORIENTED_EDGE('',*,*,#15230,.T.);
#21952=ORIENTED_EDGE('',*,*,#15227,.T.);
#21953=ORIENTED_EDGE('',*,*,#15224,.T.);
#21954=ORIENTED_EDGE('',*,*,#15221,.T.);
#21955=ORIENTED_EDGE('',*,*,#15218,.T.);
#21956=ORIENTED_EDGE('',*,*,#15215,.T.);
#21957=ORIENTED_EDGE('',*,*,#15212,.T.);
#21958=ORIENTED_EDGE('',*,*,#15209,.T.);
#21959=ORIENTED_EDGE('',*,*,#15206,.T.);
#21960=ORIENTED_EDGE('',*,*,#15203,.T.);
#21961=ORIENTED_EDGE('',*,*,#15200,.T.);
#21962=ORIENTED_EDGE('',*,*,#15197,.T.);
#21963=ORIENTED_EDGE('',*,*,#15194,.T.);
#21964=ORIENTED_EDGE('',*,*,#15191,.T.);
#21965=ORIENTED_EDGE('',*,*,#15188,.T.);
#21966=ORIENTED_EDGE('',*,*,#15185,.T.);
#21967=ORIENTED_EDGE('',*,*,#15182,.T.);
#21968=ORIENTED_EDGE('',*,*,#15179,.T.);
#21969=ORIENTED_EDGE('',*,*,#15176,.T.);
#21970=ORIENTED_EDGE('',*,*,#15173,.T.);
#21971=ORIENTED_EDGE('',*,*,#15170,.T.);
#21972=ORIENTED_EDGE('',*,*,#15167,.T.);
#21973=ORIENTED_EDGE('',*,*,#15101,.F.);
#21974=ORIENTED_EDGE('',*,*,#15103,.F.);
#21975=ORIENTED_EDGE('',*,*,#15106,.F.);
#21976=ORIENTED_EDGE('',*,*,#15109,.F.);
#21977=ORIENTED_EDGE('',*,*,#15112,.F.);
#21978=ORIENTED_EDGE('',*,*,#15163,.T.);
#21979=ORIENTED_EDGE('',*,*,#15160,.T.);
#21980=ORIENTED_EDGE('',*,*,#15157,.T.);
#21981=ORIENTED_EDGE('',*,*,#15154,.T.);
#21982=ORIENTED_EDGE('',*,*,#15151,.T.);
#21983=ORIENTED_EDGE('',*,*,#15148,.T.);
#21984=ORIENTED_EDGE('',*,*,#15145,.T.);
#21985=ORIENTED_EDGE('',*,*,#15142,.T.);
#21986=ORIENTED_EDGE('',*,*,#15139,.T.);
#21987=ORIENTED_EDGE('',*,*,#15136,.T.);
#21988=ORIENTED_EDGE('',*,*,#15166,.T.);
#21989=ORIENTED_EDGE('',*,*,#15169,.T.);
#21990=ORIENTED_EDGE('',*,*,#15172,.T.);
#21991=ORIENTED_EDGE('',*,*,#15175,.T.);
#21992=ORIENTED_EDGE('',*,*,#15178,.T.);
#21993=ORIENTED_EDGE('',*,*,#15181,.T.);
#21994=ORIENTED_EDGE('',*,*,#15184,.T.);
#21995=ORIENTED_EDGE('',*,*,#15187,.T.);
#21996=ORIENTED_EDGE('',*,*,#15190,.T.);
#21997=ORIENTED_EDGE('',*,*,#15193,.T.);
#21998=ORIENTED_EDGE('',*,*,#15196,.T.);
#21999=ORIENTED_EDGE('',*,*,#15199,.T.);
#22000=ORIENTED_EDGE('',*,*,#15202,.T.);
#22001=ORIENTED_EDGE('',*,*,#15205,.T.);
#22002=ORIENTED_EDGE('',*,*,#15208,.T.);
#22003=ORIENTED_EDGE('',*,*,#15211,.T.);
#22004=ORIENTED_EDGE('',*,*,#15214,.T.);
#22005=ORIENTED_EDGE('',*,*,#15217,.T.);
#22006=ORIENTED_EDGE('',*,*,#15220,.T.);
#22007=ORIENTED_EDGE('',*,*,#15223,.T.);
#22008=ORIENTED_EDGE('',*,*,#15226,.T.);
#22009=ORIENTED_EDGE('',*,*,#15229,.T.);
#22010=ORIENTED_EDGE('',*,*,#15232,.T.);
#22011=ORIENTED_EDGE('',*,*,#15235,.T.);
#22012=ORIENTED_EDGE('',*,*,#15238,.T.);
#22013=ORIENTED_EDGE('',*,*,#15241,.T.);
#22014=ORIENTED_EDGE('',*,*,#15244,.T.);
#22015=ORIENTED_EDGE('',*,*,#15247,.T.);
#22016=ORIENTED_EDGE('',*,*,#15250,.T.);
#22017=ORIENTED_EDGE('',*,*,#15253,.T.);
#22018=ORIENTED_EDGE('',*,*,#15256,.T.);
#22019=ORIENTED_EDGE('',*,*,#15259,.T.);
#22020=ORIENTED_EDGE('',*,*,#15262,.T.);
#22021=ORIENTED_EDGE('',*,*,#15265,.T.);
#22022=ORIENTED_EDGE('',*,*,#15268,.T.);
#22023=ORIENTED_EDGE('',*,*,#15271,.T.);
#22024=ORIENTED_EDGE('',*,*,#15274,.T.);
#22025=ORIENTED_EDGE('',*,*,#15277,.T.);
#22026=ORIENTED_EDGE('',*,*,#15280,.T.);
#22027=ORIENTED_EDGE('',*,*,#15283,.T.);
#22028=ORIENTED_EDGE('',*,*,#15286,.T.);
#22029=ORIENTED_EDGE('',*,*,#15289,.T.);
#22030=ORIENTED_EDGE('',*,*,#15292,.T.);
#22031=ORIENTED_EDGE('',*,*,#15295,.T.);
#22032=ORIENTED_EDGE('',*,*,#15298,.T.);
#22033=ORIENTED_EDGE('',*,*,#15301,.T.);
#22034=ORIENTED_EDGE('',*,*,#15304,.T.);
#22035=ORIENTED_EDGE('',*,*,#15307,.T.);
#22036=ORIENTED_EDGE('',*,*,#15310,.T.);
#22037=ORIENTED_EDGE('',*,*,#15313,.T.);
#22038=ORIENTED_EDGE('',*,*,#15316,.T.);
#22039=ORIENTED_EDGE('',*,*,#15319,.T.);
#22040=ORIENTED_EDGE('',*,*,#15322,.T.);
#22041=ORIENTED_EDGE('',*,*,#15325,.T.);
#22042=ORIENTED_EDGE('',*,*,#15328,.T.);
#22043=ORIENTED_EDGE('',*,*,#15331,.T.);
#22044=ORIENTED_EDGE('',*,*,#15334,.T.);
#22045=ORIENTED_EDGE('',*,*,#15337,.T.);
#22046=ORIENTED_EDGE('',*,*,#15340,.T.);
#22047=ORIENTED_EDGE('',*,*,#15343,.T.);
#22048=ORIENTED_EDGE('',*,*,#15346,.T.);
#22049=ORIENTED_EDGE('',*,*,#15349,.T.);
#22050=ORIENTED_EDGE('',*,*,#15352,.T.);
#22051=ORIENTED_EDGE('',*,*,#15355,.T.);
#22052=ORIENTED_EDGE('',*,*,#15358,.T.);
#22053=ORIENTED_EDGE('',*,*,#15361,.T.);
#22054=ORIENTED_EDGE('',*,*,#15364,.T.);
#22055=ORIENTED_EDGE('',*,*,#15367,.T.);
#22056=ORIENTED_EDGE('',*,*,#15370,.T.);
#22057=ORIENTED_EDGE('',*,*,#15373,.T.);
#22058=ORIENTED_EDGE('',*,*,#15376,.T.);
#22059=ORIENTED_EDGE('',*,*,#15379,.T.);
#22060=ORIENTED_EDGE('',*,*,#15382,.T.);
#22061=ORIENTED_EDGE('',*,*,#15385,.T.);
#22062=ORIENTED_EDGE('',*,*,#15388,.T.);
#22063=ORIENTED_EDGE('',*,*,#15391,.T.);
#22064=ORIENTED_EDGE('',*,*,#15394,.T.);
#22065=ORIENTED_EDGE('',*,*,#15397,.T.);
#22066=ORIENTED_EDGE('',*,*,#15400,.T.);
#22067=ORIENTED_EDGE('',*,*,#15403,.T.);
#22068=ORIENTED_EDGE('',*,*,#15406,.T.);
#22069=ORIENTED_EDGE('',*,*,#15409,.T.);
#22070=ORIENTED_EDGE('',*,*,#15412,.T.);
#22071=ORIENTED_EDGE('',*,*,#15415,.T.);
#22072=ORIENTED_EDGE('',*,*,#15418,.T.);
#22073=ORIENTED_EDGE('',*,*,#15421,.T.);
#22074=ORIENTED_EDGE('',*,*,#15424,.T.);
#22075=ORIENTED_EDGE('',*,*,#15427,.T.);
#22076=ORIENTED_EDGE('',*,*,#15430,.T.);
#22077=ORIENTED_EDGE('',*,*,#15433,.T.);
#22078=ORIENTED_EDGE('',*,*,#15436,.T.);
#22079=ORIENTED_EDGE('',*,*,#15439,.T.);
#22080=ORIENTED_EDGE('',*,*,#15442,.T.);
#22081=ORIENTED_EDGE('',*,*,#15445,.T.);
#22082=ORIENTED_EDGE('',*,*,#15448,.T.);
#22083=ORIENTED_EDGE('',*,*,#15451,.T.);
#22084=ORIENTED_EDGE('',*,*,#15454,.T.);
#22085=ORIENTED_EDGE('',*,*,#15457,.T.);
#22086=ORIENTED_EDGE('',*,*,#15460,.T.);
#22087=ORIENTED_EDGE('',*,*,#15463,.T.);
#22088=ORIENTED_EDGE('',*,*,#15466,.T.);
#22089=ORIENTED_EDGE('',*,*,#15469,.T.);
#22090=ORIENTED_EDGE('',*,*,#15472,.T.);
#22091=ORIENTED_EDGE('',*,*,#15475,.T.);
#22092=ORIENTED_EDGE('',*,*,#15478,.T.);
#22093=ORIENTED_EDGE('',*,*,#15481,.T.);
#22094=ORIENTED_EDGE('',*,*,#15484,.T.);
#22095=ORIENTED_EDGE('',*,*,#15487,.T.);
#22096=ORIENTED_EDGE('',*,*,#15490,.T.);
#22097=ORIENTED_EDGE('',*,*,#15493,.T.);
#22098=ORIENTED_EDGE('',*,*,#15496,.T.);
#22099=ORIENTED_EDGE('',*,*,#15499,.T.);
#22100=ORIENTED_EDGE('',*,*,#15502,.T.);
#22101=ORIENTED_EDGE('',*,*,#15505,.T.);
#22102=ORIENTED_EDGE('',*,*,#15508,.T.);
#22103=ORIENTED_EDGE('',*,*,#15511,.T.);
#22104=ORIENTED_EDGE('',*,*,#15514,.T.);
#22105=ORIENTED_EDGE('',*,*,#15517,.T.);
#22106=ORIENTED_EDGE('',*,*,#15520,.T.);
#22107=ORIENTED_EDGE('',*,*,#15523,.T.);
#22108=ORIENTED_EDGE('',*,*,#15526,.T.);
#22109=ORIENTED_EDGE('',*,*,#15529,.T.);
#22110=ORIENTED_EDGE('',*,*,#15532,.T.);
#22111=ORIENTED_EDGE('',*,*,#15535,.T.);
#22112=ORIENTED_EDGE('',*,*,#15538,.T.);
#22113=ORIENTED_EDGE('',*,*,#15541,.T.);
#22114=ORIENTED_EDGE('',*,*,#15544,.T.);
#22115=ORIENTED_EDGE('',*,*,#15547,.T.);
#22116=ORIENTED_EDGE('',*,*,#15550,.T.);
#22117=ORIENTED_EDGE('',*,*,#15553,.T.);
#22118=ORIENTED_EDGE('',*,*,#15556,.T.);
#22119=ORIENTED_EDGE('',*,*,#15559,.T.);
#22120=ORIENTED_EDGE('',*,*,#15562,.T.);
#22121=ORIENTED_EDGE('',*,*,#15565,.T.);
#22122=ORIENTED_EDGE('',*,*,#15568,.T.);
#22123=ORIENTED_EDGE('',*,*,#15571,.T.);
#22124=ORIENTED_EDGE('',*,*,#15574,.T.);
#22125=ORIENTED_EDGE('',*,*,#15577,.T.);
#22126=ORIENTED_EDGE('',*,*,#15580,.T.);
#22127=ORIENTED_EDGE('',*,*,#15583,.T.);
#22128=ORIENTED_EDGE('',*,*,#15586,.T.);
#22129=ORIENTED_EDGE('',*,*,#15589,.T.);
#22130=ORIENTED_EDGE('',*,*,#15592,.T.);
#22131=ORIENTED_EDGE('',*,*,#15595,.T.);
#22132=ORIENTED_EDGE('',*,*,#15598,.T.);
#22133=ORIENTED_EDGE('',*,*,#15601,.T.);
#22134=ORIENTED_EDGE('',*,*,#15604,.T.);
#22135=ORIENTED_EDGE('',*,*,#15607,.T.);
#22136=ORIENTED_EDGE('',*,*,#15610,.T.);
#22137=ORIENTED_EDGE('',*,*,#15613,.T.);
#22138=ORIENTED_EDGE('',*,*,#15616,.T.);
#22139=ORIENTED_EDGE('',*,*,#15619,.T.);
#22140=ORIENTED_EDGE('',*,*,#15622,.T.);
#22141=ORIENTED_EDGE('',*,*,#15625,.T.);
#22142=ORIENTED_EDGE('',*,*,#15628,.T.);
#22143=ORIENTED_EDGE('',*,*,#15631,.T.);
#22144=ORIENTED_EDGE('',*,*,#15634,.T.);
#22145=ORIENTED_EDGE('',*,*,#15637,.T.);
#22146=ORIENTED_EDGE('',*,*,#15640,.T.);
#22147=ORIENTED_EDGE('',*,*,#15643,.T.);
#22148=ORIENTED_EDGE('',*,*,#15646,.T.);
#22149=ORIENTED_EDGE('',*,*,#15649,.T.);
#22150=ORIENTED_EDGE('',*,*,#15652,.T.);
#22151=ORIENTED_EDGE('',*,*,#15655,.T.);
#22152=ORIENTED_EDGE('',*,*,#15658,.T.);
#22153=ORIENTED_EDGE('',*,*,#15661,.T.);
#22154=ORIENTED_EDGE('',*,*,#15664,.T.);
#22155=ORIENTED_EDGE('',*,*,#15667,.T.);
#22156=ORIENTED_EDGE('',*,*,#15670,.T.);
#22157=ORIENTED_EDGE('',*,*,#15673,.T.);
#22158=ORIENTED_EDGE('',*,*,#15676,.T.);
#22159=ORIENTED_EDGE('',*,*,#15679,.T.);
#22160=ORIENTED_EDGE('',*,*,#15682,.T.);
#22161=ORIENTED_EDGE('',*,*,#15685,.T.);
#22162=ORIENTED_EDGE('',*,*,#15688,.T.);
#22163=ORIENTED_EDGE('',*,*,#15691,.T.);
#22164=ORIENTED_EDGE('',*,*,#15694,.T.);
#22165=ORIENTED_EDGE('',*,*,#15697,.T.);
#22166=ORIENTED_EDGE('',*,*,#15700,.T.);
#22167=ORIENTED_EDGE('',*,*,#15703,.T.);
#22168=ORIENTED_EDGE('',*,*,#15706,.T.);
#22169=ORIENTED_EDGE('',*,*,#15709,.T.);
#22170=ORIENTED_EDGE('',*,*,#15712,.T.);
#22171=ORIENTED_EDGE('',*,*,#15715,.T.);
#22172=ORIENTED_EDGE('',*,*,#15718,.T.);
#22173=ORIENTED_EDGE('',*,*,#15721,.T.);
#22174=ORIENTED_EDGE('',*,*,#15724,.T.);
#22175=ORIENTED_EDGE('',*,*,#15727,.T.);
#22176=ORIENTED_EDGE('',*,*,#15730,.T.);
#22177=ORIENTED_EDGE('',*,*,#15733,.T.);
#22178=ORIENTED_EDGE('',*,*,#15736,.T.);
#22179=ORIENTED_EDGE('',*,*,#15739,.T.);
#22180=ORIENTED_EDGE('',*,*,#15742,.T.);
#22181=ORIENTED_EDGE('',*,*,#15745,.T.);
#22182=ORIENTED_EDGE('',*,*,#15748,.T.);
#22183=ORIENTED_EDGE('',*,*,#15751,.T.);
#22184=ORIENTED_EDGE('',*,*,#15754,.T.);
#22185=ORIENTED_EDGE('',*,*,#15757,.T.);
#22186=ORIENTED_EDGE('',*,*,#15760,.T.);
#22187=ORIENTED_EDGE('',*,*,#15763,.T.);
#22188=ORIENTED_EDGE('',*,*,#15766,.T.);
#22189=ORIENTED_EDGE('',*,*,#15769,.T.);
#22190=ORIENTED_EDGE('',*,*,#15772,.T.);
#22191=ORIENTED_EDGE('',*,*,#15775,.T.);
#22192=ORIENTED_EDGE('',*,*,#15778,.T.);
#22193=ORIENTED_EDGE('',*,*,#15781,.T.);
#22194=ORIENTED_EDGE('',*,*,#15784,.T.);
#22195=ORIENTED_EDGE('',*,*,#15787,.T.);
#22196=ORIENTED_EDGE('',*,*,#15790,.T.);
#22197=ORIENTED_EDGE('',*,*,#15793,.T.);
#22198=ORIENTED_EDGE('',*,*,#15796,.T.);
#22199=ORIENTED_EDGE('',*,*,#15799,.T.);
#22200=ORIENTED_EDGE('',*,*,#15802,.T.);
#22201=ORIENTED_EDGE('',*,*,#15805,.T.);
#22202=ORIENTED_EDGE('',*,*,#15808,.T.);
#22203=ORIENTED_EDGE('',*,*,#15811,.T.);
#22204=ORIENTED_EDGE('',*,*,#15814,.T.);
#22205=ORIENTED_EDGE('',*,*,#15817,.T.);
#22206=ORIENTED_EDGE('',*,*,#15820,.T.);
#22207=ORIENTED_EDGE('',*,*,#15823,.T.);
#22208=ORIENTED_EDGE('',*,*,#15826,.T.);
#22209=ORIENTED_EDGE('',*,*,#15829,.T.);
#22210=ORIENTED_EDGE('',*,*,#15832,.T.);
#22211=ORIENTED_EDGE('',*,*,#15835,.T.);
#22212=ORIENTED_EDGE('',*,*,#15838,.T.);
#22213=ORIENTED_EDGE('',*,*,#15841,.T.);
#22214=ORIENTED_EDGE('',*,*,#15844,.T.);
#22215=ORIENTED_EDGE('',*,*,#15847,.T.);
#22216=ORIENTED_EDGE('',*,*,#15850,.T.);
#22217=ORIENTED_EDGE('',*,*,#15853,.T.);
#22218=ORIENTED_EDGE('',*,*,#15856,.T.);
#22219=ORIENTED_EDGE('',*,*,#15859,.T.);
#22220=ORIENTED_EDGE('',*,*,#15862,.T.);
#22221=ORIENTED_EDGE('',*,*,#15865,.T.);
#22222=ORIENTED_EDGE('',*,*,#15868,.T.);
#22223=ORIENTED_EDGE('',*,*,#15871,.T.);
#22224=ORIENTED_EDGE('',*,*,#15874,.T.);
#22225=ORIENTED_EDGE('',*,*,#15877,.T.);
#22226=ORIENTED_EDGE('',*,*,#15880,.T.);
#22227=ORIENTED_EDGE('',*,*,#15883,.T.);
#22228=ORIENTED_EDGE('',*,*,#15886,.T.);
#22229=ORIENTED_EDGE('',*,*,#15889,.T.);
#22230=ORIENTED_EDGE('',*,*,#15892,.T.);
#22231=ORIENTED_EDGE('',*,*,#15895,.T.);
#22232=ORIENTED_EDGE('',*,*,#15898,.T.);
#22233=ORIENTED_EDGE('',*,*,#15901,.T.);
#22234=ORIENTED_EDGE('',*,*,#15904,.T.);
#22235=ORIENTED_EDGE('',*,*,#15907,.T.);
#22236=ORIENTED_EDGE('',*,*,#15910,.T.);
#22237=ORIENTED_EDGE('',*,*,#15913,.T.);
#22238=ORIENTED_EDGE('',*,*,#15916,.T.);
#22239=ORIENTED_EDGE('',*,*,#15919,.T.);
#22240=ORIENTED_EDGE('',*,*,#15922,.T.);
#22241=ORIENTED_EDGE('',*,*,#15925,.T.);
#22242=ORIENTED_EDGE('',*,*,#15928,.T.);
#22243=ORIENTED_EDGE('',*,*,#15931,.T.);
#22244=ORIENTED_EDGE('',*,*,#15934,.T.);
#22245=ORIENTED_EDGE('',*,*,#15937,.T.);
#22246=ORIENTED_EDGE('',*,*,#15940,.T.);
#22247=ORIENTED_EDGE('',*,*,#15943,.T.);
#22248=ORIENTED_EDGE('',*,*,#15946,.T.);
#22249=ORIENTED_EDGE('',*,*,#15949,.T.);
#22250=ORIENTED_EDGE('',*,*,#15952,.T.);
#22251=ORIENTED_EDGE('',*,*,#15955,.T.);
#22252=ORIENTED_EDGE('',*,*,#15958,.T.);
#22253=ORIENTED_EDGE('',*,*,#15961,.T.);
#22254=ORIENTED_EDGE('',*,*,#15964,.T.);
#22255=ORIENTED_EDGE('',*,*,#15967,.T.);
#22256=ORIENTED_EDGE('',*,*,#15970,.T.);
#22257=ORIENTED_EDGE('',*,*,#15973,.T.);
#22258=ORIENTED_EDGE('',*,*,#15976,.T.);
#22259=ORIENTED_EDGE('',*,*,#15979,.T.);
#22260=ORIENTED_EDGE('',*,*,#15982,.T.);
#22261=ORIENTED_EDGE('',*,*,#15985,.T.);
#22262=ORIENTED_EDGE('',*,*,#15988,.T.);
#22263=ORIENTED_EDGE('',*,*,#15991,.T.);
#22264=ORIENTED_EDGE('',*,*,#15994,.T.);
#22265=ORIENTED_EDGE('',*,*,#15997,.T.);
#22266=ORIENTED_EDGE('',*,*,#16000,.T.);
#22267=ORIENTED_EDGE('',*,*,#15127,.F.);
#22268=ORIENTED_EDGE('',*,*,#15129,.F.);
#22269=ORIENTED_EDGE('',*,*,#15131,.F.);
#22270=ORIENTED_EDGE('',*,*,#15133,.F.);
#22271=ORIENTED_EDGE('',*,*,#15135,.F.);
#22272=ORIENTED_EDGE('',*,*,#15165,.T.);
#22273=ORIENTED_EDGE('',*,*,#15162,.T.);
#22274=ORIENTED_EDGE('',*,*,#15159,.T.);
#22275=ORIENTED_EDGE('',*,*,#15156,.T.);
#22276=ORIENTED_EDGE('',*,*,#15153,.T.);
#22277=ORIENTED_EDGE('',*,*,#15150,.T.);
#22278=ORIENTED_EDGE('',*,*,#15147,.T.);
#22279=ORIENTED_EDGE('',*,*,#15144,.T.);
#22280=ORIENTED_EDGE('',*,*,#15141,.T.);
#22281=ORIENTED_EDGE('',*,*,#15138,.T.);
#25514=CONICAL_SURFACE('',#28002,4.6625,0.785398163397448);
#25515=CONICAL_SURFACE('',#28006,4.6625,0.785398163397448);
#25516=CONICAL_SURFACE('',#28018,4.6625,0.785398163397448);
#25517=CONICAL_SURFACE('',#28021,4.6625,0.785398163397448);
#26090=ADVANCED_FACE('',(#2897),#1423,.T.);
#26091=ADVANCED_FACE('',(#2898),#25514,.T.);
#26092=ADVANCED_FACE('',(#2899),#1424,.T.);
#26093=ADVANCED_FACE('',(#2900),#25515,.T.);
#26094=ADVANCED_FACE('',(#2901),#1425,.T.);
#26095=ADVANCED_FACE('',(#2902),#1426,.T.);
#26096=ADVANCED_FACE('',(#2903),#2282,.T.);
#26097=ADVANCED_FACE('',(#2904),#1427,.T.);
#26098=ADVANCED_FACE('',(#2905),#2283,.T.);
#26099=ADVANCED_FACE('',(#2906),#1428,.T.);
#26100=ADVANCED_FACE('',(#2907),#1429,.T.);
#26101=ADVANCED_FACE('',(#2908),#25516,.T.);
#26102=ADVANCED_FACE('',(#2909),#1430,.T.);
#26103=ADVANCED_FACE('',(#2910),#25517,.T.);
#26104=ADVANCED_FACE('',(#2911),#1431,.T.);
#26105=ADVANCED_FACE('',(#2912),#2284,.F.);
#26106=ADVANCED_FACE('',(#2913),#2285,.F.);
#26107=ADVANCED_FACE('',(#2914),#2286,.F.);
#26108=ADVANCED_FACE('',(#2915),#2287,.F.);
#26109=ADVANCED_FACE('',(#2916),#2288,.F.);
#26110=ADVANCED_FACE('',(#2917),#2289,.F.);
#26111=ADVANCED_FACE('',(#2918),#2290,.F.);
#26112=ADVANCED_FACE('',(#2919),#2291,.F.);
#26113=ADVANCED_FACE('',(#2920),#2292,.F.);
#26114=ADVANCED_FACE('',(#2921),#2293,.F.);
#26115=ADVANCED_FACE('',(#2922),#1432,.T.);
#26116=ADVANCED_FACE('',(#2923),#1433,.T.);
#26117=ADVANCED_FACE('',(#2924),#1434,.T.);
#26118=ADVANCED_FACE('',(#2925),#1435,.T.);
#26119=ADVANCED_FACE('',(#2926),#1436,.T.);
#26120=ADVANCED_FACE('',(#2927),#1437,.T.);
#26121=ADVANCED_FACE('',(#2928),#1438,.T.);
#26122=ADVANCED_FACE('',(#2929),#1439,.T.);
#26123=ADVANCED_FACE('',(#2930),#1440,.T.);
#26124=ADVANCED_FACE('',(#2931),#1441,.T.);
#26125=ADVANCED_FACE('',(#2932),#1442,.T.);
#26126=ADVANCED_FACE('',(#2933),#1443,.T.);
#26127=ADVANCED_FACE('',(#2934),#1444,.T.);
#26128=ADVANCED_FACE('',(#2935),#1445,.T.);
#26129=ADVANCED_FACE('',(#2936),#1446,.T.);
#26130=ADVANCED_FACE('',(#2937),#1447,.T.);
#26131=ADVANCED_FACE('',(#2938),#1448,.T.);
#26132=ADVANCED_FACE('',(#2939),#1449,.T.);
#26133=ADVANCED_FACE('',(#2940),#1450,.T.);
#26134=ADVANCED_FACE('',(#2941),#1451,.T.);
#26135=ADVANCED_FACE('',(#2942),#1452,.T.);
#26136=ADVANCED_FACE('',(#2943),#1453,.T.);
#26137=ADVANCED_FACE('',(#2944),#1454,.T.);
#26138=ADVANCED_FACE('',(#2945),#1455,.T.);
#26139=ADVANCED_FACE('',(#2946),#1456,.T.);
#26140=ADVANCED_FACE('',(#2947),#1457,.T.);
#26141=ADVANCED_FACE('',(#2948),#1458,.T.);
#26142=ADVANCED_FACE('',(#2949),#1459,.T.);
#26143=ADVANCED_FACE('',(#2950),#1460,.T.);
#26144=ADVANCED_FACE('',(#2951),#1461,.T.);
#26145=ADVANCED_FACE('',(#2952),#1462,.T.);
#26146=ADVANCED_FACE('',(#2953),#1463,.T.);
#26147=ADVANCED_FACE('',(#2954),#1464,.T.);
#26148=ADVANCED_FACE('',(#2955),#1465,.T.);
#26149=ADVANCED_FACE('',(#2956),#1466,.T.);
#26150=ADVANCED_FACE('',(#2957),#1467,.T.);
#26151=ADVANCED_FACE('',(#2958),#1468,.T.);
#26152=ADVANCED_FACE('',(#2959),#1469,.T.);
#26153=ADVANCED_FACE('',(#2960),#1470,.T.);
#26154=ADVANCED_FACE('',(#2961),#1471,.T.);
#26155=ADVANCED_FACE('',(#2962),#1472,.T.);
#26156=ADVANCED_FACE('',(#2963),#1473,.T.);
#26157=ADVANCED_FACE('',(#2964),#1474,.T.);
#26158=ADVANCED_FACE('',(#2965),#1475,.T.);
#26159=ADVANCED_FACE('',(#2966),#1476,.T.);
#26160=ADVANCED_FACE('',(#2967),#1477,.T.);
#26161=ADVANCED_FACE('',(#2968),#1478,.T.);
#26162=ADVANCED_FACE('',(#2969),#1479,.T.);
#26163=ADVANCED_FACE('',(#2970),#1480,.T.);
#26164=ADVANCED_FACE('',(#2971),#1481,.T.);
#26165=ADVANCED_FACE('',(#2972),#1482,.T.);
#26166=ADVANCED_FACE('',(#2973),#1483,.T.);
#26167=ADVANCED_FACE('',(#2974),#1484,.T.);
#26168=ADVANCED_FACE('',(#2975),#1485,.T.);
#26169=ADVANCED_FACE('',(#2976),#1486,.T.);
#26170=ADVANCED_FACE('',(#2977),#1487,.T.);
#26171=ADVANCED_FACE('',(#2978),#1488,.T.);
#26172=ADVANCED_FACE('',(#2979),#1489,.T.);
#26173=ADVANCED_FACE('',(#2980),#1490,.T.);
#26174=ADVANCED_FACE('',(#2981),#1491,.T.);
#26175=ADVANCED_FACE('',(#2982),#1492,.T.);
#26176=ADVANCED_FACE('',(#2983),#1493,.T.);
#26177=ADVANCED_FACE('',(#2984),#1494,.T.);
#26178=ADVANCED_FACE('',(#2985),#1495,.T.);
#26179=ADVANCED_FACE('',(#2986),#1496,.T.);
#26180=ADVANCED_FACE('',(#2987),#1497,.T.);
#26181=ADVANCED_FACE('',(#2988),#1498,.T.);
#26182=ADVANCED_FACE('',(#2989),#1499,.T.);
#26183=ADVANCED_FACE('',(#2990),#1500,.T.);
#26184=ADVANCED_FACE('',(#2991),#1501,.T.);
#26185=ADVANCED_FACE('',(#2992),#1502,.T.);
#26186=ADVANCED_FACE('',(#2993),#1503,.T.);
#26187=ADVANCED_FACE('',(#2994),#1504,.T.);
#26188=ADVANCED_FACE('',(#2995),#1505,.T.);
#26189=ADVANCED_FACE('',(#2996),#1506,.T.);
#26190=ADVANCED_FACE('',(#2997),#1507,.T.);
#26191=ADVANCED_FACE('',(#2998),#1508,.T.);
#26192=ADVANCED_FACE('',(#2999),#1509,.T.);
#26193=ADVANCED_FACE('',(#3000),#1510,.T.);
#26194=ADVANCED_FACE('',(#3001),#1511,.T.);
#26195=ADVANCED_FACE('',(#3002),#1512,.T.);
#26196=ADVANCED_FACE('',(#3003),#1513,.T.);
#26197=ADVANCED_FACE('',(#3004),#1514,.T.);
#26198=ADVANCED_FACE('',(#3005),#1515,.T.);
#26199=ADVANCED_FACE('',(#3006),#1516,.T.);
#26200=ADVANCED_FACE('',(#3007),#1517,.T.);
#26201=ADVANCED_FACE('',(#3008),#1518,.T.);
#26202=ADVANCED_FACE('',(#3009),#1519,.T.);
#26203=ADVANCED_FACE('',(#3010),#1520,.T.);
#26204=ADVANCED_FACE('',(#3011),#1521,.T.);
#26205=ADVANCED_FACE('',(#3012),#1522,.T.);
#26206=ADVANCED_FACE('',(#3013),#1523,.T.);
#26207=ADVANCED_FACE('',(#3014),#1524,.T.);
#26208=ADVANCED_FACE('',(#3015),#1525,.T.);
#26209=ADVANCED_FACE('',(#3016),#1526,.T.);
#26210=ADVANCED_FACE('',(#3017),#1527,.T.);
#26211=ADVANCED_FACE('',(#3018),#1528,.T.);
#26212=ADVANCED_FACE('',(#3019),#1529,.T.);
#26213=ADVANCED_FACE('',(#3020),#1530,.T.);
#26214=ADVANCED_FACE('',(#3021),#1531,.T.);
#26215=ADVANCED_FACE('',(#3022),#1532,.T.);
#26216=ADVANCED_FACE('',(#3023),#1533,.T.);
#26217=ADVANCED_FACE('',(#3024),#1534,.T.);
#26218=ADVANCED_FACE('',(#3025),#1535,.T.);
#26219=ADVANCED_FACE('',(#3026),#1536,.T.);
#26220=ADVANCED_FACE('',(#3027),#1537,.T.);
#26221=ADVANCED_FACE('',(#3028),#1538,.T.);
#26222=ADVANCED_FACE('',(#3029),#1539,.T.);
#26223=ADVANCED_FACE('',(#3030),#1540,.T.);
#26224=ADVANCED_FACE('',(#3031),#1541,.T.);
#26225=ADVANCED_FACE('',(#3032),#1542,.T.);
#26226=ADVANCED_FACE('',(#3033),#1543,.T.);
#26227=ADVANCED_FACE('',(#3034),#1544,.T.);
#26228=ADVANCED_FACE('',(#3035),#1545,.T.);
#26229=ADVANCED_FACE('',(#3036),#1546,.T.);
#26230=ADVANCED_FACE('',(#3037),#1547,.T.);
#26231=ADVANCED_FACE('',(#3038),#1548,.T.);
#26232=ADVANCED_FACE('',(#3039),#1549,.T.);
#26233=ADVANCED_FACE('',(#3040),#1550,.T.);
#26234=ADVANCED_FACE('',(#3041),#1551,.T.);
#26235=ADVANCED_FACE('',(#3042),#1552,.T.);
#26236=ADVANCED_FACE('',(#3043),#1553,.T.);
#26237=ADVANCED_FACE('',(#3044),#1554,.T.);
#26238=ADVANCED_FACE('',(#3045),#1555,.T.);
#26239=ADVANCED_FACE('',(#3046),#1556,.T.);
#26240=ADVANCED_FACE('',(#3047),#1557,.T.);
#26241=ADVANCED_FACE('',(#3048),#1558,.T.);
#26242=ADVANCED_FACE('',(#3049),#1559,.T.);
#26243=ADVANCED_FACE('',(#3050),#1560,.T.);
#26244=ADVANCED_FACE('',(#3051),#1561,.T.);
#26245=ADVANCED_FACE('',(#3052),#1562,.T.);
#26246=ADVANCED_FACE('',(#3053),#1563,.T.);
#26247=ADVANCED_FACE('',(#3054),#1564,.T.);
#26248=ADVANCED_FACE('',(#3055),#1565,.T.);
#26249=ADVANCED_FACE('',(#3056),#1566,.T.);
#26250=ADVANCED_FACE('',(#3057),#1567,.T.);
#26251=ADVANCED_FACE('',(#3058),#1568,.T.);
#26252=ADVANCED_FACE('',(#3059),#1569,.T.);
#26253=ADVANCED_FACE('',(#3060),#1570,.T.);
#26254=ADVANCED_FACE('',(#3061),#1571,.T.);
#26255=ADVANCED_FACE('',(#3062),#1572,.T.);
#26256=ADVANCED_FACE('',(#3063),#1573,.T.);
#26257=ADVANCED_FACE('',(#3064),#1574,.T.);
#26258=ADVANCED_FACE('',(#3065),#1575,.T.);
#26259=ADVANCED_FACE('',(#3066),#1576,.T.);
#26260=ADVANCED_FACE('',(#3067),#1577,.T.);
#26261=ADVANCED_FACE('',(#3068),#1578,.T.);
#26262=ADVANCED_FACE('',(#3069),#1579,.T.);
#26263=ADVANCED_FACE('',(#3070),#1580,.T.);
#26264=ADVANCED_FACE('',(#3071),#1581,.T.);
#26265=ADVANCED_FACE('',(#3072),#1582,.T.);
#26266=ADVANCED_FACE('',(#3073),#1583,.T.);
#26267=ADVANCED_FACE('',(#3074),#1584,.T.);
#26268=ADVANCED_FACE('',(#3075),#1585,.T.);
#26269=ADVANCED_FACE('',(#3076),#1586,.T.);
#26270=ADVANCED_FACE('',(#3077),#1587,.T.);
#26271=ADVANCED_FACE('',(#3078),#1588,.T.);
#26272=ADVANCED_FACE('',(#3079),#1589,.T.);
#26273=ADVANCED_FACE('',(#3080),#1590,.T.);
#26274=ADVANCED_FACE('',(#3081),#1591,.T.);
#26275=ADVANCED_FACE('',(#3082),#1592,.T.);
#26276=ADVANCED_FACE('',(#3083),#1593,.T.);
#26277=ADVANCED_FACE('',(#3084),#1594,.T.);
#26278=ADVANCED_FACE('',(#3085),#1595,.T.);
#26279=ADVANCED_FACE('',(#3086),#1596,.T.);
#26280=ADVANCED_FACE('',(#3087),#1597,.T.);
#26281=ADVANCED_FACE('',(#3088),#1598,.T.);
#26282=ADVANCED_FACE('',(#3089),#1599,.T.);
#26283=ADVANCED_FACE('',(#3090),#1600,.T.);
#26284=ADVANCED_FACE('',(#3091),#1601,.T.);
#26285=ADVANCED_FACE('',(#3092),#1602,.T.);
#26286=ADVANCED_FACE('',(#3093),#1603,.T.);
#26287=ADVANCED_FACE('',(#3094),#1604,.T.);
#26288=ADVANCED_FACE('',(#3095),#1605,.T.);
#26289=ADVANCED_FACE('',(#3096),#1606,.T.);
#26290=ADVANCED_FACE('',(#3097),#1607,.T.);
#26291=ADVANCED_FACE('',(#3098),#1608,.T.);
#26292=ADVANCED_FACE('',(#3099),#1609,.T.);
#26293=ADVANCED_FACE('',(#3100),#1610,.T.);
#26294=ADVANCED_FACE('',(#3101),#1611,.T.);
#26295=ADVANCED_FACE('',(#3102),#1612,.T.);
#26296=ADVANCED_FACE('',(#3103),#1613,.T.);
#26297=ADVANCED_FACE('',(#3104),#1614,.T.);
#26298=ADVANCED_FACE('',(#3105),#1615,.T.);
#26299=ADVANCED_FACE('',(#3106),#1616,.T.);
#26300=ADVANCED_FACE('',(#3107),#1617,.T.);
#26301=ADVANCED_FACE('',(#3108),#1618,.T.);
#26302=ADVANCED_FACE('',(#3109),#1619,.T.);
#26303=ADVANCED_FACE('',(#3110),#1620,.T.);
#26304=ADVANCED_FACE('',(#3111),#1621,.T.);
#26305=ADVANCED_FACE('',(#3112),#1622,.T.);
#26306=ADVANCED_FACE('',(#3113),#1623,.T.);
#26307=ADVANCED_FACE('',(#3114),#1624,.T.);
#26308=ADVANCED_FACE('',(#3115),#1625,.T.);
#26309=ADVANCED_FACE('',(#3116),#1626,.T.);
#26310=ADVANCED_FACE('',(#3117),#1627,.T.);
#26311=ADVANCED_FACE('',(#3118),#1628,.T.);
#26312=ADVANCED_FACE('',(#3119),#1629,.T.);
#26313=ADVANCED_FACE('',(#3120),#1630,.T.);
#26314=ADVANCED_FACE('',(#3121),#1631,.T.);
#26315=ADVANCED_FACE('',(#3122),#1632,.T.);
#26316=ADVANCED_FACE('',(#3123),#1633,.T.);
#26317=ADVANCED_FACE('',(#3124),#1634,.T.);
#26318=ADVANCED_FACE('',(#3125),#1635,.T.);
#26319=ADVANCED_FACE('',(#3126),#1636,.T.);
#26320=ADVANCED_FACE('',(#3127),#1637,.T.);
#26321=ADVANCED_FACE('',(#3128),#1638,.T.);
#26322=ADVANCED_FACE('',(#3129),#1639,.T.);
#26323=ADVANCED_FACE('',(#3130),#1640,.T.);
#26324=ADVANCED_FACE('',(#3131),#1641,.T.);
#26325=ADVANCED_FACE('',(#3132),#1642,.T.);
#26326=ADVANCED_FACE('',(#3133),#1643,.T.);
#26327=ADVANCED_FACE('',(#3134),#1644,.T.);
#26328=ADVANCED_FACE('',(#3135),#1645,.T.);
#26329=ADVANCED_FACE('',(#3136),#1646,.T.);
#26330=ADVANCED_FACE('',(#3137),#1647,.T.);
#26331=ADVANCED_FACE('',(#3138),#1648,.T.);
#26332=ADVANCED_FACE('',(#3139),#1649,.T.);
#26333=ADVANCED_FACE('',(#3140),#1650,.T.);
#26334=ADVANCED_FACE('',(#3141),#1651,.T.);
#26335=ADVANCED_FACE('',(#3142),#1652,.T.);
#26336=ADVANCED_FACE('',(#3143),#1653,.T.);
#26337=ADVANCED_FACE('',(#3144),#1654,.T.);
#26338=ADVANCED_FACE('',(#3145),#1655,.T.);
#26339=ADVANCED_FACE('',(#3146),#1656,.T.);
#26340=ADVANCED_FACE('',(#3147),#1657,.T.);
#26341=ADVANCED_FACE('',(#3148),#1658,.T.);
#26342=ADVANCED_FACE('',(#3149),#1659,.T.);
#26343=ADVANCED_FACE('',(#3150),#1660,.T.);
#26344=ADVANCED_FACE('',(#3151),#1661,.T.);
#26345=ADVANCED_FACE('',(#3152),#1662,.T.);
#26346=ADVANCED_FACE('',(#3153),#1663,.T.);
#26347=ADVANCED_FACE('',(#3154),#1664,.T.);
#26348=ADVANCED_FACE('',(#3155),#1665,.T.);
#26349=ADVANCED_FACE('',(#3156),#1666,.T.);
#26350=ADVANCED_FACE('',(#3157),#1667,.T.);
#26351=ADVANCED_FACE('',(#3158),#1668,.T.);
#26352=ADVANCED_FACE('',(#3159),#1669,.T.);
#26353=ADVANCED_FACE('',(#3160),#1670,.T.);
#26354=ADVANCED_FACE('',(#3161),#1671,.T.);
#26355=ADVANCED_FACE('',(#3162),#1672,.T.);
#26356=ADVANCED_FACE('',(#3163),#1673,.T.);
#26357=ADVANCED_FACE('',(#3164),#1674,.T.);
#26358=ADVANCED_FACE('',(#3165),#1675,.T.);
#26359=ADVANCED_FACE('',(#3166),#1676,.T.);
#26360=ADVANCED_FACE('',(#3167),#1677,.T.);
#26361=ADVANCED_FACE('',(#3168),#1678,.T.);
#26362=ADVANCED_FACE('',(#3169),#1679,.T.);
#26363=ADVANCED_FACE('',(#3170),#1680,.T.);
#26364=ADVANCED_FACE('',(#3171),#1681,.T.);
#26365=ADVANCED_FACE('',(#3172),#1682,.T.);
#26366=ADVANCED_FACE('',(#3173),#1683,.T.);
#26367=ADVANCED_FACE('',(#3174),#1684,.T.);
#26368=ADVANCED_FACE('',(#3175),#1685,.T.);
#26369=ADVANCED_FACE('',(#3176),#1686,.T.);
#26370=ADVANCED_FACE('',(#3177),#1687,.T.);
#26371=ADVANCED_FACE('',(#3178),#1688,.T.);
#26372=ADVANCED_FACE('',(#3179),#1689,.T.);
#26373=ADVANCED_FACE('',(#3180),#1690,.T.);
#26374=ADVANCED_FACE('',(#3181),#1691,.T.);
#26375=ADVANCED_FACE('',(#3182),#1692,.T.);
#26376=ADVANCED_FACE('',(#3183),#1693,.T.);
#26377=ADVANCED_FACE('',(#3184),#1694,.T.);
#26378=ADVANCED_FACE('',(#3185),#1695,.T.);
#26379=ADVANCED_FACE('',(#3186),#1696,.T.);
#26380=ADVANCED_FACE('',(#3187),#1697,.T.);
#26381=ADVANCED_FACE('',(#3188),#1698,.T.);
#26382=ADVANCED_FACE('',(#3189),#1699,.T.);
#26383=ADVANCED_FACE('',(#3190),#1700,.T.);
#26384=ADVANCED_FACE('',(#3191),#1701,.T.);
#26385=ADVANCED_FACE('',(#3192),#1702,.T.);
#26386=ADVANCED_FACE('',(#3193),#1703,.T.);
#26387=ADVANCED_FACE('',(#3194),#1704,.T.);
#26388=ADVANCED_FACE('',(#3195),#1705,.T.);
#26389=ADVANCED_FACE('',(#3196),#1706,.T.);
#26390=ADVANCED_FACE('',(#3197),#1707,.T.);
#26391=ADVANCED_FACE('',(#3198),#1708,.T.);
#26392=ADVANCED_FACE('',(#3199),#1709,.T.);
#26393=ADVANCED_FACE('',(#3200),#1710,.T.);
#26394=ADVANCED_FACE('',(#3201,#1061,#1062,#1063,#1064,#1065,#1066,#1067,
#1068,#1069,#1070),#1711,.T.);
#26395=ADVANCED_FACE('',(#3202,#1071,#1072,#1073,#1074,#1075,#1076,#1077,
#1078,#1079,#1080),#1712,.F.);
#26935=CLOSED_SHELL('',(#26090,#26091,#26092,#26093,#26094,#26095,#26096,
#26097,#26098,#26099,#26100,#26101,#26102,#26103,#26104,#26105,#26106,#26107,
#26108,#26109,#26110,#26111,#26112,#26113,#26114,#26115,#26116,#26117,#26118,
#26119,#26120,#26121,#26122,#26123,#26124,#26125,#26126,#26127,#26128,#26129,
#26130,#26131,#26132,#26133,#26134,#26135,#26136,#26137,#26138,#26139,#26140,
#26141,#26142,#26143,#26144,#26145,#26146,#26147,#26148,#26149,#26150,#26151,
#26152,#26153,#26154,#26155,#26156,#26157,#26158,#26159,#26160,#26161,#26162,
#26163,#26164,#26165,#26166,#26167,#26168,#26169,#26170,#26171,#26172,#26173,
#26174,#26175,#26176,#26177,#26178,#26179,#26180,#26181,#26182,#26183,#26184,
#26185,#26186,#26187,#26188,#26189,#26190,#26191,#26192,#26193,#26194,#26195,
#26196,#26197,#26198,#26199,#26200,#26201,#26202,#26203,#26204,#26205,#26206,
#26207,#26208,#26209,#26210,#26211,#26212,#26213,#26214,#26215,#26216,#26217,
#26218,#26219,#26220,#26221,#26222,#26223,#26224,#26225,#26226,#26227,#26228,
#26229,#26230,#26231,#26232,#26233,#26234,#26235,#26236,#26237,#26238,#26239,
#26240,#26241,#26242,#26243,#26244,#26245,#26246,#26247,#26248,#26249,#26250,
#26251,#26252,#26253,#26254,#26255,#26256,#26257,#26258,#26259,#26260,#26261,
#26262,#26263,#26264,#26265,#26266,#26267,#26268,#26269,#26270,#26271,#26272,
#26273,#26274,#26275,#26276,#26277,#26278,#26279,#26280,#26281,#26282,#26283,
#26284,#26285,#26286,#26287,#26288,#26289,#26290,#26291,#26292,#26293,#26294,
#26295,#26296,#26297,#26298,#26299,#26300,#26301,#26302,#26303,#26304,#26305,
#26306,#26307,#26308,#26309,#26310,#26311,#26312,#26313,#26314,#26315,#26316,
#26317,#26318,#26319,#26320,#26321,#26322,#26323,#26324,#26325,#26326,#26327,
#26328,#26329,#26330,#26331,#26332,#26333,#26334,#26335,#26336,#26337,#26338,
#26339,#26340,#26341,#26342,#26343,#26344,#26345,#26346,#26347,#26348,#26349,
#26350,#26351,#26352,#26353,#26354,#26355,#26356,#26357,#26358,#26359,#26360,
#26361,#26362,#26363,#26364,#26365,#26366,#26367,#26368,#26369,#26370,#26371,
#26372,#26373,#26374,#26375,#26376,#26377,#26378,#26379,#26380,#26381,#26382,
#26383,#26384,#26385,#26386,#26387,#26388,#26389,#26390,#26391,#26392,#26393,
#26394,#26395));
#28000=AXIS2_PLACEMENT_3D('',#50940,#31897,#31898);
#28001=AXIS2_PLACEMENT_3D('',#50941,#31899,#31900);
#28002=AXIS2_PLACEMENT_3D('',#50950,#31905,#31906);
#28003=AXIS2_PLACEMENT_3D('',#50954,#31908,#31909);
#28004=AXIS2_PLACEMENT_3D('',#50955,#31910,#31911);
#28005=AXIS2_PLACEMENT_3D('',#50956,#31912,#31913);
#28006=AXIS2_PLACEMENT_3D('',#50962,#31917,#31918);
#28007=AXIS2_PLACEMENT_3D('',#50966,#31920,#31921);
#28008=AXIS2_PLACEMENT_3D('',#50967,#31922,#31923);
#28009=AXIS2_PLACEMENT_3D('',#50968,#31924,#31925);
#28010=AXIS2_PLACEMENT_3D('',#50974,#31929,#31930);
#28011=AXIS2_PLACEMENT_3D('',#50980,#31934,#31935);
#28012=AXIS2_PLACEMENT_3D('',#50983,#31937,#31938);
#28013=AXIS2_PLACEMENT_3D('',#50984,#31939,#31940);
#28014=AXIS2_PLACEMENT_3D('',#50988,#31943,#31944);
#28015=AXIS2_PLACEMENT_3D('',#50991,#31946,#31947);
#28016=AXIS2_PLACEMENT_3D('',#50992,#31948,#31949);
#28017=AXIS2_PLACEMENT_3D('',#50996,#31952,#31953);
#28018=AXIS2_PLACEMENT_3D('',#51002,#31957,#31958);
#28019=AXIS2_PLACEMENT_3D('',#51005,#31960,#31961);
#28020=AXIS2_PLACEMENT_3D('',#51006,#31962,#31963);
#28021=AXIS2_PLACEMENT_3D('',#51010,#31966,#31967);
#28022=AXIS2_PLACEMENT_3D('',#51013,#31969,#31970);
#28023=AXIS2_PLACEMENT_3D('',#51014,#31971,#31972);
#28024=AXIS2_PLACEMENT_3D('',#51018,#31975,#31976);
#28025=AXIS2_PLACEMENT_3D('',#51020,#31977,#31978);
#28026=AXIS2_PLACEMENT_3D('',#51023,#31980,#31981);
#28027=AXIS2_PLACEMENT_3D('',#51024,#31982,#31983);
#28028=AXIS2_PLACEMENT_3D('',#51026,#31984,#31985);
#28029=AXIS2_PLACEMENT_3D('',#51029,#31987,#31988);
#28030=AXIS2_PLACEMENT_3D('',#51030,#31989,#31990);
#28031=AXIS2_PLACEMENT_3D('',#51032,#31991,#31992);
#28032=AXIS2_PLACEMENT_3D('',#51035,#31994,#31995);
#28033=AXIS2_PLACEMENT_3D('',#51036,#31996,#31997);
#28034=AXIS2_PLACEMENT_3D('',#51038,#31998,#31999);
#28035=AXIS2_PLACEMENT_3D('',#51041,#32001,#32002);
#28036=AXIS2_PLACEMENT_3D('',#51042,#32003,#32004);
#28037=AXIS2_PLACEMENT_3D('',#51044,#32005,#32006);
#28038=AXIS2_PLACEMENT_3D('',#51047,#32008,#32009);
#28039=AXIS2_PLACEMENT_3D('',#51048,#32010,#32011);
#28040=AXIS2_PLACEMENT_3D('',#51050,#32012,#32013);
#28041=AXIS2_PLACEMENT_3D('',#51053,#32015,#32016);
#28042=AXIS2_PLACEMENT_3D('',#51054,#32017,#32018);
#28043=AXIS2_PLACEMENT_3D('',#51056,#32019,#32020);
#28044=AXIS2_PLACEMENT_3D('',#51059,#32022,#32023);
#28045=AXIS2_PLACEMENT_3D('',#51060,#32024,#32025);
#28046=AXIS2_PLACEMENT_3D('',#51062,#32026,#32027);
#28047=AXIS2_PLACEMENT_3D('',#51065,#32029,#32030);
#28048=AXIS2_PLACEMENT_3D('',#51066,#32031,#32032);
#28049=AXIS2_PLACEMENT_3D('',#51068,#32033,#32034);
#28050=AXIS2_PLACEMENT_3D('',#51071,#32036,#32037);
#28051=AXIS2_PLACEMENT_3D('',#51072,#32038,#32039);
#28052=AXIS2_PLACEMENT_3D('',#51074,#32040,#32041);
#28053=AXIS2_PLACEMENT_3D('',#51077,#32043,#32044);
#28054=AXIS2_PLACEMENT_3D('',#51078,#32045,#32046);
#28055=AXIS2_PLACEMENT_3D('',#51084,#32050,#32051);
#28056=AXIS2_PLACEMENT_3D('',#51090,#32055,#32056);
#28057=AXIS2_PLACEMENT_3D('',#51096,#32060,#32061);
#28058=AXIS2_PLACEMENT_3D('',#51102,#32065,#32066);
#28059=AXIS2_PLACEMENT_3D('',#51108,#32070,#32071);
#28060=AXIS2_PLACEMENT_3D('',#51114,#32075,#32076);
#28061=AXIS2_PLACEMENT_3D('',#51120,#32080,#32081);
#28062=AXIS2_PLACEMENT_3D('',#51126,#32085,#32086);
#28063=AXIS2_PLACEMENT_3D('',#51132,#32090,#32091);
#28064=AXIS2_PLACEMENT_3D('',#51138,#32095,#32096);
#28065=AXIS2_PLACEMENT_3D('',#51144,#32100,#32101);
#28066=AXIS2_PLACEMENT_3D('',#51150,#32105,#32106);
#28067=AXIS2_PLACEMENT_3D('',#51156,#32110,#32111);
#28068=AXIS2_PLACEMENT_3D('',#51162,#32115,#32116);
#28069=AXIS2_PLACEMENT_3D('',#51168,#32120,#32121);
#28070=AXIS2_PLACEMENT_3D('',#51174,#32125,#32126);
#28071=AXIS2_PLACEMENT_3D('',#51180,#32130,#32131);
#28072=AXIS2_PLACEMENT_3D('',#51186,#32135,#32136);
#28073=AXIS2_PLACEMENT_3D('',#51192,#32140,#32141);
#28074=AXIS2_PLACEMENT_3D('',#51198,#32145,#32146);
#28075=AXIS2_PLACEMENT_3D('',#51204,#32150,#32151);
#28076=AXIS2_PLACEMENT_3D('',#51210,#32155,#32156);
#28077=AXIS2_PLACEMENT_3D('',#51216,#32160,#32161);
#28078=AXIS2_PLACEMENT_3D('',#51222,#32165,#32166);
#28079=AXIS2_PLACEMENT_3D('',#51228,#32170,#32171);
#28080=AXIS2_PLACEMENT_3D('',#51234,#32175,#32176);
#28081=AXIS2_PLACEMENT_3D('',#51240,#32180,#32181);
#28082=AXIS2_PLACEMENT_3D('',#51246,#32185,#32186);
#28083=AXIS2_PLACEMENT_3D('',#51252,#32190,#32191);
#28084=AXIS2_PLACEMENT_3D('',#51258,#32195,#32196);
#28085=AXIS2_PLACEMENT_3D('',#51264,#32200,#32201);
#28086=AXIS2_PLACEMENT_3D('',#51270,#32205,#32206);
#28087=AXIS2_PLACEMENT_3D('',#51276,#32210,#32211);
#28088=AXIS2_PLACEMENT_3D('',#51282,#32215,#32216);
#28089=AXIS2_PLACEMENT_3D('',#51288,#32220,#32221);
#28090=AXIS2_PLACEMENT_3D('',#51294,#32225,#32226);
#28091=AXIS2_PLACEMENT_3D('',#51300,#32230,#32231);
#28092=AXIS2_PLACEMENT_3D('',#51306,#32235,#32236);
#28093=AXIS2_PLACEMENT_3D('',#51312,#32240,#32241);
#28094=AXIS2_PLACEMENT_3D('',#51318,#32245,#32246);
#28095=AXIS2_PLACEMENT_3D('',#51324,#32250,#32251);
#28096=AXIS2_PLACEMENT_3D('',#51330,#32255,#32256);
#28097=AXIS2_PLACEMENT_3D('',#51336,#32260,#32261);
#28098=AXIS2_PLACEMENT_3D('',#51342,#32265,#32266);
#28099=AXIS2_PLACEMENT_3D('',#51348,#32270,#32271);
#28100=AXIS2_PLACEMENT_3D('',#51354,#32275,#32276);
#28101=AXIS2_PLACEMENT_3D('',#51360,#32280,#32281);
#28102=AXIS2_PLACEMENT_3D('',#51366,#32285,#32286);
#28103=AXIS2_PLACEMENT_3D('',#51372,#32290,#32291);
#28104=AXIS2_PLACEMENT_3D('',#51378,#32295,#32296);
#28105=AXIS2_PLACEMENT_3D('',#51384,#32300,#32301);
#28106=AXIS2_PLACEMENT_3D('',#51390,#32305,#32306);
#28107=AXIS2_PLACEMENT_3D('',#51396,#32310,#32311);
#28108=AXIS2_PLACEMENT_3D('',#51402,#32315,#32316);
#28109=AXIS2_PLACEMENT_3D('',#51408,#32320,#32321);
#28110=AXIS2_PLACEMENT_3D('',#51414,#32325,#32326);
#28111=AXIS2_PLACEMENT_3D('',#51420,#32330,#32331);
#28112=AXIS2_PLACEMENT_3D('',#51426,#32335,#32336);
#28113=AXIS2_PLACEMENT_3D('',#51432,#32340,#32341);
#28114=AXIS2_PLACEMENT_3D('',#51438,#32345,#32346);
#28115=AXIS2_PLACEMENT_3D('',#51444,#32350,#32351);
#28116=AXIS2_PLACEMENT_3D('',#51450,#32355,#32356);
#28117=AXIS2_PLACEMENT_3D('',#51456,#32360,#32361);
#28118=AXIS2_PLACEMENT_3D('',#51462,#32365,#32366);
#28119=AXIS2_PLACEMENT_3D('',#51468,#32370,#32371);
#28120=AXIS2_PLACEMENT_3D('',#51474,#32375,#32376);
#28121=AXIS2_PLACEMENT_3D('',#51480,#32380,#32381);
#28122=AXIS2_PLACEMENT_3D('',#51486,#32385,#32386);
#28123=AXIS2_PLACEMENT_3D('',#51492,#32390,#32391);
#28124=AXIS2_PLACEMENT_3D('',#51498,#32395,#32396);
#28125=AXIS2_PLACEMENT_3D('',#51504,#32400,#32401);
#28126=AXIS2_PLACEMENT_3D('',#51510,#32405,#32406);
#28127=AXIS2_PLACEMENT_3D('',#51516,#32410,#32411);
#28128=AXIS2_PLACEMENT_3D('',#51522,#32415,#32416);
#28129=AXIS2_PLACEMENT_3D('',#51528,#32420,#32421);
#28130=AXIS2_PLACEMENT_3D('',#51534,#32425,#32426);
#28131=AXIS2_PLACEMENT_3D('',#51540,#32430,#32431);
#28132=AXIS2_PLACEMENT_3D('',#51546,#32435,#32436);
#28133=AXIS2_PLACEMENT_3D('',#51552,#32440,#32441);
#28134=AXIS2_PLACEMENT_3D('',#51558,#32445,#32446);
#28135=AXIS2_PLACEMENT_3D('',#51564,#32450,#32451);
#28136=AXIS2_PLACEMENT_3D('',#51570,#32455,#32456);
#28137=AXIS2_PLACEMENT_3D('',#51576,#32460,#32461);
#28138=AXIS2_PLACEMENT_3D('',#51582,#32465,#32466);
#28139=AXIS2_PLACEMENT_3D('',#51588,#32470,#32471);
#28140=AXIS2_PLACEMENT_3D('',#51594,#32475,#32476);
#28141=AXIS2_PLACEMENT_3D('',#51600,#32480,#32481);
#28142=AXIS2_PLACEMENT_3D('',#51606,#32485,#32486);
#28143=AXIS2_PLACEMENT_3D('',#51612,#32490,#32491);
#28144=AXIS2_PLACEMENT_3D('',#51618,#32495,#32496);
#28145=AXIS2_PLACEMENT_3D('',#51624,#32500,#32501);
#28146=AXIS2_PLACEMENT_3D('',#51630,#32505,#32506);
#28147=AXIS2_PLACEMENT_3D('',#51636,#32510,#32511);
#28148=AXIS2_PLACEMENT_3D('',#51642,#32515,#32516);
#28149=AXIS2_PLACEMENT_3D('',#51648,#32520,#32521);
#28150=AXIS2_PLACEMENT_3D('',#51654,#32525,#32526);
#28151=AXIS2_PLACEMENT_3D('',#51660,#32530,#32531);
#28152=AXIS2_PLACEMENT_3D('',#51666,#32535,#32536);
#28153=AXIS2_PLACEMENT_3D('',#51672,#32540,#32541);
#28154=AXIS2_PLACEMENT_3D('',#51678,#32545,#32546);
#28155=AXIS2_PLACEMENT_3D('',#51684,#32550,#32551);
#28156=AXIS2_PLACEMENT_3D('',#51690,#32555,#32556);
#28157=AXIS2_PLACEMENT_3D('',#51696,#32560,#32561);
#28158=AXIS2_PLACEMENT_3D('',#51702,#32565,#32566);
#28159=AXIS2_PLACEMENT_3D('',#51708,#32570,#32571);
#28160=AXIS2_PLACEMENT_3D('',#51714,#32575,#32576);
#28161=AXIS2_PLACEMENT_3D('',#51720,#32580,#32581);
#28162=AXIS2_PLACEMENT_3D('',#51726,#32585,#32586);
#28163=AXIS2_PLACEMENT_3D('',#51732,#32590,#32591);
#28164=AXIS2_PLACEMENT_3D('',#51738,#32595,#32596);
#28165=AXIS2_PLACEMENT_3D('',#51744,#32600,#32601);
#28166=AXIS2_PLACEMENT_3D('',#51750,#32605,#32606);
#28167=AXIS2_PLACEMENT_3D('',#51756,#32610,#32611);
#28168=AXIS2_PLACEMENT_3D('',#51762,#32615,#32616);
#28169=AXIS2_PLACEMENT_3D('',#51768,#32620,#32621);
#28170=AXIS2_PLACEMENT_3D('',#51774,#32625,#32626);
#28171=AXIS2_PLACEMENT_3D('',#51780,#32630,#32631);
#28172=AXIS2_PLACEMENT_3D('',#51786,#32635,#32636);
#28173=AXIS2_PLACEMENT_3D('',#51792,#32640,#32641);
#28174=AXIS2_PLACEMENT_3D('',#51798,#32645,#32646);
#28175=AXIS2_PLACEMENT_3D('',#51804,#32650,#32651);
#28176=AXIS2_PLACEMENT_3D('',#51810,#32655,#32656);
#28177=AXIS2_PLACEMENT_3D('',#51816,#32660,#32661);
#28178=AXIS2_PLACEMENT_3D('',#51822,#32665,#32666);
#28179=AXIS2_PLACEMENT_3D('',#51828,#32670,#32671);
#28180=AXIS2_PLACEMENT_3D('',#51834,#32675,#32676);
#28181=AXIS2_PLACEMENT_3D('',#51840,#32680,#32681);
#28182=AXIS2_PLACEMENT_3D('',#51846,#32685,#32686);
#28183=AXIS2_PLACEMENT_3D('',#51852,#32690,#32691);
#28184=AXIS2_PLACEMENT_3D('',#51858,#32695,#32696);
#28185=AXIS2_PLACEMENT_3D('',#51864,#32700,#32701);
#28186=AXIS2_PLACEMENT_3D('',#51870,#32705,#32706);
#28187=AXIS2_PLACEMENT_3D('',#51876,#32710,#32711);
#28188=AXIS2_PLACEMENT_3D('',#51882,#32715,#32716);
#28189=AXIS2_PLACEMENT_3D('',#51888,#32720,#32721);
#28190=AXIS2_PLACEMENT_3D('',#51894,#32725,#32726);
#28191=AXIS2_PLACEMENT_3D('',#51900,#32730,#32731);
#28192=AXIS2_PLACEMENT_3D('',#51906,#32735,#32736);
#28193=AXIS2_PLACEMENT_3D('',#51912,#32740,#32741);
#28194=AXIS2_PLACEMENT_3D('',#51918,#32745,#32746);
#28195=AXIS2_PLACEMENT_3D('',#51924,#32750,#32751);
#28196=AXIS2_PLACEMENT_3D('',#51930,#32755,#32756);
#28197=AXIS2_PLACEMENT_3D('',#51936,#32760,#32761);
#28198=AXIS2_PLACEMENT_3D('',#51942,#32765,#32766);
#28199=AXIS2_PLACEMENT_3D('',#51948,#32770,#32771);
#28200=AXIS2_PLACEMENT_3D('',#51954,#32775,#32776);
#28201=AXIS2_PLACEMENT_3D('',#51960,#32780,#32781);
#28202=AXIS2_PLACEMENT_3D('',#51966,#32785,#32786);
#28203=AXIS2_PLACEMENT_3D('',#51972,#32790,#32791);
#28204=AXIS2_PLACEMENT_3D('',#51978,#32795,#32796);
#28205=AXIS2_PLACEMENT_3D('',#51984,#32800,#32801);
#28206=AXIS2_PLACEMENT_3D('',#51990,#32805,#32806);
#28207=AXIS2_PLACEMENT_3D('',#51996,#32810,#32811);
#28208=AXIS2_PLACEMENT_3D('',#52002,#32815,#32816);
#28209=AXIS2_PLACEMENT_3D('',#52008,#32820,#32821);
#28210=AXIS2_PLACEMENT_3D('',#52014,#32825,#32826);
#28211=AXIS2_PLACEMENT_3D('',#52020,#32830,#32831);
#28212=AXIS2_PLACEMENT_3D('',#52026,#32835,#32836);
#28213=AXIS2_PLACEMENT_3D('',#52032,#32840,#32841);
#28214=AXIS2_PLACEMENT_3D('',#52038,#32845,#32846);
#28215=AXIS2_PLACEMENT_3D('',#52044,#32850,#32851);
#28216=AXIS2_PLACEMENT_3D('',#52050,#32855,#32856);
#28217=AXIS2_PLACEMENT_3D('',#52056,#32860,#32861);
#28218=AXIS2_PLACEMENT_3D('',#52062,#32865,#32866);
#28219=AXIS2_PLACEMENT_3D('',#52068,#32870,#32871);
#28220=AXIS2_PLACEMENT_3D('',#52074,#32875,#32876);
#28221=AXIS2_PLACEMENT_3D('',#52080,#32880,#32881);
#28222=AXIS2_PLACEMENT_3D('',#52086,#32885,#32886);
#28223=AXIS2_PLACEMENT_3D('',#52092,#32890,#32891);
#28224=AXIS2_PLACEMENT_3D('',#52098,#32895,#32896);
#28225=AXIS2_PLACEMENT_3D('',#52104,#32900,#32901);
#28226=AXIS2_PLACEMENT_3D('',#52110,#32905,#32906);
#28227=AXIS2_PLACEMENT_3D('',#52116,#32910,#32911);
#28228=AXIS2_PLACEMENT_3D('',#52122,#32915,#32916);
#28229=AXIS2_PLACEMENT_3D('',#52128,#32920,#32921);
#28230=AXIS2_PLACEMENT_3D('',#52134,#32925,#32926);
#28231=AXIS2_PLACEMENT_3D('',#52140,#32930,#32931);
#28232=AXIS2_PLACEMENT_3D('',#52146,#32935,#32936);
#28233=AXIS2_PLACEMENT_3D('',#52152,#32940,#32941);
#28234=AXIS2_PLACEMENT_3D('',#52158,#32945,#32946);
#28235=AXIS2_PLACEMENT_3D('',#52164,#32950,#32951);
#28236=AXIS2_PLACEMENT_3D('',#52170,#32955,#32956);
#28237=AXIS2_PLACEMENT_3D('',#52176,#32960,#32961);
#28238=AXIS2_PLACEMENT_3D('',#52182,#32965,#32966);
#28239=AXIS2_PLACEMENT_3D('',#52188,#32970,#32971);
#28240=AXIS2_PLACEMENT_3D('',#52194,#32975,#32976);
#28241=AXIS2_PLACEMENT_3D('',#52200,#32980,#32981);
#28242=AXIS2_PLACEMENT_3D('',#52206,#32985,#32986);
#28243=AXIS2_PLACEMENT_3D('',#52212,#32990,#32991);
#28244=AXIS2_PLACEMENT_3D('',#52218,#32995,#32996);
#28245=AXIS2_PLACEMENT_3D('',#52224,#33000,#33001);
#28246=AXIS2_PLACEMENT_3D('',#52230,#33005,#33006);
#28247=AXIS2_PLACEMENT_3D('',#52236,#33010,#33011);
#28248=AXIS2_PLACEMENT_3D('',#52242,#33015,#33016);
#28249=AXIS2_PLACEMENT_3D('',#52248,#33020,#33021);
#28250=AXIS2_PLACEMENT_3D('',#52254,#33025,#33026);
#28251=AXIS2_PLACEMENT_3D('',#52260,#33030,#33031);
#28252=AXIS2_PLACEMENT_3D('',#52266,#33035,#33036);
#28253=AXIS2_PLACEMENT_3D('',#52272,#33040,#33041);
#28254=AXIS2_PLACEMENT_3D('',#52278,#33045,#33046);
#28255=AXIS2_PLACEMENT_3D('',#52284,#33050,#33051);
#28256=AXIS2_PLACEMENT_3D('',#52290,#33055,#33056);
#28257=AXIS2_PLACEMENT_3D('',#52296,#33060,#33061);
#28258=AXIS2_PLACEMENT_3D('',#52302,#33065,#33066);
#28259=AXIS2_PLACEMENT_3D('',#52308,#33070,#33071);
#28260=AXIS2_PLACEMENT_3D('',#52314,#33075,#33076);
#28261=AXIS2_PLACEMENT_3D('',#52320,#33080,#33081);
#28262=AXIS2_PLACEMENT_3D('',#52326,#33085,#33086);
#28263=AXIS2_PLACEMENT_3D('',#52332,#33090,#33091);
#28264=AXIS2_PLACEMENT_3D('',#52338,#33095,#33096);
#28265=AXIS2_PLACEMENT_3D('',#52344,#33100,#33101);
#28266=AXIS2_PLACEMENT_3D('',#52350,#33105,#33106);
#28267=AXIS2_PLACEMENT_3D('',#52356,#33110,#33111);
#28268=AXIS2_PLACEMENT_3D('',#52362,#33115,#33116);
#28269=AXIS2_PLACEMENT_3D('',#52368,#33120,#33121);
#28270=AXIS2_PLACEMENT_3D('',#52374,#33125,#33126);
#28271=AXIS2_PLACEMENT_3D('',#52380,#33130,#33131);
#28272=AXIS2_PLACEMENT_3D('',#52386,#33135,#33136);
#28273=AXIS2_PLACEMENT_3D('',#52392,#33140,#33141);
#28274=AXIS2_PLACEMENT_3D('',#52398,#33145,#33146);
#28275=AXIS2_PLACEMENT_3D('',#52404,#33150,#33151);
#28276=AXIS2_PLACEMENT_3D('',#52410,#33155,#33156);
#28277=AXIS2_PLACEMENT_3D('',#52416,#33160,#33161);
#28278=AXIS2_PLACEMENT_3D('',#52422,#33165,#33166);
#28279=AXIS2_PLACEMENT_3D('',#52428,#33170,#33171);
#28280=AXIS2_PLACEMENT_3D('',#52434,#33175,#33176);
#28281=AXIS2_PLACEMENT_3D('',#52440,#33180,#33181);
#28282=AXIS2_PLACEMENT_3D('',#52446,#33185,#33186);
#28283=AXIS2_PLACEMENT_3D('',#52452,#33190,#33191);
#28284=AXIS2_PLACEMENT_3D('',#52458,#33195,#33196);
#28285=AXIS2_PLACEMENT_3D('',#52464,#33200,#33201);
#28286=AXIS2_PLACEMENT_3D('',#52470,#33205,#33206);
#28287=AXIS2_PLACEMENT_3D('',#52476,#33210,#33211);
#28288=AXIS2_PLACEMENT_3D('',#52482,#33215,#33216);
#28289=AXIS2_PLACEMENT_3D('',#52488,#33220,#33221);
#28290=AXIS2_PLACEMENT_3D('',#52494,#33225,#33226);
#28291=AXIS2_PLACEMENT_3D('',#52500,#33230,#33231);
#28292=AXIS2_PLACEMENT_3D('',#52506,#33235,#33236);
#28293=AXIS2_PLACEMENT_3D('',#52512,#33240,#33241);
#28294=AXIS2_PLACEMENT_3D('',#52518,#33245,#33246);
#28295=AXIS2_PLACEMENT_3D('',#52524,#33250,#33251);
#28296=AXIS2_PLACEMENT_3D('',#52530,#33255,#33256);
#28297=AXIS2_PLACEMENT_3D('',#52536,#33260,#33261);
#28298=AXIS2_PLACEMENT_3D('',#52542,#33265,#33266);
#28299=AXIS2_PLACEMENT_3D('',#52548,#33270,#33271);
#28300=AXIS2_PLACEMENT_3D('',#52554,#33275,#33276);
#28301=AXIS2_PLACEMENT_3D('',#52560,#33280,#33281);
#28302=AXIS2_PLACEMENT_3D('',#52566,#33285,#33286);
#28303=AXIS2_PLACEMENT_3D('',#52572,#33290,#33291);
#28304=AXIS2_PLACEMENT_3D('',#52578,#33295,#33296);
#28305=AXIS2_PLACEMENT_3D('',#52584,#33300,#33301);
#28306=AXIS2_PLACEMENT_3D('',#52590,#33305,#33306);
#28307=AXIS2_PLACEMENT_3D('',#52596,#33310,#33311);
#28308=AXIS2_PLACEMENT_3D('',#52602,#33315,#33316);
#28309=AXIS2_PLACEMENT_3D('',#52608,#33320,#33321);
#28310=AXIS2_PLACEMENT_3D('',#52614,#33325,#33326);
#28311=AXIS2_PLACEMENT_3D('',#52620,#33330,#33331);
#28312=AXIS2_PLACEMENT_3D('',#52626,#33335,#33336);
#28313=AXIS2_PLACEMENT_3D('',#52632,#33340,#33341);
#28314=AXIS2_PLACEMENT_3D('',#52638,#33345,#33346);
#28315=AXIS2_PLACEMENT_3D('',#52644,#33350,#33351);
#28316=AXIS2_PLACEMENT_3D('',#52650,#33355,#33356);
#28317=AXIS2_PLACEMENT_3D('',#52656,#33360,#33361);
#28318=AXIS2_PLACEMENT_3D('',#52662,#33365,#33366);
#28319=AXIS2_PLACEMENT_3D('',#52668,#33370,#33371);
#28320=AXIS2_PLACEMENT_3D('',#52674,#33375,#33376);
#28321=AXIS2_PLACEMENT_3D('',#52680,#33380,#33381);
#28322=AXIS2_PLACEMENT_3D('',#52686,#33385,#33386);
#28323=AXIS2_PLACEMENT_3D('',#52692,#33390,#33391);
#28324=AXIS2_PLACEMENT_3D('',#52698,#33395,#33396);
#28325=AXIS2_PLACEMENT_3D('',#52704,#33400,#33401);
#28326=AXIS2_PLACEMENT_3D('',#52710,#33405,#33406);
#28327=AXIS2_PLACEMENT_3D('',#52716,#33410,#33411);
#28328=AXIS2_PLACEMENT_3D('',#52722,#33415,#33416);
#28329=AXIS2_PLACEMENT_3D('',#52728,#33420,#33421);
#28330=AXIS2_PLACEMENT_3D('',#52734,#33425,#33426);
#28331=AXIS2_PLACEMENT_3D('',#52740,#33430,#33431);
#28332=AXIS2_PLACEMENT_3D('',#52746,#33435,#33436);
#28333=AXIS2_PLACEMENT_3D('',#52749,#33439,#33440);
#28334=AXIS2_PLACEMENT_3D('',#52750,#33441,#33442);
#31897=DIRECTION('axis',(0.,0.,1.));
#31898=DIRECTION('refdir',(1.,0.,0.));
#31899=DIRECTION('center_axis',(0.,0.70710678118654,-0.707106781186555));
#31900=DIRECTION('ref_axis',(-1.,0.,0.));
#31901=DIRECTION('',(-0.24924356936395,0.684791078771744,0.684791078771729));
#31902=DIRECTION('',(-1.,0.,0.));
#31903=DIRECTION('',(0.,0.707106781186557,0.707106781186538));
#31904=DIRECTION('',(1.,0.,0.));
#31905=DIRECTION('center_axis',(0.,-1.,0.));
#31906=DIRECTION('ref_axis',(0.,0.,-1.));
#31907=DIRECTION('',(0.,0.707106781186547,-0.707106781186547));
#31908=DIRECTION('center_axis',(0.,-1.,0.));
#31909=DIRECTION('ref_axis',(0.,0.,-1.));
#31910=DIRECTION('center_axis',(0.,1.,0.));
#31911=DIRECTION('ref_axis',(0.,0.,-1.));
#31912=DIRECTION('center_axis',(0.,0.70710678118654,0.707106781186555));
#31913=DIRECTION('ref_axis',(1.,0.,0.));
#31914=DIRECTION('',(6.28036983473502E-14,0.707106781186555,-0.70710678118654));
#31915=DIRECTION('',(-1.,0.,0.));
#31916=DIRECTION('',(1.,0.,0.));
#31917=DIRECTION('center_axis',(0.,-1.,0.));
#31918=DIRECTION('ref_axis',(0.,0.,1.));
#31919=DIRECTION('',(0.,0.707106781186547,0.707106781186547));
#31920=DIRECTION('center_axis',(0.,-1.,0.));
#31921=DIRECTION('ref_axis',(0.,0.,1.));
#31922=DIRECTION('center_axis',(0.,1.,0.));
#31923=DIRECTION('ref_axis',(0.,0.,1.));
#31924=DIRECTION('center_axis',(0.,0.70710678118654,-0.707106781186555));
#31925=DIRECTION('ref_axis',(-1.,0.,0.));
#31926=DIRECTION('',(-0.24924356936395,-0.684791078771744,-0.684791078771729));
#31927=DIRECTION('',(1.,0.,0.));
#31928=DIRECTION('',(-1.,0.,0.));
#31929=DIRECTION('center_axis',(0.,0.,-1.));
#31930=DIRECTION('ref_axis',(-1.,0.,0.));
#31931=DIRECTION('',(0.,1.,0.));
#31932=DIRECTION('',(1.,0.,0.));
#31933=DIRECTION('',(0.,1.,0.));
#31934=DIRECTION('center_axis',(0.,1.,0.));
#31935=DIRECTION('ref_axis',(0.,0.,1.));
#31936=DIRECTION('',(0.,1.,0.));
#31937=DIRECTION('center_axis',(0.,-1.,0.));
#31938=DIRECTION('ref_axis',(0.,0.,1.));
#31939=DIRECTION('center_axis',(0.,0.,1.));
#31940=DIRECTION('ref_axis',(1.,0.,0.));
#31941=DIRECTION('',(0.,1.,0.));
#31942=DIRECTION('',(-1.,0.,0.));
#31943=DIRECTION('center_axis',(0.,1.,0.));
#31944=DIRECTION('ref_axis',(0.,0.,-1.));
#31945=DIRECTION('',(0.,1.,0.));
#31946=DIRECTION('center_axis',(0.,-1.,0.));
#31947=DIRECTION('ref_axis',(0.,0.,-1.));
#31948=DIRECTION('center_axis',(0.,0.,-1.));
#31949=DIRECTION('ref_axis',(-1.,0.,0.));
#31950=DIRECTION('',(0.,1.,0.));
#31951=DIRECTION('',(1.,0.,0.));
#31952=DIRECTION('center_axis',(0.,-0.707106781186555,-0.70710678118654));
#31953=DIRECTION('ref_axis',(-1.,0.,0.));
#31954=DIRECTION('',(0.249243569363955,-0.684791078771728,0.684791078771743));
#31955=DIRECTION('',(0.,-0.707106781186544,0.707106781186551));
#31956=DIRECTION('',(-1.,0.,0.));
#31957=DIRECTION('center_axis',(0.,1.,0.));
#31958=DIRECTION('ref_axis',(0.,0.,1.));
#31959=DIRECTION('',(0.,-0.707106781186548,-0.707106781186548));
#31960=DIRECTION('center_axis',(0.,1.,0.));
#31961=DIRECTION('ref_axis',(0.,0.,1.));
#31962=DIRECTION('center_axis',(0.,-0.707106781186555,0.70710678118654));
#31963=DIRECTION('ref_axis',(1.,0.,0.));
#31964=DIRECTION('',(0.,-0.70710678118654,-0.707106781186555));
#31965=DIRECTION('',(1.,0.,0.));
#31966=DIRECTION('center_axis',(0.,1.,0.));
#31967=DIRECTION('ref_axis',(0.,0.,-1.));
#31968=DIRECTION('',(0.,-0.707106781186548,0.707106781186548));
#31969=DIRECTION('center_axis',(0.,1.,0.));
#31970=DIRECTION('ref_axis',(0.,0.,-1.));
#31971=DIRECTION('center_axis',(0.,-0.707106781186555,-0.70710678118654));
#31972=DIRECTION('ref_axis',(-1.,0.,0.));
#31973=DIRECTION('',(0.249243569363955,0.684791078771728,-0.684791078771743));
#31974=DIRECTION('',(-1.,0.,0.));
#31975=DIRECTION('center_axis',(0.,-1.,0.));
#31976=DIRECTION('ref_axis',(1.,0.,0.));
#31977=DIRECTION('center_axis',(0.,-1.,0.));
#31978=DIRECTION('ref_axis',(1.,0.,0.));
#31979=DIRECTION('',(0.,-1.,0.));
#31980=DIRECTION('center_axis',(0.,1.,0.));
#31981=DIRECTION('ref_axis',(1.,0.,0.));
#31982=DIRECTION('center_axis',(0.,-1.,0.));
#31983=DIRECTION('ref_axis',(1.,0.,0.));
#31984=DIRECTION('center_axis',(0.,-1.,0.));
#31985=DIRECTION('ref_axis',(1.,0.,0.));
#31986=DIRECTION('',(0.,-1.,0.));
#31987=DIRECTION('center_axis',(0.,1.,0.));
#31988=DIRECTION('ref_axis',(1.,0.,0.));
#31989=DIRECTION('center_axis',(0.,-1.,0.));
#31990=DIRECTION('ref_axis',(1.,0.,0.));
#31991=DIRECTION('center_axis',(0.,-1.,0.));
#31992=DIRECTION('ref_axis',(1.,0.,0.));
#31993=DIRECTION('',(0.,-1.,0.));
#31994=DIRECTION('center_axis',(0.,1.,0.));
#31995=DIRECTION('ref_axis',(1.,0.,0.));
#31996=DIRECTION('center_axis',(0.,-1.,0.));
#31997=DIRECTION('ref_axis',(1.,0.,0.));
#31998=DIRECTION('center_axis',(0.,-1.,0.));
#31999=DIRECTION('ref_axis',(1.,0.,0.));
#32000=DIRECTION('',(0.,-1.,0.));
#32001=DIRECTION('center_axis',(0.,1.,0.));
#32002=DIRECTION('ref_axis',(1.,0.,0.));
#32003=DIRECTION('center_axis',(0.,-1.,0.));
#32004=DIRECTION('ref_axis',(1.,0.,0.));
#32005=DIRECTION('center_axis',(0.,-1.,0.));
#32006=DIRECTION('ref_axis',(1.,0.,0.));
#32007=DIRECTION('',(0.,-1.,0.));
#32008=DIRECTION('center_axis',(0.,1.,0.));
#32009=DIRECTION('ref_axis',(1.,0.,0.));
#32010=DIRECTION('center_axis',(0.,-1.,0.));
#32011=DIRECTION('ref_axis',(1.,0.,0.));
#32012=DIRECTION('center_axis',(0.,-1.,0.));
#32013=DIRECTION('ref_axis',(1.,0.,0.));
#32014=DIRECTION('',(0.,-1.,0.));
#32015=DIRECTION('center_axis',(0.,1.,0.));
#32016=DIRECTION('ref_axis',(1.,0.,0.));
#32017=DIRECTION('center_axis',(0.,-1.,0.));
#32018=DIRECTION('ref_axis',(1.,0.,0.));
#32019=DIRECTION('center_axis',(0.,-1.,0.));
#32020=DIRECTION('ref_axis',(1.,0.,0.));
#32021=DIRECTION('',(0.,-1.,0.));
#32022=DIRECTION('center_axis',(0.,1.,0.));
#32023=DIRECTION('ref_axis',(1.,0.,0.));
#32024=DIRECTION('center_axis',(0.,-1.,0.));
#32025=DIRECTION('ref_axis',(1.,0.,0.));
#32026=DIRECTION('center_axis',(0.,-1.,0.));
#32027=DIRECTION('ref_axis',(1.,0.,0.));
#32028=DIRECTION('',(0.,-1.,0.));
#32029=DIRECTION('center_axis',(0.,1.,0.));
#32030=DIRECTION('ref_axis',(1.,0.,0.));
#32031=DIRECTION('center_axis',(0.,-1.,0.));
#32032=DIRECTION('ref_axis',(1.,0.,0.));
#32033=DIRECTION('center_axis',(0.,-1.,0.));
#32034=DIRECTION('ref_axis',(1.,0.,0.));
#32035=DIRECTION('',(0.,-1.,0.));
#32036=DIRECTION('center_axis',(0.,1.,0.));
#32037=DIRECTION('ref_axis',(1.,0.,0.));
#32038=DIRECTION('center_axis',(0.,-1.,0.));
#32039=DIRECTION('ref_axis',(1.,0.,0.));
#32040=DIRECTION('center_axis',(0.,-1.,0.));
#32041=DIRECTION('ref_axis',(1.,0.,0.));
#32042=DIRECTION('',(0.,-1.,0.));
#32043=DIRECTION('center_axis',(0.,1.,0.));
#32044=DIRECTION('ref_axis',(1.,0.,0.));
#32045=DIRECTION('center_axis',(-0.939692620785909,0.,-0.342020143325667));
#32046=DIRECTION('ref_axis',(-0.342020143325667,0.,0.939692620785909));
#32047=DIRECTION('',(0.342020143325667,0.,-0.939692620785909));
#32048=DIRECTION('',(-0.342020143325667,0.,0.939692620785909));
#32049=DIRECTION('',(0.,1.,0.));
#32050=DIRECTION('center_axis',(0.,0.,-1.));
#32051=DIRECTION('ref_axis',(-1.,0.,0.));
#32052=DIRECTION('',(1.,0.,0.));
#32053=DIRECTION('',(-1.,0.,0.));
#32054=DIRECTION('',(0.,1.,0.));
#32055=DIRECTION('center_axis',(0.939692620785909,0.,-0.342020143325667));
#32056=DIRECTION('ref_axis',(-0.342020143325667,0.,-0.939692620785909));
#32057=DIRECTION('',(0.342020143325667,0.,0.939692620785909));
#32058=DIRECTION('',(-0.342020143325667,0.,-0.939692620785909));
#32059=DIRECTION('',(0.,1.,0.));
#32060=DIRECTION('center_axis',(0.,0.,-1.));
#32061=DIRECTION('ref_axis',(-1.,0.,0.));
#32062=DIRECTION('',(1.,0.,0.));
#32063=DIRECTION('',(-1.,0.,0.));
#32064=DIRECTION('',(0.,1.,0.));
#32065=DIRECTION('center_axis',(-0.939692620785909,0.,-0.342020143325667));
#32066=DIRECTION('ref_axis',(-0.342020143325667,0.,0.939692620785909));
#32067=DIRECTION('',(0.342020143325667,0.,-0.939692620785909));
#32068=DIRECTION('',(-0.342020143325667,0.,0.939692620785909));
#32069=DIRECTION('',(0.,1.,0.));
#32070=DIRECTION('center_axis',(0.,0.,-1.));
#32071=DIRECTION('ref_axis',(-1.,0.,0.));
#32072=DIRECTION('',(1.,0.,0.));
#32073=DIRECTION('',(-1.,0.,0.));
#32074=DIRECTION('',(0.,1.,0.));
#32075=DIRECTION('center_axis',(0.939692620785909,0.,-0.342020143325667));
#32076=DIRECTION('ref_axis',(-0.342020143325667,0.,-0.939692620785909));
#32077=DIRECTION('',(0.342020143325667,0.,0.939692620785909));
#32078=DIRECTION('',(-0.342020143325667,0.,-0.939692620785909));
#32079=DIRECTION('',(0.,1.,0.));
#32080=DIRECTION('center_axis',(0.,0.,-1.));
#32081=DIRECTION('ref_axis',(-1.,0.,0.));
#32082=DIRECTION('',(1.,0.,0.));
#32083=DIRECTION('',(-1.,0.,0.));
#32084=DIRECTION('',(0.,1.,0.));
#32085=DIRECTION('center_axis',(-0.939692620785909,0.,-0.342020143325667));
#32086=DIRECTION('ref_axis',(-0.342020143325667,0.,0.939692620785909));
#32087=DIRECTION('',(0.342020143325667,0.,-0.939692620785909));
#32088=DIRECTION('',(-0.342020143325667,0.,0.939692620785909));
#32089=DIRECTION('',(0.,1.,0.));
#32090=DIRECTION('center_axis',(0.,0.,-1.));
#32091=DIRECTION('ref_axis',(-1.,0.,0.));
#32092=DIRECTION('',(1.,0.,0.));
#32093=DIRECTION('',(-1.,0.,0.));
#32094=DIRECTION('',(0.,1.,0.));
#32095=DIRECTION('center_axis',(0.939692620785909,0.,-0.342020143325667));
#32096=DIRECTION('ref_axis',(-0.342020143325667,0.,-0.939692620785909));
#32097=DIRECTION('',(0.342020143325667,0.,0.939692620785909));
#32098=DIRECTION('',(-0.342020143325667,0.,-0.939692620785909));
#32099=DIRECTION('',(0.,1.,0.));
#32100=DIRECTION('center_axis',(0.,0.,-1.));
#32101=DIRECTION('ref_axis',(-1.,0.,0.));
#32102=DIRECTION('',(1.,0.,0.));
#32103=DIRECTION('',(-1.,0.,0.));
#32104=DIRECTION('',(0.,1.,0.));
#32105=DIRECTION('center_axis',(-0.939692620785909,0.,-0.342020143325667));
#32106=DIRECTION('ref_axis',(-0.342020143325667,0.,0.939692620785909));
#32107=DIRECTION('',(0.342020143325667,0.,-0.939692620785909));
#32108=DIRECTION('',(-0.342020143325667,0.,0.939692620785909));
#32109=DIRECTION('',(0.,1.,0.));
#32110=DIRECTION('center_axis',(0.,0.,-1.));
#32111=DIRECTION('ref_axis',(-1.,0.,0.));
#32112=DIRECTION('',(1.,0.,0.));
#32113=DIRECTION('',(-1.,0.,0.));
#32114=DIRECTION('',(0.,1.,0.));
#32115=DIRECTION('center_axis',(0.939692620785909,0.,-0.342020143325667));
#32116=DIRECTION('ref_axis',(-0.342020143325667,0.,-0.939692620785909));
#32117=DIRECTION('',(0.342020143325667,0.,0.939692620785909));
#32118=DIRECTION('',(-0.342020143325667,0.,-0.939692620785909));
#32119=DIRECTION('',(0.,1.,0.));
#32120=DIRECTION('center_axis',(0.,0.,-1.));
#32121=DIRECTION('ref_axis',(-1.,0.,0.));
#32122=DIRECTION('',(1.,0.,0.));
#32123=DIRECTION('',(-1.,0.,0.));
#32124=DIRECTION('',(0.,1.,0.));
#32125=DIRECTION('center_axis',(-0.939692620785909,0.,-0.342020143325667));
#32126=DIRECTION('ref_axis',(-0.342020143325667,0.,0.939692620785909));
#32127=DIRECTION('',(0.342020143325667,0.,-0.939692620785909));
#32128=DIRECTION('',(-0.342020143325667,0.,0.939692620785909));
#32129=DIRECTION('',(0.,1.,0.));
#32130=DIRECTION('center_axis',(0.,0.,-1.));
#32131=DIRECTION('ref_axis',(-1.,0.,0.));
#32132=DIRECTION('',(1.,0.,0.));
#32133=DIRECTION('',(-1.,0.,0.));
#32134=DIRECTION('',(0.,1.,0.));
#32135=DIRECTION('center_axis',(0.939692620785909,0.,-0.342020143325667));
#32136=DIRECTION('ref_axis',(-0.342020143325667,0.,-0.939692620785909));
#32137=DIRECTION('',(0.342020143325667,0.,0.939692620785909));
#32138=DIRECTION('',(-0.342020143325667,0.,-0.939692620785909));
#32139=DIRECTION('',(0.,1.,0.));
#32140=DIRECTION('center_axis',(0.,0.,-1.));
#32141=DIRECTION('ref_axis',(-1.,0.,0.));
#32142=DIRECTION('',(1.,0.,0.));
#32143=DIRECTION('',(-1.,0.,0.));
#32144=DIRECTION('',(0.,1.,0.));
#32145=DIRECTION('center_axis',(-0.939692620785911,0.,-0.342020143325663));
#32146=DIRECTION('ref_axis',(-0.342020143325663,0.,0.939692620785911));
#32147=DIRECTION('',(0.342020143325663,0.,-0.939692620785911));
#32148=DIRECTION('',(-0.342020143325663,0.,0.939692620785911));
#32149=DIRECTION('',(0.,1.,0.));
#32150=DIRECTION('center_axis',(0.,0.,-1.));
#32151=DIRECTION('ref_axis',(-1.,0.,0.));
#32152=DIRECTION('',(1.,0.,0.));
#32153=DIRECTION('',(-1.,0.,0.));
#32154=DIRECTION('',(0.,1.,0.));
#32155=DIRECTION('center_axis',(0.939692620785911,0.,-0.342020143325663));
#32156=DIRECTION('ref_axis',(-0.342020143325663,0.,-0.939692620785911));
#32157=DIRECTION('',(0.342020143325663,0.,0.939692620785911));
#32158=DIRECTION('',(-0.342020143325663,0.,-0.939692620785911));
#32159=DIRECTION('',(0.,1.,0.));
#32160=DIRECTION('center_axis',(0.,0.,-1.));
#32161=DIRECTION('ref_axis',(-1.,0.,0.));
#32162=DIRECTION('',(1.,0.,0.));
#32163=DIRECTION('',(-1.,0.,0.));
#32164=DIRECTION('',(0.,1.,0.));
#32165=DIRECTION('center_axis',(-0.939692620785911,0.,-0.342020143325663));
#32166=DIRECTION('ref_axis',(-0.342020143325663,0.,0.939692620785911));
#32167=DIRECTION('',(0.342020143325663,0.,-0.939692620785911));
#32168=DIRECTION('',(-0.342020143325663,0.,0.939692620785911));
#32169=DIRECTION('',(0.,1.,0.));
#32170=DIRECTION('center_axis',(0.,0.,-1.));
#32171=DIRECTION('ref_axis',(-1.,0.,0.));
#32172=DIRECTION('',(1.,0.,0.));
#32173=DIRECTION('',(-1.,0.,0.));
#32174=DIRECTION('',(0.,1.,0.));
#32175=DIRECTION('center_axis',(0.939692620785911,0.,-0.342020143325663));
#32176=DIRECTION('ref_axis',(-0.342020143325663,0.,-0.939692620785911));
#32177=DIRECTION('',(0.342020143325663,0.,0.939692620785911));
#32178=DIRECTION('',(-0.342020143325663,0.,-0.939692620785911));
#32179=DIRECTION('',(0.,1.,0.));
#32180=DIRECTION('center_axis',(0.,0.,-1.));
#32181=DIRECTION('ref_axis',(-1.,0.,0.));
#32182=DIRECTION('',(1.,0.,0.));
#32183=DIRECTION('',(-1.,0.,0.));
#32184=DIRECTION('',(0.,1.,0.));
#32185=DIRECTION('center_axis',(-0.939692620785909,0.,-0.342020143325667));
#32186=DIRECTION('ref_axis',(-0.342020143325667,0.,0.939692620785909));
#32187=DIRECTION('',(0.342020143325667,0.,-0.939692620785909));
#32188=DIRECTION('',(-0.342020143325667,0.,0.939692620785909));
#32189=DIRECTION('',(0.,1.,0.));
#32190=DIRECTION('center_axis',(0.,0.,-1.));
#32191=DIRECTION('ref_axis',(-1.,0.,0.));
#32192=DIRECTION('',(1.,0.,0.));
#32193=DIRECTION('',(-1.,0.,0.));
#32194=DIRECTION('',(0.,1.,0.));
#32195=DIRECTION('center_axis',(0.939692620785909,0.,-0.342020143325667));
#32196=DIRECTION('ref_axis',(-0.342020143325667,0.,-0.939692620785909));
#32197=DIRECTION('',(0.342020143325667,0.,0.939692620785909));
#32198=DIRECTION('',(-0.342020143325667,0.,-0.939692620785909));
#32199=DIRECTION('',(0.,1.,0.));
#32200=DIRECTION('center_axis',(0.,0.,-1.));
#32201=DIRECTION('ref_axis',(-1.,0.,0.));
#32202=DIRECTION('',(1.,0.,0.));
#32203=DIRECTION('',(-1.,0.,0.));
#32204=DIRECTION('',(0.,1.,0.));
#32205=DIRECTION('center_axis',(-0.939692620785909,0.,-0.342020143325667));
#32206=DIRECTION('ref_axis',(-0.342020143325667,0.,0.939692620785909));
#32207=DIRECTION('',(0.342020143325667,0.,-0.939692620785909));
#32208=DIRECTION('',(-0.342020143325667,0.,0.939692620785909));
#32209=DIRECTION('',(0.,1.,0.));
#32210=DIRECTION('center_axis',(0.,0.,-1.));
#32211=DIRECTION('ref_axis',(-1.,0.,0.));
#32212=DIRECTION('',(1.,0.,0.));
#32213=DIRECTION('',(-1.,0.,0.));
#32214=DIRECTION('',(0.,1.,0.));
#32215=DIRECTION('center_axis',(0.939692620785909,0.,-0.342020143325667));
#32216=DIRECTION('ref_axis',(-0.342020143325667,0.,-0.939692620785909));
#32217=DIRECTION('',(0.342020143325667,0.,0.939692620785909));
#32218=DIRECTION('',(-0.342020143325667,0.,-0.939692620785909));
#32219=DIRECTION('',(0.,1.,0.));
#32220=DIRECTION('center_axis',(0.,0.,-1.));
#32221=DIRECTION('ref_axis',(-1.,0.,0.));
#32222=DIRECTION('',(1.,0.,0.));
#32223=DIRECTION('',(-1.,0.,0.));
#32224=DIRECTION('',(0.,1.,0.));
#32225=DIRECTION('center_axis',(-0.939692620785908,0.,-0.342020143325671));
#32226=DIRECTION('ref_axis',(-0.342020143325671,0.,0.939692620785908));
#32227=DIRECTION('',(0.342020143325671,0.,-0.939692620785907));
#32228=DIRECTION('',(-0.342020143325671,0.,0.939692620785907));
#32229=DIRECTION('',(0.,1.,0.));
#32230=DIRECTION('center_axis',(0.,0.,-1.));
#32231=DIRECTION('ref_axis',(-1.,0.,0.));
#32232=DIRECTION('',(1.,0.,0.));
#32233=DIRECTION('',(-1.,0.,0.));
#32234=DIRECTION('',(0.,1.,0.));
#32235=DIRECTION('center_axis',(0.939692620785908,0.,-0.342020143325671));
#32236=DIRECTION('ref_axis',(-0.342020143325671,0.,-0.939692620785908));
#32237=DIRECTION('',(0.342020143325671,0.,0.939692620785907));
#32238=DIRECTION('',(-0.342020143325671,0.,-0.939692620785907));
#32239=DIRECTION('',(0.,1.,0.));
#32240=DIRECTION('center_axis',(0.,0.,-1.));
#32241=DIRECTION('ref_axis',(-1.,0.,0.));
#32242=DIRECTION('',(1.,0.,0.));
#32243=DIRECTION('',(-1.,0.,0.));
#32244=DIRECTION('',(0.,1.,0.));
#32245=DIRECTION('center_axis',(-0.939692620785908,0.,-0.342020143325671));
#32246=DIRECTION('ref_axis',(-0.342020143325671,0.,0.939692620785908));
#32247=DIRECTION('',(0.342020143325671,0.,-0.939692620785907));
#32248=DIRECTION('',(-0.342020143325671,0.,0.939692620785907));
#32249=DIRECTION('',(0.,1.,0.));
#32250=DIRECTION('center_axis',(0.,0.,-1.));
#32251=DIRECTION('ref_axis',(-1.,0.,0.));
#32252=DIRECTION('',(1.,0.,0.));
#32253=DIRECTION('',(-1.,0.,0.));
#32254=DIRECTION('',(0.,1.,0.));
#32255=DIRECTION('center_axis',(0.939692620785909,0.,-0.342020143325667));
#32256=DIRECTION('ref_axis',(-0.342020143325667,0.,-0.939692620785909));
#32257=DIRECTION('',(0.342020143325667,0.,0.939692620785909));
#32258=DIRECTION('',(-0.342020143325667,0.,-0.939692620785909));
#32259=DIRECTION('',(0.,1.,0.));
#32260=DIRECTION('center_axis',(0.,0.,-1.));
#32261=DIRECTION('ref_axis',(-1.,0.,0.));
#32262=DIRECTION('',(1.,0.,0.));
#32263=DIRECTION('',(-1.,0.,0.));
#32264=DIRECTION('',(0.,1.,0.));
#32265=DIRECTION('center_axis',(-0.939692620785909,0.,-0.342020143325667));
#32266=DIRECTION('ref_axis',(-0.342020143325667,0.,0.939692620785909));
#32267=DIRECTION('',(0.342020143325667,0.,-0.939692620785909));
#32268=DIRECTION('',(-0.342020143325667,0.,0.939692620785909));
#32269=DIRECTION('',(0.,1.,0.));
#32270=DIRECTION('center_axis',(0.,0.,-1.));
#32271=DIRECTION('ref_axis',(-1.,0.,0.));
#32272=DIRECTION('',(1.,0.,0.));
#32273=DIRECTION('',(-1.,0.,0.));
#32274=DIRECTION('',(0.,1.,0.));
#32275=DIRECTION('center_axis',(0.939692620785909,0.,-0.342020143325667));
#32276=DIRECTION('ref_axis',(-0.342020143325667,0.,-0.939692620785909));
#32277=DIRECTION('',(0.342020143325667,0.,0.939692620785909));
#32278=DIRECTION('',(-0.342020143325667,0.,-0.939692620785909));
#32279=DIRECTION('',(0.,1.,0.));
#32280=DIRECTION('center_axis',(0.,0.,-1.));
#32281=DIRECTION('ref_axis',(-1.,0.,0.));
#32282=DIRECTION('',(1.,0.,0.));
#32283=DIRECTION('',(-1.,0.,0.));
#32284=DIRECTION('',(0.,1.,0.));
#32285=DIRECTION('center_axis',(-0.939692620785909,0.,-0.342020143325667));
#32286=DIRECTION('ref_axis',(-0.342020143325667,0.,0.939692620785909));
#32287=DIRECTION('',(0.342020143325667,0.,-0.939692620785909));
#32288=DIRECTION('',(-0.342020143325667,0.,0.939692620785909));
#32289=DIRECTION('',(0.,1.,0.));
#32290=DIRECTION('center_axis',(0.,0.,-1.));
#32291=DIRECTION('ref_axis',(-1.,0.,0.));
#32292=DIRECTION('',(1.,0.,0.));
#32293=DIRECTION('',(-1.,0.,0.));
#32294=DIRECTION('',(0.,1.,0.));
#32295=DIRECTION('center_axis',(0.939692620785909,0.,-0.342020143325667));
#32296=DIRECTION('ref_axis',(-0.342020143325667,0.,-0.939692620785909));
#32297=DIRECTION('',(0.342020143325667,0.,0.939692620785909));
#32298=DIRECTION('',(-0.342020143325667,0.,-0.939692620785909));
#32299=DIRECTION('',(0.,1.,0.));
#32300=DIRECTION('center_axis',(0.,0.,-1.));
#32301=DIRECTION('ref_axis',(-1.,0.,0.));
#32302=DIRECTION('',(1.,0.,0.));
#32303=DIRECTION('',(-1.,0.,0.));
#32304=DIRECTION('',(0.,1.,0.));
#32305=DIRECTION('center_axis',(-0.939692620785909,0.,-0.342020143325667));
#32306=DIRECTION('ref_axis',(-0.342020143325667,0.,0.939692620785909));
#32307=DIRECTION('',(0.342020143325667,0.,-0.939692620785909));
#32308=DIRECTION('',(-0.342020143325667,0.,0.939692620785909));
#32309=DIRECTION('',(0.,1.,0.));
#32310=DIRECTION('center_axis',(0.,0.,-1.));
#32311=DIRECTION('ref_axis',(-1.,0.,0.));
#32312=DIRECTION('',(1.,0.,0.));
#32313=DIRECTION('',(-1.,0.,0.));
#32314=DIRECTION('',(0.,1.,0.));
#32315=DIRECTION('center_axis',(0.939692620785908,0.,-0.342020143325671));
#32316=DIRECTION('ref_axis',(-0.342020143325671,0.,-0.939692620785908));
#32317=DIRECTION('',(0.342020143325671,0.,0.939692620785907));
#32318=DIRECTION('',(-0.342020143325671,0.,-0.939692620785907));
#32319=DIRECTION('',(0.,1.,0.));
#32320=DIRECTION('center_axis',(0.,0.,-1.));
#32321=DIRECTION('ref_axis',(-1.,0.,0.));
#32322=DIRECTION('',(1.,0.,0.));
#32323=DIRECTION('',(-1.,0.,0.));
#32324=DIRECTION('',(0.,1.,0.));
#32325=DIRECTION('center_axis',(-0.939692620785908,0.,-0.342020143325671));
#32326=DIRECTION('ref_axis',(-0.342020143325671,0.,0.939692620785908));
#32327=DIRECTION('',(0.342020143325671,0.,-0.939692620785907));
#32328=DIRECTION('',(-0.342020143325671,0.,0.939692620785907));
#32329=DIRECTION('',(0.,1.,0.));
#32330=DIRECTION('center_axis',(0.,0.,-1.));
#32331=DIRECTION('ref_axis',(-1.,0.,0.));
#32332=DIRECTION('',(1.,0.,0.));
#32333=DIRECTION('',(-1.,0.,0.));
#32334=DIRECTION('',(0.,1.,0.));
#32335=DIRECTION('center_axis',(0.939692620785908,0.,-0.342020143325671));
#32336=DIRECTION('ref_axis',(-0.342020143325671,0.,-0.939692620785908));
#32337=DIRECTION('',(0.342020143325671,0.,0.939692620785907));
#32338=DIRECTION('',(-0.342020143325671,0.,-0.939692620785907));
#32339=DIRECTION('',(0.,1.,0.));
#32340=DIRECTION('center_axis',(0.,0.,-1.));
#32341=DIRECTION('ref_axis',(-1.,0.,0.));
#32342=DIRECTION('',(1.,0.,0.));
#32343=DIRECTION('',(-1.,0.,0.));
#32344=DIRECTION('',(0.,1.,0.));
#32345=DIRECTION('center_axis',(-0.939692620785908,0.,-0.342020143325671));
#32346=DIRECTION('ref_axis',(-0.342020143325671,0.,0.939692620785908));
#32347=DIRECTION('',(0.342020143325671,0.,-0.939692620785907));
#32348=DIRECTION('',(-0.342020143325671,0.,0.939692620785907));
#32349=DIRECTION('',(0.,1.,0.));
#32350=DIRECTION('center_axis',(0.,0.,-1.));
#32351=DIRECTION('ref_axis',(-1.,0.,0.));
#32352=DIRECTION('',(1.,0.,0.));
#32353=DIRECTION('',(-1.,0.,0.));
#32354=DIRECTION('',(0.,1.,0.));
#32355=DIRECTION('center_axis',(0.939692620785908,0.,-0.342020143325671));
#32356=DIRECTION('ref_axis',(-0.342020143325671,0.,-0.939692620785908));
#32357=DIRECTION('',(0.342020143325671,0.,0.939692620785907));
#32358=DIRECTION('',(-0.342020143325671,0.,-0.939692620785907));
#32359=DIRECTION('',(0.,1.,0.));
#32360=DIRECTION('center_axis',(0.,0.,-1.));
#32361=DIRECTION('ref_axis',(-1.,0.,0.));
#32362=DIRECTION('',(1.,0.,0.));
#32363=DIRECTION('',(-1.,0.,0.));
#32364=DIRECTION('',(0.,1.,0.));
#32365=DIRECTION('center_axis',(-0.939692620785908,0.,-0.342020143325671));
#32366=DIRECTION('ref_axis',(-0.342020143325671,0.,0.939692620785908));
#32367=DIRECTION('',(0.342020143325671,0.,-0.939692620785907));
#32368=DIRECTION('',(-0.342020143325671,0.,0.939692620785907));
#32369=DIRECTION('',(0.,1.,0.));
#32370=DIRECTION('center_axis',(0.,0.,-1.));
#32371=DIRECTION('ref_axis',(-1.,0.,0.));
#32372=DIRECTION('',(1.,0.,0.));
#32373=DIRECTION('',(-1.,0.,0.));
#32374=DIRECTION('',(0.,1.,0.));
#32375=DIRECTION('center_axis',(0.939692620785909,0.,-0.342020143325667));
#32376=DIRECTION('ref_axis',(-0.342020143325667,0.,-0.939692620785909));
#32377=DIRECTION('',(0.342020143325667,0.,0.939692620785909));
#32378=DIRECTION('',(-0.342020143325667,0.,-0.939692620785909));
#32379=DIRECTION('',(0.,1.,0.));
#32380=DIRECTION('center_axis',(0.,0.,-1.));
#32381=DIRECTION('ref_axis',(-1.,0.,0.));
#32382=DIRECTION('',(1.,0.,0.));
#32383=DIRECTION('',(-1.,0.,0.));
#32384=DIRECTION('',(0.,1.,0.));
#32385=DIRECTION('center_axis',(-0.939692620785909,0.,-0.342020143325667));
#32386=DIRECTION('ref_axis',(-0.342020143325667,0.,0.939692620785909));
#32387=DIRECTION('',(0.342020143325667,0.,-0.939692620785909));
#32388=DIRECTION('',(-0.342020143325667,0.,0.939692620785909));
#32389=DIRECTION('',(0.,1.,0.));
#32390=DIRECTION('center_axis',(0.,0.,-1.));
#32391=DIRECTION('ref_axis',(-1.,0.,0.));
#32392=DIRECTION('',(1.,0.,0.));
#32393=DIRECTION('',(-1.,0.,0.));
#32394=DIRECTION('',(0.,1.,0.));
#32395=DIRECTION('center_axis',(0.939692620785909,0.,-0.342020143325667));
#32396=DIRECTION('ref_axis',(-0.342020143325667,0.,-0.939692620785909));
#32397=DIRECTION('',(0.342020143325667,0.,0.939692620785909));
#32398=DIRECTION('',(-0.342020143325667,0.,-0.939692620785909));
#32399=DIRECTION('',(0.,1.,0.));
#32400=DIRECTION('center_axis',(0.,0.,-1.));
#32401=DIRECTION('ref_axis',(-1.,0.,0.));
#32402=DIRECTION('',(1.,0.,0.));
#32403=DIRECTION('',(-1.,0.,0.));
#32404=DIRECTION('',(0.,1.,0.));
#32405=DIRECTION('center_axis',(-0.939692620785909,0.,-0.342020143325667));
#32406=DIRECTION('ref_axis',(-0.342020143325667,0.,0.939692620785909));
#32407=DIRECTION('',(0.342020143325667,0.,-0.939692620785909));
#32408=DIRECTION('',(-0.342020143325667,0.,0.939692620785909));
#32409=DIRECTION('',(0.,1.,0.));
#32410=DIRECTION('center_axis',(0.,0.,-1.));
#32411=DIRECTION('ref_axis',(-1.,0.,0.));
#32412=DIRECTION('',(1.,0.,0.));
#32413=DIRECTION('',(-1.,0.,0.));
#32414=DIRECTION('',(0.,1.,0.));
#32415=DIRECTION('center_axis',(0.939692620785909,0.,-0.342020143325667));
#32416=DIRECTION('ref_axis',(-0.342020143325667,0.,-0.939692620785909));
#32417=DIRECTION('',(0.342020143325667,0.,0.939692620785909));
#32418=DIRECTION('',(-0.342020143325667,0.,-0.939692620785909));
#32419=DIRECTION('',(0.,1.,0.));
#32420=DIRECTION('center_axis',(0.,0.,-1.));
#32421=DIRECTION('ref_axis',(-1.,0.,0.));
#32422=DIRECTION('',(1.,0.,0.));
#32423=DIRECTION('',(-1.,0.,0.));
#32424=DIRECTION('',(0.,1.,0.));
#32425=DIRECTION('center_axis',(-0.939692620785908,0.,-0.342020143325669));
#32426=DIRECTION('ref_axis',(-0.342020143325669,0.,0.939692620785908));
#32427=DIRECTION('',(0.342020143325669,0.,-0.939692620785908));
#32428=DIRECTION('',(-0.342020143325669,0.,0.939692620785908));
#32429=DIRECTION('',(0.,1.,0.));
#32430=DIRECTION('center_axis',(0.,0.,-1.));
#32431=DIRECTION('ref_axis',(-1.,0.,0.));
#32432=DIRECTION('',(1.,0.,0.));
#32433=DIRECTION('',(-1.,0.,0.));
#32434=DIRECTION('',(0.,1.,0.));
#32435=DIRECTION('center_axis',(0.939692620785908,0.,-0.342020143325669));
#32436=DIRECTION('ref_axis',(-0.342020143325669,0.,-0.939692620785908));
#32437=DIRECTION('',(0.342020143325669,0.,0.939692620785908));
#32438=DIRECTION('',(-0.342020143325669,0.,-0.939692620785908));
#32439=DIRECTION('',(0.,1.,0.));
#32440=DIRECTION('center_axis',(0.,0.,-1.));
#32441=DIRECTION('ref_axis',(-1.,0.,0.));
#32442=DIRECTION('',(1.,0.,0.));
#32443=DIRECTION('',(-1.,0.,0.));
#32444=DIRECTION('',(0.,1.,0.));
#32445=DIRECTION('center_axis',(-0.939692620785908,0.,-0.342020143325669));
#32446=DIRECTION('ref_axis',(-0.342020143325669,0.,0.939692620785908));
#32447=DIRECTION('',(0.342020143325669,0.,-0.939692620785908));
#32448=DIRECTION('',(-0.342020143325669,0.,0.939692620785908));
#32449=DIRECTION('',(0.,1.,0.));
#32450=DIRECTION('center_axis',(0.,0.,-1.));
#32451=DIRECTION('ref_axis',(-1.,0.,0.));
#32452=DIRECTION('',(1.,0.,0.));
#32453=DIRECTION('',(-1.,0.,0.));
#32454=DIRECTION('',(0.,1.,0.));
#32455=DIRECTION('center_axis',(0.939692620785908,0.,-0.342020143325669));
#32456=DIRECTION('ref_axis',(-0.342020143325669,0.,-0.939692620785908));
#32457=DIRECTION('',(0.342020143325669,0.,0.939692620785908));
#32458=DIRECTION('',(-0.342020143325669,0.,-0.939692620785908));
#32459=DIRECTION('',(0.,1.,0.));
#32460=DIRECTION('center_axis',(0.,0.,-1.));
#32461=DIRECTION('ref_axis',(-1.,0.,0.));
#32462=DIRECTION('',(1.,0.,0.));
#32463=DIRECTION('',(-1.,0.,0.));
#32464=DIRECTION('',(0.,1.,0.));
#32465=DIRECTION('center_axis',(-0.939692620785908,0.,-0.342020143325669));
#32466=DIRECTION('ref_axis',(-0.342020143325669,0.,0.939692620785908));
#32467=DIRECTION('',(0.342020143325669,0.,-0.939692620785908));
#32468=DIRECTION('',(-0.342020143325669,0.,0.939692620785908));
#32469=DIRECTION('',(0.,1.,0.));
#32470=DIRECTION('center_axis',(0.,0.,-1.));
#32471=DIRECTION('ref_axis',(-1.,0.,0.));
#32472=DIRECTION('',(1.,0.,0.));
#32473=DIRECTION('',(-1.,0.,0.));
#32474=DIRECTION('',(0.,1.,0.));
#32475=DIRECTION('center_axis',(0.939692620785908,0.,-0.342020143325669));
#32476=DIRECTION('ref_axis',(-0.342020143325669,0.,-0.939692620785908));
#32477=DIRECTION('',(0.342020143325669,0.,0.939692620785908));
#32478=DIRECTION('',(-0.342020143325669,0.,-0.939692620785908));
#32479=DIRECTION('',(0.,1.,0.));
#32480=DIRECTION('center_axis',(0.,0.,-1.));
#32481=DIRECTION('ref_axis',(-1.,0.,0.));
#32482=DIRECTION('',(1.,0.,0.));
#32483=DIRECTION('',(-1.,0.,0.));
#32484=DIRECTION('',(0.,1.,0.));
#32485=DIRECTION('center_axis',(-0.939692620785909,0.,-0.342020143325667));
#32486=DIRECTION('ref_axis',(-0.342020143325667,0.,0.939692620785909));
#32487=DIRECTION('',(0.342020143325667,0.,-0.939692620785909));
#32488=DIRECTION('',(-0.342020143325667,0.,0.939692620785909));
#32489=DIRECTION('',(0.,1.,0.));
#32490=DIRECTION('center_axis',(0.,0.,-1.));
#32491=DIRECTION('ref_axis',(-1.,0.,0.));
#32492=DIRECTION('',(1.,0.,0.));
#32493=DIRECTION('',(-1.,0.,0.));
#32494=DIRECTION('',(0.,1.,0.));
#32495=DIRECTION('center_axis',(0.939692620785908,0.,-0.342020143325669));
#32496=DIRECTION('ref_axis',(-0.342020143325669,0.,-0.939692620785908));
#32497=DIRECTION('',(0.342020143325669,0.,0.939692620785908));
#32498=DIRECTION('',(-0.342020143325669,0.,-0.939692620785908));
#32499=DIRECTION('',(0.,1.,0.));
#32500=DIRECTION('center_axis',(0.,0.,-1.));
#32501=DIRECTION('ref_axis',(-1.,0.,0.));
#32502=DIRECTION('',(1.,0.,0.));
#32503=DIRECTION('',(-1.,0.,0.));
#32504=DIRECTION('',(0.,1.,0.));
#32505=DIRECTION('center_axis',(-0.939692620785908,0.,-0.342020143325669));
#32506=DIRECTION('ref_axis',(-0.342020143325669,0.,0.939692620785908));
#32507=DIRECTION('',(0.342020143325669,0.,-0.939692620785908));
#32508=DIRECTION('',(-0.342020143325669,0.,0.939692620785908));
#32509=DIRECTION('',(0.,1.,0.));
#32510=DIRECTION('center_axis',(0.,0.,-1.));
#32511=DIRECTION('ref_axis',(-1.,0.,0.));
#32512=DIRECTION('',(1.,0.,0.));
#32513=DIRECTION('',(-1.,0.,0.));
#32514=DIRECTION('',(0.,1.,0.));
#32515=DIRECTION('center_axis',(0.939692620785908,0.,-0.342020143325669));
#32516=DIRECTION('ref_axis',(-0.342020143325669,0.,-0.939692620785908));
#32517=DIRECTION('',(0.342020143325669,0.,0.939692620785908));
#32518=DIRECTION('',(-0.342020143325669,0.,-0.939692620785908));
#32519=DIRECTION('',(0.,1.,0.));
#32520=DIRECTION('center_axis',(0.,0.,-1.));
#32521=DIRECTION('ref_axis',(-1.,0.,0.));
#32522=DIRECTION('',(1.,0.,0.));
#32523=DIRECTION('',(-1.,0.,0.));
#32524=DIRECTION('',(0.,1.,0.));
#32525=DIRECTION('center_axis',(-0.939692620785908,0.,-0.342020143325669));
#32526=DIRECTION('ref_axis',(-0.342020143325669,0.,0.939692620785908));
#32527=DIRECTION('',(0.342020143325669,0.,-0.939692620785908));
#32528=DIRECTION('',(-0.342020143325669,0.,0.939692620785908));
#32529=DIRECTION('',(0.,1.,0.));
#32530=DIRECTION('center_axis',(0.,0.,-1.));
#32531=DIRECTION('ref_axis',(-1.,0.,0.));
#32532=DIRECTION('',(1.,0.,0.));
#32533=DIRECTION('',(-1.,0.,0.));
#32534=DIRECTION('',(0.,1.,0.));
#32535=DIRECTION('center_axis',(0.939692620785908,0.,-0.342020143325669));
#32536=DIRECTION('ref_axis',(-0.342020143325669,0.,-0.939692620785908));
#32537=DIRECTION('',(0.342020143325669,0.,0.939692620785908));
#32538=DIRECTION('',(-0.342020143325669,0.,-0.939692620785908));
#32539=DIRECTION('',(0.,1.,0.));
#32540=DIRECTION('center_axis',(0.,0.,-1.));
#32541=DIRECTION('ref_axis',(-1.,0.,0.));
#32542=DIRECTION('',(1.,0.,0.));
#32543=DIRECTION('',(-1.,0.,0.));
#32544=DIRECTION('',(0.,1.,0.));
#32545=DIRECTION('center_axis',(-0.939692620785908,0.,-0.342020143325669));
#32546=DIRECTION('ref_axis',(-0.342020143325669,0.,0.939692620785908));
#32547=DIRECTION('',(0.342020143325669,0.,-0.939692620785908));
#32548=DIRECTION('',(-0.342020143325669,0.,0.939692620785908));
#32549=DIRECTION('',(0.,1.,0.));
#32550=DIRECTION('center_axis',(0.,0.,-1.));
#32551=DIRECTION('ref_axis',(-1.,0.,0.));
#32552=DIRECTION('',(1.,0.,0.));
#32553=DIRECTION('',(-1.,0.,0.));
#32554=DIRECTION('',(0.,1.,0.));
#32555=DIRECTION('center_axis',(0.939692620785908,0.,-0.342020143325669));
#32556=DIRECTION('ref_axis',(-0.342020143325669,0.,-0.939692620785908));
#32557=DIRECTION('',(0.342020143325669,0.,0.939692620785908));
#32558=DIRECTION('',(-0.342020143325669,0.,-0.939692620785908));
#32559=DIRECTION('',(0.,1.,0.));
#32560=DIRECTION('center_axis',(0.,0.,-1.));
#32561=DIRECTION('ref_axis',(-1.,0.,0.));
#32562=DIRECTION('',(1.,0.,0.));
#32563=DIRECTION('',(-1.,0.,0.));
#32564=DIRECTION('',(0.,1.,0.));
#32565=DIRECTION('center_axis',(-0.939692620785908,0.,-0.342020143325669));
#32566=DIRECTION('ref_axis',(-0.342020143325669,0.,0.939692620785908));
#32567=DIRECTION('',(0.342020143325669,0.,-0.939692620785908));
#32568=DIRECTION('',(-0.342020143325669,0.,0.939692620785908));
#32569=DIRECTION('',(0.,1.,0.));
#32570=DIRECTION('center_axis',(0.,0.,-1.));
#32571=DIRECTION('ref_axis',(-1.,0.,0.));
#32572=DIRECTION('',(1.,0.,0.));
#32573=DIRECTION('',(-1.,0.,0.));
#32574=DIRECTION('',(0.,1.,0.));
#32575=DIRECTION('center_axis',(0.939692620785908,0.,-0.342020143325669));
#32576=DIRECTION('ref_axis',(-0.342020143325669,0.,-0.939692620785908));
#32577=DIRECTION('',(0.342020143325669,0.,0.939692620785908));
#32578=DIRECTION('',(-0.342020143325669,0.,-0.939692620785908));
#32579=DIRECTION('',(0.,1.,0.));
#32580=DIRECTION('center_axis',(0.,0.,-1.));
#32581=DIRECTION('ref_axis',(-1.,0.,0.));
#32582=DIRECTION('',(1.,0.,0.));
#32583=DIRECTION('',(-1.,0.,0.));
#32584=DIRECTION('',(0.,1.,0.));
#32585=DIRECTION('center_axis',(-0.939692620785909,0.,-0.342020143325668));
#32586=DIRECTION('ref_axis',(-0.342020143325668,0.,0.939692620785909));
#32587=DIRECTION('',(0.342020143325668,0.,-0.939692620785909));
#32588=DIRECTION('',(-0.342020143325668,0.,0.939692620785909));
#32589=DIRECTION('',(0.,1.,0.));
#32590=DIRECTION('center_axis',(0.,0.,-1.));
#32591=DIRECTION('ref_axis',(-1.,0.,0.));
#32592=DIRECTION('',(1.,0.,0.));
#32593=DIRECTION('',(-1.,0.,0.));
#32594=DIRECTION('',(0.,1.,0.));
#32595=DIRECTION('center_axis',(0.939692620785908,0.,-0.342020143325669));
#32596=DIRECTION('ref_axis',(-0.342020143325669,0.,-0.939692620785908));
#32597=DIRECTION('',(0.342020143325669,0.,0.939692620785908));
#32598=DIRECTION('',(-0.342020143325669,0.,-0.939692620785908));
#32599=DIRECTION('',(0.,1.,0.));
#32600=DIRECTION('center_axis',(0.,0.,-1.));
#32601=DIRECTION('ref_axis',(-1.,0.,0.));
#32602=DIRECTION('',(1.,0.,0.));
#32603=DIRECTION('',(-1.,0.,0.));
#32604=DIRECTION('',(0.,1.,0.));
#32605=DIRECTION('center_axis',(-0.939692620785908,0.,-0.342020143325669));
#32606=DIRECTION('ref_axis',(-0.342020143325669,0.,0.939692620785908));
#32607=DIRECTION('',(0.342020143325669,0.,-0.939692620785908));
#32608=DIRECTION('',(-0.342020143325669,0.,0.939692620785908));
#32609=DIRECTION('',(0.,1.,0.));
#32610=DIRECTION('center_axis',(0.,0.,-1.));
#32611=DIRECTION('ref_axis',(-1.,0.,0.));
#32612=DIRECTION('',(1.,0.,0.));
#32613=DIRECTION('',(-1.,0.,0.));
#32614=DIRECTION('',(0.,1.,0.));
#32615=DIRECTION('center_axis',(0.939692620785908,0.,-0.34202014332567));
#32616=DIRECTION('ref_axis',(-0.34202014332567,0.,-0.939692620785908));
#32617=DIRECTION('',(0.34202014332567,0.,0.939692620785908));
#32618=DIRECTION('',(-0.34202014332567,0.,-0.939692620785908));
#32619=DIRECTION('',(0.,1.,0.));
#32620=DIRECTION('center_axis',(0.,0.,-1.));
#32621=DIRECTION('ref_axis',(-1.,0.,0.));
#32622=DIRECTION('',(1.,0.,0.));
#32623=DIRECTION('',(-1.,0.,0.));
#32624=DIRECTION('',(0.,1.,0.));
#32625=DIRECTION('center_axis',(-0.939692620785908,0.,-0.34202014332567));
#32626=DIRECTION('ref_axis',(-0.34202014332567,0.,0.939692620785908));
#32627=DIRECTION('',(0.34202014332567,0.,-0.939692620785908));
#32628=DIRECTION('',(-0.34202014332567,0.,0.939692620785908));
#32629=DIRECTION('',(0.,1.,0.));
#32630=DIRECTION('center_axis',(0.,0.,-1.));
#32631=DIRECTION('ref_axis',(-1.,0.,0.));
#32632=DIRECTION('',(1.,0.,0.));
#32633=DIRECTION('',(-1.,0.,0.));
#32634=DIRECTION('',(0.,1.,0.));
#32635=DIRECTION('center_axis',(0.939692620785908,0.,-0.342020143325669));
#32636=DIRECTION('ref_axis',(-0.342020143325669,0.,-0.939692620785908));
#32637=DIRECTION('',(0.342020143325669,0.,0.939692620785908));
#32638=DIRECTION('',(-0.342020143325669,0.,-0.939692620785908));
#32639=DIRECTION('',(0.,1.,0.));
#32640=DIRECTION('center_axis',(0.,0.,-1.));
#32641=DIRECTION('ref_axis',(-1.,0.,0.));
#32642=DIRECTION('',(1.,0.,0.));
#32643=DIRECTION('',(-1.,0.,0.));
#32644=DIRECTION('',(0.,1.,0.));
#32645=DIRECTION('center_axis',(-0.939692620785908,0.,-0.342020143325669));
#32646=DIRECTION('ref_axis',(-0.342020143325669,0.,0.939692620785908));
#32647=DIRECTION('',(0.342020143325669,0.,-0.939692620785908));
#32648=DIRECTION('',(-0.342020143325669,0.,0.939692620785908));
#32649=DIRECTION('',(0.,1.,0.));
#32650=DIRECTION('center_axis',(0.,0.,-1.));
#32651=DIRECTION('ref_axis',(-1.,0.,0.));
#32652=DIRECTION('',(1.,0.,0.));
#32653=DIRECTION('',(-1.,0.,0.));
#32654=DIRECTION('',(0.,1.,0.));
#32655=DIRECTION('center_axis',(0.939692620785908,0.,-0.34202014332567));
#32656=DIRECTION('ref_axis',(-0.34202014332567,0.,-0.939692620785908));
#32657=DIRECTION('',(0.34202014332567,0.,0.939692620785908));
#32658=DIRECTION('',(-0.34202014332567,0.,-0.939692620785908));
#32659=DIRECTION('',(0.,1.,0.));
#32660=DIRECTION('center_axis',(0.,0.,-1.));
#32661=DIRECTION('ref_axis',(-1.,0.,0.));
#32662=DIRECTION('',(1.,0.,0.));
#32663=DIRECTION('',(-1.,0.,0.));
#32664=DIRECTION('',(0.,1.,0.));
#32665=DIRECTION('center_axis',(-0.939692620785908,0.,-0.342020143325669));
#32666=DIRECTION('ref_axis',(-0.342020143325669,0.,0.939692620785908));
#32667=DIRECTION('',(0.342020143325669,0.,-0.939692620785908));
#32668=DIRECTION('',(-0.342020143325669,0.,0.939692620785908));
#32669=DIRECTION('',(0.,1.,0.));
#32670=DIRECTION('center_axis',(0.,0.,-1.));
#32671=DIRECTION('ref_axis',(-1.,0.,0.));
#32672=DIRECTION('',(1.,0.,0.));
#32673=DIRECTION('',(-1.,0.,0.));
#32674=DIRECTION('',(0.,1.,0.));
#32675=DIRECTION('center_axis',(0.939692620785908,0.,-0.342020143325669));
#32676=DIRECTION('ref_axis',(-0.342020143325669,0.,-0.939692620785908));
#32677=DIRECTION('',(0.342020143325669,0.,0.939692620785908));
#32678=DIRECTION('',(-0.342020143325669,0.,-0.939692620785908));
#32679=DIRECTION('',(0.,1.,0.));
#32680=DIRECTION('center_axis',(0.,0.,-1.));
#32681=DIRECTION('ref_axis',(-1.,0.,0.));
#32682=DIRECTION('',(1.,0.,0.));
#32683=DIRECTION('',(-1.,0.,0.));
#32684=DIRECTION('',(0.,1.,0.));
#32685=DIRECTION('center_axis',(-0.939692620785909,0.,-0.342020143325668));
#32686=DIRECTION('ref_axis',(-0.342020143325668,0.,0.939692620785909));
#32687=DIRECTION('',(0.342020143325668,0.,-0.939692620785909));
#32688=DIRECTION('',(-0.342020143325668,0.,0.939692620785909));
#32689=DIRECTION('',(0.,1.,0.));
#32690=DIRECTION('center_axis',(0.,0.,-1.));
#32691=DIRECTION('ref_axis',(-1.,0.,0.));
#32692=DIRECTION('',(1.,0.,0.));
#32693=DIRECTION('',(-1.,0.,0.));
#32694=DIRECTION('',(0.,1.,0.));
#32695=DIRECTION('center_axis',(0.939692620785908,0.,-0.342020143325669));
#32696=DIRECTION('ref_axis',(-0.342020143325669,0.,-0.939692620785908));
#32697=DIRECTION('',(0.342020143325669,0.,0.939692620785908));
#32698=DIRECTION('',(-0.342020143325669,0.,-0.939692620785908));
#32699=DIRECTION('',(0.,1.,0.));
#32700=DIRECTION('center_axis',(0.,0.,-1.));
#32701=DIRECTION('ref_axis',(-1.,0.,0.));
#32702=DIRECTION('',(1.,0.,0.));
#32703=DIRECTION('',(-1.,0.,0.));
#32704=DIRECTION('',(0.,1.,0.));
#32705=DIRECTION('center_axis',(-0.939692620785908,0.,-0.342020143325669));
#32706=DIRECTION('ref_axis',(-0.342020143325669,0.,0.939692620785908));
#32707=DIRECTION('',(0.342020143325669,0.,-0.939692620785908));
#32708=DIRECTION('',(-0.342020143325669,0.,0.939692620785908));
#32709=DIRECTION('',(0.,1.,0.));
#32710=DIRECTION('center_axis',(0.,0.,-1.));
#32711=DIRECTION('ref_axis',(-1.,0.,0.));
#32712=DIRECTION('',(1.,0.,0.));
#32713=DIRECTION('',(-1.,0.,0.));
#32714=DIRECTION('',(0.,1.,0.));
#32715=DIRECTION('center_axis',(0.939692620785908,0.,-0.342020143325669));
#32716=DIRECTION('ref_axis',(-0.342020143325669,0.,-0.939692620785908));
#32717=DIRECTION('',(0.342020143325669,0.,0.939692620785908));
#32718=DIRECTION('',(-0.342020143325669,0.,-0.939692620785908));
#32719=DIRECTION('',(0.,1.,0.));
#32720=DIRECTION('center_axis',(0.,0.,-1.));
#32721=DIRECTION('ref_axis',(-1.,0.,0.));
#32722=DIRECTION('',(1.,0.,0.));
#32723=DIRECTION('',(-1.,0.,0.));
#32724=DIRECTION('',(0.,1.,0.));
#32725=DIRECTION('center_axis',(-0.939692620785908,0.,-0.342020143325669));
#32726=DIRECTION('ref_axis',(-0.342020143325669,0.,0.939692620785908));
#32727=DIRECTION('',(0.342020143325669,0.,-0.939692620785908));
#32728=DIRECTION('',(-0.342020143325669,0.,0.939692620785908));
#32729=DIRECTION('',(0.,1.,0.));
#32730=DIRECTION('center_axis',(0.,0.,-1.));
#32731=DIRECTION('ref_axis',(-1.,0.,0.));
#32732=DIRECTION('',(1.,0.,0.));
#32733=DIRECTION('',(-1.,0.,0.));
#32734=DIRECTION('',(0.,1.,0.));
#32735=DIRECTION('center_axis',(0.939692620785908,0.,-0.342020143325669));
#32736=DIRECTION('ref_axis',(-0.342020143325669,0.,-0.939692620785908));
#32737=DIRECTION('',(0.342020143325669,0.,0.939692620785908));
#32738=DIRECTION('',(-0.342020143325669,0.,-0.939692620785908));
#32739=DIRECTION('',(0.,1.,0.));
#32740=DIRECTION('center_axis',(0.,0.,-1.));
#32741=DIRECTION('ref_axis',(-1.,0.,0.));
#32742=DIRECTION('',(1.,0.,0.));
#32743=DIRECTION('',(-1.,0.,0.));
#32744=DIRECTION('',(0.,1.,0.));
#32745=DIRECTION('center_axis',(-0.939692620785908,0.,-0.342020143325669));
#32746=DIRECTION('ref_axis',(-0.342020143325669,0.,0.939692620785908));
#32747=DIRECTION('',(0.342020143325669,0.,-0.939692620785908));
#32748=DIRECTION('',(-0.342020143325669,0.,0.939692620785908));
#32749=DIRECTION('',(0.,1.,0.));
#32750=DIRECTION('center_axis',(0.,0.,-1.));
#32751=DIRECTION('ref_axis',(-1.,0.,0.));
#32752=DIRECTION('',(1.,0.,0.));
#32753=DIRECTION('',(-1.,0.,0.));
#32754=DIRECTION('',(0.,1.,0.));
#32755=DIRECTION('center_axis',(0.939692620785908,0.,-0.342020143325669));
#32756=DIRECTION('ref_axis',(-0.342020143325669,0.,-0.939692620785908));
#32757=DIRECTION('',(0.342020143325669,0.,0.939692620785908));
#32758=DIRECTION('',(-0.342020143325669,0.,-0.939692620785908));
#32759=DIRECTION('',(0.,1.,0.));
#32760=DIRECTION('center_axis',(0.,0.,-1.));
#32761=DIRECTION('ref_axis',(-1.,0.,0.));
#32762=DIRECTION('',(1.,0.,0.));
#32763=DIRECTION('',(-1.,0.,0.));
#32764=DIRECTION('',(0.,1.,0.));
#32765=DIRECTION('center_axis',(-0.939692620785908,0.,-0.342020143325669));
#32766=DIRECTION('ref_axis',(-0.342020143325669,0.,0.939692620785908));
#32767=DIRECTION('',(0.342020143325669,0.,-0.939692620785908));
#32768=DIRECTION('',(-0.342020143325669,0.,0.939692620785908));
#32769=DIRECTION('',(0.,1.,0.));
#32770=DIRECTION('center_axis',(0.,0.,-1.));
#32771=DIRECTION('ref_axis',(-1.,0.,0.));
#32772=DIRECTION('',(1.,0.,0.));
#32773=DIRECTION('',(-1.,0.,0.));
#32774=DIRECTION('',(0.,1.,0.));
#32775=DIRECTION('center_axis',(0.939692620785908,0.,-0.342020143325669));
#32776=DIRECTION('ref_axis',(-0.342020143325669,0.,-0.939692620785908));
#32777=DIRECTION('',(0.342020143325669,0.,0.939692620785908));
#32778=DIRECTION('',(-0.342020143325669,0.,-0.939692620785908));
#32779=DIRECTION('',(0.,1.,0.));
#32780=DIRECTION('center_axis',(0.,0.,-1.));
#32781=DIRECTION('ref_axis',(-1.,0.,0.));
#32782=DIRECTION('',(1.,0.,0.));
#32783=DIRECTION('',(-1.,0.,0.));
#32784=DIRECTION('',(0.,1.,0.));
#32785=DIRECTION('center_axis',(-0.939692620785908,0.,-0.342020143325669));
#32786=DIRECTION('ref_axis',(-0.342020143325669,0.,0.939692620785908));
#32787=DIRECTION('',(0.342020143325669,0.,-0.939692620785908));
#32788=DIRECTION('',(-0.342020143325669,0.,0.939692620785908));
#32789=DIRECTION('',(0.,1.,0.));
#32790=DIRECTION('center_axis',(0.,0.,-1.));
#32791=DIRECTION('ref_axis',(-1.,0.,0.));
#32792=DIRECTION('',(1.,0.,0.));
#32793=DIRECTION('',(-1.,0.,0.));
#32794=DIRECTION('',(0.,1.,0.));
#32795=DIRECTION('center_axis',(0.939692620785909,0.,-0.342020143325668));
#32796=DIRECTION('ref_axis',(-0.342020143325668,0.,-0.939692620785909));
#32797=DIRECTION('',(0.342020143325668,0.,0.939692620785909));
#32798=DIRECTION('',(-0.342020143325668,0.,-0.939692620785909));
#32799=DIRECTION('',(0.,1.,0.));
#32800=DIRECTION('center_axis',(0.,0.,-1.));
#32801=DIRECTION('ref_axis',(-1.,0.,0.));
#32802=DIRECTION('',(1.,0.,0.));
#32803=DIRECTION('',(-1.,0.,0.));
#32804=DIRECTION('',(0.,1.,0.));
#32805=DIRECTION('center_axis',(-0.939692620785908,0.,-0.342020143325669));
#32806=DIRECTION('ref_axis',(-0.342020143325669,0.,0.939692620785908));
#32807=DIRECTION('',(0.342020143325669,0.,-0.939692620785908));
#32808=DIRECTION('',(-0.342020143325669,0.,0.939692620785908));
#32809=DIRECTION('',(0.,1.,0.));
#32810=DIRECTION('center_axis',(0.,0.,-1.));
#32811=DIRECTION('ref_axis',(-1.,0.,0.));
#32812=DIRECTION('',(1.,0.,0.));
#32813=DIRECTION('',(-1.,0.,0.));
#32814=DIRECTION('',(0.,1.,0.));
#32815=DIRECTION('center_axis',(0.939692620785908,0.,-0.342020143325669));
#32816=DIRECTION('ref_axis',(-0.342020143325669,0.,-0.939692620785908));
#32817=DIRECTION('',(0.342020143325669,0.,0.939692620785908));
#32818=DIRECTION('',(-0.342020143325669,0.,-0.939692620785908));
#32819=DIRECTION('',(0.,1.,0.));
#32820=DIRECTION('center_axis',(0.,0.,-1.));
#32821=DIRECTION('ref_axis',(-1.,0.,0.));
#32822=DIRECTION('',(1.,0.,0.));
#32823=DIRECTION('',(-1.,0.,0.));
#32824=DIRECTION('',(0.,1.,0.));
#32825=DIRECTION('center_axis',(-0.939692620785908,0.,-0.34202014332567));
#32826=DIRECTION('ref_axis',(-0.34202014332567,0.,0.939692620785908));
#32827=DIRECTION('',(0.34202014332567,0.,-0.939692620785908));
#32828=DIRECTION('',(-0.34202014332567,0.,0.939692620785908));
#32829=DIRECTION('',(0.,1.,0.));
#32830=DIRECTION('center_axis',(0.,0.,-1.));
#32831=DIRECTION('ref_axis',(-1.,0.,0.));
#32832=DIRECTION('',(1.,0.,0.));
#32833=DIRECTION('',(-1.,0.,0.));
#32834=DIRECTION('',(0.,1.,0.));
#32835=DIRECTION('center_axis',(0.939692620785908,0.,-0.342020143325669));
#32836=DIRECTION('ref_axis',(-0.342020143325669,0.,-0.939692620785908));
#32837=DIRECTION('',(0.342020143325669,0.,0.939692620785908));
#32838=DIRECTION('',(-0.342020143325669,0.,-0.939692620785908));
#32839=DIRECTION('',(0.,1.,0.));
#32840=DIRECTION('center_axis',(0.,0.,-1.));
#32841=DIRECTION('ref_axis',(-1.,0.,0.));
#32842=DIRECTION('',(1.,0.,0.));
#32843=DIRECTION('',(-1.,0.,0.));
#32844=DIRECTION('',(0.,1.,0.));
#32845=DIRECTION('center_axis',(-0.939692620785908,0.,-0.342020143325669));
#32846=DIRECTION('ref_axis',(-0.342020143325669,0.,0.939692620785908));
#32847=DIRECTION('',(0.342020143325669,0.,-0.939692620785908));
#32848=DIRECTION('',(-0.342020143325669,0.,0.939692620785908));
#32849=DIRECTION('',(0.,1.,0.));
#32850=DIRECTION('center_axis',(0.,0.,-1.));
#32851=DIRECTION('ref_axis',(-1.,0.,0.));
#32852=DIRECTION('',(1.,0.,0.));
#32853=DIRECTION('',(-1.,0.,0.));
#32854=DIRECTION('',(0.,1.,0.));
#32855=DIRECTION('center_axis',(0.939692620785908,0.,-0.34202014332567));
#32856=DIRECTION('ref_axis',(-0.34202014332567,0.,-0.939692620785908));
#32857=DIRECTION('',(0.34202014332567,0.,0.939692620785908));
#32858=DIRECTION('',(-0.34202014332567,0.,-0.939692620785908));
#32859=DIRECTION('',(0.,1.,0.));
#32860=DIRECTION('center_axis',(0.,0.,-1.));
#32861=DIRECTION('ref_axis',(-1.,0.,0.));
#32862=DIRECTION('',(1.,0.,0.));
#32863=DIRECTION('',(-1.,0.,0.));
#32864=DIRECTION('',(0.,1.,0.));
#32865=DIRECTION('center_axis',(-0.939692620785908,0.,-0.34202014332567));
#32866=DIRECTION('ref_axis',(-0.34202014332567,0.,0.939692620785908));
#32867=DIRECTION('',(0.34202014332567,0.,-0.939692620785908));
#32868=DIRECTION('',(-0.34202014332567,0.,0.939692620785908));
#32869=DIRECTION('',(0.,1.,0.));
#32870=DIRECTION('center_axis',(0.,0.,-1.));
#32871=DIRECTION('ref_axis',(-1.,0.,0.));
#32872=DIRECTION('',(1.,0.,0.));
#32873=DIRECTION('',(-1.,0.,0.));
#32874=DIRECTION('',(0.,1.,0.));
#32875=DIRECTION('center_axis',(0.939692620785908,0.,-0.342020143325669));
#32876=DIRECTION('ref_axis',(-0.342020143325669,0.,-0.939692620785908));
#32877=DIRECTION('',(0.342020143325669,0.,0.939692620785908));
#32878=DIRECTION('',(-0.342020143325669,0.,-0.939692620785908));
#32879=DIRECTION('',(0.,1.,0.));
#32880=DIRECTION('center_axis',(0.,0.,-1.));
#32881=DIRECTION('ref_axis',(-1.,0.,0.));
#32882=DIRECTION('',(1.,0.,0.));
#32883=DIRECTION('',(-1.,0.,0.));
#32884=DIRECTION('',(0.,1.,0.));
#32885=DIRECTION('center_axis',(-0.939692620785908,0.,-0.342020143325669));
#32886=DIRECTION('ref_axis',(-0.342020143325669,0.,0.939692620785908));
#32887=DIRECTION('',(0.342020143325669,0.,-0.939692620785908));
#32888=DIRECTION('',(-0.342020143325669,0.,0.939692620785908));
#32889=DIRECTION('',(0.,1.,0.));
#32890=DIRECTION('center_axis',(0.,0.,-1.));
#32891=DIRECTION('ref_axis',(-1.,0.,0.));
#32892=DIRECTION('',(1.,0.,0.));
#32893=DIRECTION('',(-1.,0.,0.));
#32894=DIRECTION('',(0.,1.,0.));
#32895=DIRECTION('center_axis',(0.939692620785909,0.,-0.342020143325668));
#32896=DIRECTION('ref_axis',(-0.342020143325668,0.,-0.939692620785909));
#32897=DIRECTION('',(0.342020143325668,0.,0.939692620785909));
#32898=DIRECTION('',(-0.342020143325668,0.,-0.939692620785909));
#32899=DIRECTION('',(0.,1.,0.));
#32900=DIRECTION('center_axis',(0.,0.,-1.));
#32901=DIRECTION('ref_axis',(-1.,0.,0.));
#32902=DIRECTION('',(1.,0.,0.));
#32903=DIRECTION('',(-1.,0.,0.));
#32904=DIRECTION('',(0.,1.,0.));
#32905=DIRECTION('center_axis',(-0.939692620785908,0.,-0.342020143325669));
#32906=DIRECTION('ref_axis',(-0.342020143325669,0.,0.939692620785908));
#32907=DIRECTION('',(0.342020143325669,0.,-0.939692620785908));
#32908=DIRECTION('',(-0.342020143325669,0.,0.939692620785908));
#32909=DIRECTION('',(0.,1.,0.));
#32910=DIRECTION('center_axis',(0.,0.,-1.));
#32911=DIRECTION('ref_axis',(-1.,0.,0.));
#32912=DIRECTION('',(1.,0.,0.));
#32913=DIRECTION('',(-1.,0.,0.));
#32914=DIRECTION('',(0.,1.,0.));
#32915=DIRECTION('center_axis',(0.939692620785908,0.,-0.342020143325669));
#32916=DIRECTION('ref_axis',(-0.342020143325669,0.,-0.939692620785908));
#32917=DIRECTION('',(0.342020143325669,0.,0.939692620785908));
#32918=DIRECTION('',(-0.342020143325669,0.,-0.939692620785908));
#32919=DIRECTION('',(0.,1.,0.));
#32920=DIRECTION('center_axis',(0.,0.,-1.));
#32921=DIRECTION('ref_axis',(-1.,0.,0.));
#32922=DIRECTION('',(1.,0.,0.));
#32923=DIRECTION('',(-1.,0.,0.));
#32924=DIRECTION('',(0.,1.,0.));
#32925=DIRECTION('center_axis',(-0.939692620785908,0.,-0.342020143325669));
#32926=DIRECTION('ref_axis',(-0.342020143325669,0.,0.939692620785908));
#32927=DIRECTION('',(0.342020143325669,0.,-0.939692620785908));
#32928=DIRECTION('',(-0.342020143325669,0.,0.939692620785908));
#32929=DIRECTION('',(0.,1.,0.));
#32930=DIRECTION('center_axis',(0.,0.,-1.));
#32931=DIRECTION('ref_axis',(-1.,0.,0.));
#32932=DIRECTION('',(1.,0.,0.));
#32933=DIRECTION('',(-1.,0.,0.));
#32934=DIRECTION('',(0.,1.,0.));
#32935=DIRECTION('center_axis',(0.939692620785908,0.,-0.342020143325669));
#32936=DIRECTION('ref_axis',(-0.342020143325669,0.,-0.939692620785908));
#32937=DIRECTION('',(0.342020143325669,0.,0.939692620785908));
#32938=DIRECTION('',(-0.342020143325669,0.,-0.939692620785908));
#32939=DIRECTION('',(0.,1.,0.));
#32940=DIRECTION('center_axis',(0.,0.,-1.));
#32941=DIRECTION('ref_axis',(-1.,0.,0.));
#32942=DIRECTION('',(1.,0.,0.));
#32943=DIRECTION('',(-1.,0.,0.));
#32944=DIRECTION('',(0.,1.,0.));
#32945=DIRECTION('center_axis',(-0.939692620785908,0.,-0.342020143325669));
#32946=DIRECTION('ref_axis',(-0.342020143325669,0.,0.939692620785908));
#32947=DIRECTION('',(0.342020143325669,0.,-0.939692620785908));
#32948=DIRECTION('',(-0.342020143325669,0.,0.939692620785908));
#32949=DIRECTION('',(0.,1.,0.));
#32950=DIRECTION('center_axis',(0.,0.,-1.));
#32951=DIRECTION('ref_axis',(-1.,0.,0.));
#32952=DIRECTION('',(1.,0.,0.));
#32953=DIRECTION('',(-1.,0.,0.));
#32954=DIRECTION('',(0.,1.,0.));
#32955=DIRECTION('center_axis',(0.939692620785908,0.,-0.342020143325669));
#32956=DIRECTION('ref_axis',(-0.342020143325669,0.,-0.939692620785908));
#32957=DIRECTION('',(0.342020143325669,0.,0.939692620785908));
#32958=DIRECTION('',(-0.342020143325669,0.,-0.939692620785908));
#32959=DIRECTION('',(0.,1.,0.));
#32960=DIRECTION('center_axis',(0.,0.,-1.));
#32961=DIRECTION('ref_axis',(-1.,0.,0.));
#32962=DIRECTION('',(1.,0.,0.));
#32963=DIRECTION('',(-1.,0.,0.));
#32964=DIRECTION('',(0.,1.,0.));
#32965=DIRECTION('center_axis',(-0.939692620785908,0.,-0.342020143325669));
#32966=DIRECTION('ref_axis',(-0.342020143325669,0.,0.939692620785908));
#32967=DIRECTION('',(0.342020143325669,0.,-0.939692620785908));
#32968=DIRECTION('',(-0.342020143325669,0.,0.939692620785908));
#32969=DIRECTION('',(0.,1.,0.));
#32970=DIRECTION('center_axis',(0.,0.,-1.));
#32971=DIRECTION('ref_axis',(-1.,0.,0.));
#32972=DIRECTION('',(1.,0.,0.));
#32973=DIRECTION('',(-1.,0.,0.));
#32974=DIRECTION('',(0.,1.,0.));
#32975=DIRECTION('center_axis',(0.939692620785908,0.,-0.342020143325669));
#32976=DIRECTION('ref_axis',(-0.342020143325669,0.,-0.939692620785908));
#32977=DIRECTION('',(0.342020143325669,0.,0.939692620785908));
#32978=DIRECTION('',(-0.342020143325669,0.,-0.939692620785908));
#32979=DIRECTION('',(0.,1.,0.));
#32980=DIRECTION('center_axis',(0.,0.,-1.));
#32981=DIRECTION('ref_axis',(-1.,0.,0.));
#32982=DIRECTION('',(1.,0.,0.));
#32983=DIRECTION('',(-1.,0.,0.));
#32984=DIRECTION('',(0.,1.,0.));
#32985=DIRECTION('center_axis',(-0.939692620785908,0.,-0.342020143325669));
#32986=DIRECTION('ref_axis',(-0.342020143325669,0.,0.939692620785908));
#32987=DIRECTION('',(0.342020143325669,0.,-0.939692620785908));
#32988=DIRECTION('',(-0.342020143325669,0.,0.939692620785908));
#32989=DIRECTION('',(0.,1.,0.));
#32990=DIRECTION('center_axis',(0.,0.,-1.));
#32991=DIRECTION('ref_axis',(-1.,0.,0.));
#32992=DIRECTION('',(1.,0.,0.));
#32993=DIRECTION('',(-1.,0.,0.));
#32994=DIRECTION('',(0.,1.,0.));
#32995=DIRECTION('center_axis',(0.939692620785909,0.,-0.342020143325667));
#32996=DIRECTION('ref_axis',(-0.342020143325667,0.,-0.939692620785909));
#32997=DIRECTION('',(0.342020143325667,0.,0.939692620785909));
#32998=DIRECTION('',(-0.342020143325667,0.,-0.939692620785909));
#32999=DIRECTION('',(0.,1.,0.));
#33000=DIRECTION('center_axis',(0.,0.,-1.));
#33001=DIRECTION('ref_axis',(-1.,0.,0.));
#33002=DIRECTION('',(1.,0.,0.));
#33003=DIRECTION('',(-1.,0.,0.));
#33004=DIRECTION('',(0.,1.,0.));
#33005=DIRECTION('center_axis',(-0.939692620785908,0.,-0.342020143325669));
#33006=DIRECTION('ref_axis',(-0.342020143325669,0.,0.939692620785908));
#33007=DIRECTION('',(0.342020143325669,0.,-0.939692620785908));
#33008=DIRECTION('',(-0.342020143325669,0.,0.939692620785908));
#33009=DIRECTION('',(0.,1.,0.));
#33010=DIRECTION('center_axis',(0.,0.,-1.));
#33011=DIRECTION('ref_axis',(-1.,0.,0.));
#33012=DIRECTION('',(1.,0.,0.));
#33013=DIRECTION('',(-1.,0.,0.));
#33014=DIRECTION('',(0.,1.,0.));
#33015=DIRECTION('center_axis',(0.939692620785908,0.,-0.342020143325669));
#33016=DIRECTION('ref_axis',(-0.342020143325669,0.,-0.939692620785908));
#33017=DIRECTION('',(0.342020143325669,0.,0.939692620785908));
#33018=DIRECTION('',(-0.342020143325669,0.,-0.939692620785908));
#33019=DIRECTION('',(0.,1.,0.));
#33020=DIRECTION('center_axis',(0.,0.,-1.));
#33021=DIRECTION('ref_axis',(-1.,0.,0.));
#33022=DIRECTION('',(1.,0.,0.));
#33023=DIRECTION('',(-1.,0.,0.));
#33024=DIRECTION('',(0.,1.,0.));
#33025=DIRECTION('center_axis',(-0.939692620785908,0.,-0.342020143325669));
#33026=DIRECTION('ref_axis',(-0.342020143325669,0.,0.939692620785908));
#33027=DIRECTION('',(0.342020143325669,0.,-0.939692620785908));
#33028=DIRECTION('',(-0.342020143325669,0.,0.939692620785908));
#33029=DIRECTION('',(0.,1.,0.));
#33030=DIRECTION('center_axis',(0.,0.,-1.));
#33031=DIRECTION('ref_axis',(-1.,0.,0.));
#33032=DIRECTION('',(1.,0.,0.));
#33033=DIRECTION('',(-1.,0.,0.));
#33034=DIRECTION('',(0.,1.,0.));
#33035=DIRECTION('center_axis',(0.939692620785908,0.,-0.342020143325669));
#33036=DIRECTION('ref_axis',(-0.342020143325669,0.,-0.939692620785908));
#33037=DIRECTION('',(0.342020143325669,0.,0.939692620785908));
#33038=DIRECTION('',(-0.342020143325669,0.,-0.939692620785908));
#33039=DIRECTION('',(0.,1.,0.));
#33040=DIRECTION('center_axis',(0.,0.,-1.));
#33041=DIRECTION('ref_axis',(-1.,0.,0.));
#33042=DIRECTION('',(1.,0.,0.));
#33043=DIRECTION('',(-1.,0.,0.));
#33044=DIRECTION('',(0.,1.,0.));
#33045=DIRECTION('center_axis',(-0.939692620785908,0.,-0.342020143325669));
#33046=DIRECTION('ref_axis',(-0.342020143325669,0.,0.939692620785908));
#33047=DIRECTION('',(0.342020143325669,0.,-0.939692620785908));
#33048=DIRECTION('',(-0.342020143325669,0.,0.939692620785908));
#33049=DIRECTION('',(0.,1.,0.));
#33050=DIRECTION('center_axis',(0.,0.,-1.));
#33051=DIRECTION('ref_axis',(-1.,0.,0.));
#33052=DIRECTION('',(1.,0.,0.));
#33053=DIRECTION('',(-1.,0.,0.));
#33054=DIRECTION('',(0.,1.,0.));
#33055=DIRECTION('center_axis',(0.939692620785908,0.,-0.342020143325669));
#33056=DIRECTION('ref_axis',(-0.342020143325669,0.,-0.939692620785908));
#33057=DIRECTION('',(0.342020143325669,0.,0.939692620785908));
#33058=DIRECTION('',(-0.342020143325669,0.,-0.939692620785908));
#33059=DIRECTION('',(0.,1.,0.));
#33060=DIRECTION('center_axis',(0.,0.,-1.));
#33061=DIRECTION('ref_axis',(-1.,0.,0.));
#33062=DIRECTION('',(1.,0.,0.));
#33063=DIRECTION('',(-1.,0.,0.));
#33064=DIRECTION('',(0.,1.,0.));
#33065=DIRECTION('center_axis',(-0.939692620785909,0.,-0.342020143325667));
#33066=DIRECTION('ref_axis',(-0.342020143325667,0.,0.939692620785909));
#33067=DIRECTION('',(0.342020143325667,0.,-0.939692620785909));
#33068=DIRECTION('',(-0.342020143325667,0.,0.939692620785909));
#33069=DIRECTION('',(0.,1.,0.));
#33070=DIRECTION('center_axis',(0.,0.,-1.));
#33071=DIRECTION('ref_axis',(-1.,0.,0.));
#33072=DIRECTION('',(1.,0.,0.));
#33073=DIRECTION('',(-1.,0.,0.));
#33074=DIRECTION('',(0.,1.,0.));
#33075=DIRECTION('center_axis',(0.939692620785909,0.,-0.342020143325667));
#33076=DIRECTION('ref_axis',(-0.342020143325667,0.,-0.939692620785909));
#33077=DIRECTION('',(0.342020143325667,0.,0.939692620785909));
#33078=DIRECTION('',(-0.342020143325667,0.,-0.939692620785909));
#33079=DIRECTION('',(0.,1.,0.));
#33080=DIRECTION('center_axis',(0.,0.,-1.));
#33081=DIRECTION('ref_axis',(-1.,0.,0.));
#33082=DIRECTION('',(1.,0.,0.));
#33083=DIRECTION('',(-1.,0.,0.));
#33084=DIRECTION('',(0.,1.,0.));
#33085=DIRECTION('center_axis',(-0.939692620785909,0.,-0.342020143325667));
#33086=DIRECTION('ref_axis',(-0.342020143325667,0.,0.939692620785909));
#33087=DIRECTION('',(0.342020143325667,0.,-0.939692620785909));
#33088=DIRECTION('',(-0.342020143325667,0.,0.939692620785909));
#33089=DIRECTION('',(0.,1.,0.));
#33090=DIRECTION('center_axis',(0.,0.,-1.));
#33091=DIRECTION('ref_axis',(-1.,0.,0.));
#33092=DIRECTION('',(1.,0.,0.));
#33093=DIRECTION('',(-1.,0.,0.));
#33094=DIRECTION('',(0.,1.,0.));
#33095=DIRECTION('center_axis',(0.939692620785909,0.,-0.342020143325667));
#33096=DIRECTION('ref_axis',(-0.342020143325667,0.,-0.939692620785909));
#33097=DIRECTION('',(0.342020143325667,0.,0.939692620785909));
#33098=DIRECTION('',(-0.342020143325667,0.,-0.939692620785909));
#33099=DIRECTION('',(0.,1.,0.));
#33100=DIRECTION('center_axis',(0.,0.,-1.));
#33101=DIRECTION('ref_axis',(-1.,0.,0.));
#33102=DIRECTION('',(1.,0.,0.));
#33103=DIRECTION('',(-1.,0.,0.));
#33104=DIRECTION('',(0.,1.,0.));
#33105=DIRECTION('center_axis',(-0.939692620785909,0.,-0.342020143325667));
#33106=DIRECTION('ref_axis',(-0.342020143325667,0.,0.939692620785909));
#33107=DIRECTION('',(0.342020143325667,0.,-0.939692620785909));
#33108=DIRECTION('',(-0.342020143325667,0.,0.939692620785909));
#33109=DIRECTION('',(0.,1.,0.));
#33110=DIRECTION('center_axis',(0.,0.,-1.));
#33111=DIRECTION('ref_axis',(-1.,0.,0.));
#33112=DIRECTION('',(1.,0.,0.));
#33113=DIRECTION('',(-1.,0.,0.));
#33114=DIRECTION('',(0.,1.,0.));
#33115=DIRECTION('center_axis',(0.939692620785908,0.,-0.342020143325671));
#33116=DIRECTION('ref_axis',(-0.342020143325671,0.,-0.939692620785908));
#33117=DIRECTION('',(0.342020143325671,0.,0.939692620785907));
#33118=DIRECTION('',(-0.342020143325671,0.,-0.939692620785907));
#33119=DIRECTION('',(0.,1.,0.));
#33120=DIRECTION('center_axis',(0.,0.,-1.));
#33121=DIRECTION('ref_axis',(-1.,0.,0.));
#33122=DIRECTION('',(1.,0.,0.));
#33123=DIRECTION('',(-1.,0.,0.));
#33124=DIRECTION('',(0.,1.,0.));
#33125=DIRECTION('center_axis',(-0.939692620785908,0.,-0.342020143325671));
#33126=DIRECTION('ref_axis',(-0.342020143325671,0.,0.939692620785908));
#33127=DIRECTION('',(0.342020143325671,0.,-0.939692620785907));
#33128=DIRECTION('',(-0.342020143325671,0.,0.939692620785907));
#33129=DIRECTION('',(0.,1.,0.));
#33130=DIRECTION('center_axis',(0.,0.,-1.));
#33131=DIRECTION('ref_axis',(-1.,0.,0.));
#33132=DIRECTION('',(1.,0.,0.));
#33133=DIRECTION('',(-1.,0.,0.));
#33134=DIRECTION('',(0.,1.,0.));
#33135=DIRECTION('center_axis',(0.939692620785908,0.,-0.342020143325671));
#33136=DIRECTION('ref_axis',(-0.342020143325671,0.,-0.939692620785908));
#33137=DIRECTION('',(0.342020143325671,0.,0.939692620785907));
#33138=DIRECTION('',(-0.342020143325671,0.,-0.939692620785907));
#33139=DIRECTION('',(0.,1.,0.));
#33140=DIRECTION('center_axis',(0.,0.,-1.));
#33141=DIRECTION('ref_axis',(-1.,0.,0.));
#33142=DIRECTION('',(1.,0.,0.));
#33143=DIRECTION('',(-1.,0.,0.));
#33144=DIRECTION('',(0.,1.,0.));
#33145=DIRECTION('center_axis',(-0.939692620785908,0.,-0.342020143325671));
#33146=DIRECTION('ref_axis',(-0.342020143325671,0.,0.939692620785908));
#33147=DIRECTION('',(0.342020143325671,0.,-0.939692620785907));
#33148=DIRECTION('',(-0.342020143325671,0.,0.939692620785907));
#33149=DIRECTION('',(0.,1.,0.));
#33150=DIRECTION('center_axis',(0.,0.,-1.));
#33151=DIRECTION('ref_axis',(-1.,0.,0.));
#33152=DIRECTION('',(1.,0.,0.));
#33153=DIRECTION('',(-1.,0.,0.));
#33154=DIRECTION('',(0.,1.,0.));
#33155=DIRECTION('center_axis',(0.939692620785908,0.,-0.342020143325671));
#33156=DIRECTION('ref_axis',(-0.342020143325671,0.,-0.939692620785908));
#33157=DIRECTION('',(0.342020143325671,0.,0.939692620785907));
#33158=DIRECTION('',(-0.342020143325671,0.,-0.939692620785907));
#33159=DIRECTION('',(0.,1.,0.));
#33160=DIRECTION('center_axis',(0.,0.,-1.));
#33161=DIRECTION('ref_axis',(-1.,0.,0.));
#33162=DIRECTION('',(1.,0.,0.));
#33163=DIRECTION('',(-1.,0.,0.));
#33164=DIRECTION('',(0.,1.,0.));
#33165=DIRECTION('center_axis',(-0.939692620785908,0.,-0.342020143325671));
#33166=DIRECTION('ref_axis',(-0.342020143325671,0.,0.939692620785908));
#33167=DIRECTION('',(0.342020143325671,0.,-0.939692620785907));
#33168=DIRECTION('',(-0.342020143325671,0.,0.939692620785907));
#33169=DIRECTION('',(0.,1.,0.));
#33170=DIRECTION('center_axis',(0.,0.,-1.));
#33171=DIRECTION('ref_axis',(-1.,0.,0.));
#33172=DIRECTION('',(1.,0.,0.));
#33173=DIRECTION('',(-1.,0.,0.));
#33174=DIRECTION('',(0.,1.,0.));
#33175=DIRECTION('center_axis',(0.939692620785909,0.,-0.342020143325667));
#33176=DIRECTION('ref_axis',(-0.342020143325667,0.,-0.939692620785909));
#33177=DIRECTION('',(0.342020143325667,0.,0.939692620785909));
#33178=DIRECTION('',(-0.342020143325667,0.,-0.939692620785909));
#33179=DIRECTION('',(0.,1.,0.));
#33180=DIRECTION('center_axis',(0.,0.,-1.));
#33181=DIRECTION('ref_axis',(-1.,0.,0.));
#33182=DIRECTION('',(1.,0.,0.));
#33183=DIRECTION('',(-1.,0.,0.));
#33184=DIRECTION('',(0.,1.,0.));
#33185=DIRECTION('center_axis',(-0.939692620785909,0.,-0.342020143325667));
#33186=DIRECTION('ref_axis',(-0.342020143325667,0.,0.939692620785909));
#33187=DIRECTION('',(0.342020143325667,0.,-0.939692620785909));
#33188=DIRECTION('',(-0.342020143325667,0.,0.939692620785909));
#33189=DIRECTION('',(0.,1.,0.));
#33190=DIRECTION('center_axis',(0.,0.,-1.));
#33191=DIRECTION('ref_axis',(-1.,0.,0.));
#33192=DIRECTION('',(1.,0.,0.));
#33193=DIRECTION('',(-1.,0.,0.));
#33194=DIRECTION('',(0.,1.,0.));
#33195=DIRECTION('center_axis',(0.939692620785909,0.,-0.342020143325667));
#33196=DIRECTION('ref_axis',(-0.342020143325667,0.,-0.939692620785909));
#33197=DIRECTION('',(0.342020143325667,0.,0.939692620785909));
#33198=DIRECTION('',(-0.342020143325667,0.,-0.939692620785909));
#33199=DIRECTION('',(0.,1.,0.));
#33200=DIRECTION('center_axis',(0.,0.,-1.));
#33201=DIRECTION('ref_axis',(-1.,0.,0.));
#33202=DIRECTION('',(1.,0.,0.));
#33203=DIRECTION('',(-1.,0.,0.));
#33204=DIRECTION('',(0.,1.,0.));
#33205=DIRECTION('center_axis',(-0.939692620785909,0.,-0.342020143325667));
#33206=DIRECTION('ref_axis',(-0.342020143325667,0.,0.939692620785909));
#33207=DIRECTION('',(0.342020143325667,0.,-0.939692620785909));
#33208=DIRECTION('',(-0.342020143325667,0.,0.939692620785909));
#33209=DIRECTION('',(0.,1.,0.));
#33210=DIRECTION('center_axis',(0.,0.,-1.));
#33211=DIRECTION('ref_axis',(-1.,0.,0.));
#33212=DIRECTION('',(1.,0.,0.));
#33213=DIRECTION('',(-1.,0.,0.));
#33214=DIRECTION('',(0.,1.,0.));
#33215=DIRECTION('center_axis',(0.939692620785909,0.,-0.342020143325667));
#33216=DIRECTION('ref_axis',(-0.342020143325667,0.,-0.939692620785909));
#33217=DIRECTION('',(0.342020143325667,0.,0.939692620785909));
#33218=DIRECTION('',(-0.342020143325667,0.,-0.939692620785909));
#33219=DIRECTION('',(0.,1.,0.));
#33220=DIRECTION('center_axis',(0.,0.,-1.));
#33221=DIRECTION('ref_axis',(-1.,0.,0.));
#33222=DIRECTION('',(1.,0.,0.));
#33223=DIRECTION('',(-1.,0.,0.));
#33224=DIRECTION('',(0.,1.,0.));
#33225=DIRECTION('center_axis',(-0.939692620785909,0.,-0.342020143325667));
#33226=DIRECTION('ref_axis',(-0.342020143325667,0.,0.939692620785909));
#33227=DIRECTION('',(0.342020143325667,0.,-0.939692620785909));
#33228=DIRECTION('',(-0.342020143325667,0.,0.939692620785909));
#33229=DIRECTION('',(0.,1.,0.));
#33230=DIRECTION('center_axis',(0.,0.,-1.));
#33231=DIRECTION('ref_axis',(-1.,0.,0.));
#33232=DIRECTION('',(1.,0.,0.));
#33233=DIRECTION('',(-1.,0.,0.));
#33234=DIRECTION('',(0.,1.,0.));
#33235=DIRECTION('center_axis',(0.939692620785908,0.,-0.342020143325671));
#33236=DIRECTION('ref_axis',(-0.342020143325671,0.,-0.939692620785908));
#33237=DIRECTION('',(0.342020143325671,0.,0.939692620785907));
#33238=DIRECTION('',(-0.342020143325671,0.,-0.939692620785907));
#33239=DIRECTION('',(0.,1.,0.));
#33240=DIRECTION('center_axis',(0.,0.,-1.));
#33241=DIRECTION('ref_axis',(-1.,0.,0.));
#33242=DIRECTION('',(1.,0.,0.));
#33243=DIRECTION('',(-1.,0.,0.));
#33244=DIRECTION('',(0.,1.,0.));
#33245=DIRECTION('center_axis',(-0.939692620785908,0.,-0.342020143325671));
#33246=DIRECTION('ref_axis',(-0.342020143325671,0.,0.939692620785908));
#33247=DIRECTION('',(0.342020143325671,0.,-0.939692620785907));
#33248=DIRECTION('',(-0.342020143325671,0.,0.939692620785907));
#33249=DIRECTION('',(0.,1.,0.));
#33250=DIRECTION('center_axis',(0.,0.,-1.));
#33251=DIRECTION('ref_axis',(-1.,0.,0.));
#33252=DIRECTION('',(1.,0.,0.));
#33253=DIRECTION('',(-1.,0.,0.));
#33254=DIRECTION('',(0.,1.,0.));
#33255=DIRECTION('center_axis',(0.939692620785908,0.,-0.342020143325671));
#33256=DIRECTION('ref_axis',(-0.342020143325671,0.,-0.939692620785908));
#33257=DIRECTION('',(0.342020143325671,0.,0.939692620785907));
#33258=DIRECTION('',(-0.342020143325671,0.,-0.939692620785907));
#33259=DIRECTION('',(0.,1.,0.));
#33260=DIRECTION('center_axis',(0.,0.,-1.));
#33261=DIRECTION('ref_axis',(-1.,0.,0.));
#33262=DIRECTION('',(1.,0.,0.));
#33263=DIRECTION('',(-1.,0.,0.));
#33264=DIRECTION('',(0.,1.,0.));
#33265=DIRECTION('center_axis',(-0.939692620785909,0.,-0.342020143325667));
#33266=DIRECTION('ref_axis',(-0.342020143325667,0.,0.939692620785909));
#33267=DIRECTION('',(0.342020143325667,0.,-0.939692620785909));
#33268=DIRECTION('',(-0.342020143325667,0.,0.939692620785909));
#33269=DIRECTION('',(0.,1.,0.));
#33270=DIRECTION('center_axis',(0.,0.,-1.));
#33271=DIRECTION('ref_axis',(-1.,0.,0.));
#33272=DIRECTION('',(1.,0.,0.));
#33273=DIRECTION('',(-1.,0.,0.));
#33274=DIRECTION('',(0.,1.,0.));
#33275=DIRECTION('center_axis',(0.939692620785909,0.,-0.342020143325667));
#33276=DIRECTION('ref_axis',(-0.342020143325667,0.,-0.939692620785909));
#33277=DIRECTION('',(0.342020143325667,0.,0.939692620785909));
#33278=DIRECTION('',(-0.342020143325667,0.,-0.939692620785909));
#33279=DIRECTION('',(0.,1.,0.));
#33280=DIRECTION('center_axis',(0.,0.,-1.));
#33281=DIRECTION('ref_axis',(-1.,0.,0.));
#33282=DIRECTION('',(1.,0.,0.));
#33283=DIRECTION('',(-1.,0.,0.));
#33284=DIRECTION('',(0.,1.,0.));
#33285=DIRECTION('center_axis',(-0.939692620785909,0.,-0.342020143325667));
#33286=DIRECTION('ref_axis',(-0.342020143325667,0.,0.939692620785909));
#33287=DIRECTION('',(0.342020143325667,0.,-0.939692620785909));
#33288=DIRECTION('',(-0.342020143325667,0.,0.939692620785909));
#33289=DIRECTION('',(0.,1.,0.));
#33290=DIRECTION('center_axis',(0.,0.,-1.));
#33291=DIRECTION('ref_axis',(-1.,0.,0.));
#33292=DIRECTION('',(1.,0.,0.));
#33293=DIRECTION('',(-1.,0.,0.));
#33294=DIRECTION('',(0.,1.,0.));
#33295=DIRECTION('center_axis',(0.939692620785909,0.,-0.342020143325667));
#33296=DIRECTION('ref_axis',(-0.342020143325667,0.,-0.939692620785909));
#33297=DIRECTION('',(0.342020143325667,0.,0.939692620785909));
#33298=DIRECTION('',(-0.342020143325667,0.,-0.939692620785909));
#33299=DIRECTION('',(0.,1.,0.));
#33300=DIRECTION('center_axis',(0.,0.,-1.));
#33301=DIRECTION('ref_axis',(-1.,0.,0.));
#33302=DIRECTION('',(1.,0.,0.));
#33303=DIRECTION('',(-1.,0.,0.));
#33304=DIRECTION('',(0.,1.,0.));
#33305=DIRECTION('center_axis',(-0.939692620785911,0.,-0.342020143325663));
#33306=DIRECTION('ref_axis',(-0.342020143325663,0.,0.939692620785911));
#33307=DIRECTION('',(0.342020143325663,0.,-0.939692620785911));
#33308=DIRECTION('',(-0.342020143325663,0.,0.939692620785911));
#33309=DIRECTION('',(0.,1.,0.));
#33310=DIRECTION('center_axis',(0.,0.,-1.));
#33311=DIRECTION('ref_axis',(-1.,0.,0.));
#33312=DIRECTION('',(1.,0.,0.));
#33313=DIRECTION('',(-1.,0.,0.));
#33314=DIRECTION('',(0.,1.,0.));
#33315=DIRECTION('center_axis',(0.939692620785911,0.,-0.342020143325663));
#33316=DIRECTION('ref_axis',(-0.342020143325663,0.,-0.939692620785911));
#33317=DIRECTION('',(0.342020143325663,0.,0.939692620785911));
#33318=DIRECTION('',(-0.342020143325663,0.,-0.939692620785911));
#33319=DIRECTION('',(0.,1.,0.));
#33320=DIRECTION('center_axis',(0.,0.,-1.));
#33321=DIRECTION('ref_axis',(-1.,0.,0.));
#33322=DIRECTION('',(1.,0.,0.));
#33323=DIRECTION('',(-1.,0.,0.));
#33324=DIRECTION('',(0.,1.,0.));
#33325=DIRECTION('center_axis',(-0.939692620785911,0.,-0.342020143325663));
#33326=DIRECTION('ref_axis',(-0.342020143325663,0.,0.939692620785911));
#33327=DIRECTION('',(0.342020143325663,0.,-0.939692620785911));
#33328=DIRECTION('',(-0.342020143325663,0.,0.939692620785911));
#33329=DIRECTION('',(0.,1.,0.));
#33330=DIRECTION('center_axis',(0.,0.,-1.));
#33331=DIRECTION('ref_axis',(-1.,0.,0.));
#33332=DIRECTION('',(1.,0.,0.));
#33333=DIRECTION('',(-1.,0.,0.));
#33334=DIRECTION('',(0.,1.,0.));
#33335=DIRECTION('center_axis',(0.939692620785911,0.,-0.342020143325663));
#33336=DIRECTION('ref_axis',(-0.342020143325663,0.,-0.939692620785911));
#33337=DIRECTION('',(0.342020143325663,0.,0.939692620785911));
#33338=DIRECTION('',(-0.342020143325663,0.,-0.939692620785911));
#33339=DIRECTION('',(0.,1.,0.));
#33340=DIRECTION('center_axis',(0.,0.,-1.));
#33341=DIRECTION('ref_axis',(-1.,0.,0.));
#33342=DIRECTION('',(1.,0.,0.));
#33343=DIRECTION('',(-1.,0.,0.));
#33344=DIRECTION('',(0.,1.,0.));
#33345=DIRECTION('center_axis',(-0.939692620785909,0.,-0.342020143325667));
#33346=DIRECTION('ref_axis',(-0.342020143325667,0.,0.939692620785909));
#33347=DIRECTION('',(0.342020143325667,0.,-0.939692620785909));
#33348=DIRECTION('',(-0.342020143325667,0.,0.939692620785909));
#33349=DIRECTION('',(0.,1.,0.));
#33350=DIRECTION('center_axis',(0.,0.,-1.));
#33351=DIRECTION('ref_axis',(-1.,0.,0.));
#33352=DIRECTION('',(1.,0.,0.));
#33353=DIRECTION('',(-1.,0.,0.));
#33354=DIRECTION('',(0.,1.,0.));
#33355=DIRECTION('center_axis',(0.939692620785909,0.,-0.342020143325667));
#33356=DIRECTION('ref_axis',(-0.342020143325667,0.,-0.939692620785909));
#33357=DIRECTION('',(0.342020143325667,0.,0.939692620785909));
#33358=DIRECTION('',(-0.342020143325667,0.,-0.939692620785909));
#33359=DIRECTION('',(0.,1.,0.));
#33360=DIRECTION('center_axis',(0.,0.,-1.));
#33361=DIRECTION('ref_axis',(-1.,0.,0.));
#33362=DIRECTION('',(1.,0.,0.));
#33363=DIRECTION('',(-1.,0.,0.));
#33364=DIRECTION('',(0.,1.,0.));
#33365=DIRECTION('center_axis',(-0.939692620785909,0.,-0.342020143325667));
#33366=DIRECTION('ref_axis',(-0.342020143325667,0.,0.939692620785909));
#33367=DIRECTION('',(0.342020143325667,0.,-0.939692620785909));
#33368=DIRECTION('',(-0.342020143325667,0.,0.939692620785909));
#33369=DIRECTION('',(0.,1.,0.));
#33370=DIRECTION('center_axis',(0.,0.,-1.));
#33371=DIRECTION('ref_axis',(-1.,0.,0.));
#33372=DIRECTION('',(1.,0.,0.));
#33373=DIRECTION('',(-1.,0.,0.));
#33374=DIRECTION('',(0.,1.,0.));
#33375=DIRECTION('center_axis',(0.939692620785909,0.,-0.342020143325667));
#33376=DIRECTION('ref_axis',(-0.342020143325667,0.,-0.939692620785909));
#33377=DIRECTION('',(0.342020143325667,0.,0.939692620785909));
#33378=DIRECTION('',(-0.342020143325667,0.,-0.939692620785909));
#33379=DIRECTION('',(0.,1.,0.));
#33380=DIRECTION('center_axis',(0.,0.,-1.));
#33381=DIRECTION('ref_axis',(-1.,0.,0.));
#33382=DIRECTION('',(1.,0.,0.));
#33383=DIRECTION('',(-1.,0.,0.));
#33384=DIRECTION('',(0.,1.,0.));
#33385=DIRECTION('center_axis',(-0.939692620785909,0.,-0.342020143325667));
#33386=DIRECTION('ref_axis',(-0.342020143325667,0.,0.939692620785909));
#33387=DIRECTION('',(0.342020143325667,0.,-0.939692620785909));
#33388=DIRECTION('',(-0.342020143325667,0.,0.939692620785909));
#33389=DIRECTION('',(0.,1.,0.));
#33390=DIRECTION('center_axis',(0.,0.,-1.));
#33391=DIRECTION('ref_axis',(-1.,0.,0.));
#33392=DIRECTION('',(1.,0.,0.));
#33393=DIRECTION('',(-1.,0.,0.));
#33394=DIRECTION('',(0.,1.,0.));
#33395=DIRECTION('center_axis',(0.939692620785909,0.,-0.342020143325667));
#33396=DIRECTION('ref_axis',(-0.342020143325667,0.,-0.939692620785909));
#33397=DIRECTION('',(0.342020143325667,0.,0.939692620785909));
#33398=DIRECTION('',(-0.342020143325667,0.,-0.939692620785909));
#33399=DIRECTION('',(0.,1.,0.));
#33400=DIRECTION('center_axis',(0.,0.,-1.));
#33401=DIRECTION('ref_axis',(-1.,0.,0.));
#33402=DIRECTION('',(1.,0.,0.));
#33403=DIRECTION('',(-1.,0.,0.));
#33404=DIRECTION('',(0.,1.,0.));
#33405=DIRECTION('center_axis',(-0.939692620785909,0.,-0.342020143325667));
#33406=DIRECTION('ref_axis',(-0.342020143325667,0.,0.939692620785909));
#33407=DIRECTION('',(0.342020143325667,0.,-0.939692620785909));
#33408=DIRECTION('',(-0.342020143325667,0.,0.939692620785909));
#33409=DIRECTION('',(0.,1.,0.));
#33410=DIRECTION('center_axis',(0.,0.,-1.));
#33411=DIRECTION('ref_axis',(-1.,0.,0.));
#33412=DIRECTION('',(1.,0.,0.));
#33413=DIRECTION('',(-1.,0.,0.));
#33414=DIRECTION('',(0.,1.,0.));
#33415=DIRECTION('center_axis',(0.939692620785909,0.,-0.342020143325667));
#33416=DIRECTION('ref_axis',(-0.342020143325667,0.,-0.939692620785909));
#33417=DIRECTION('',(0.342020143325667,0.,0.939692620785909));
#33418=DIRECTION('',(-0.342020143325667,0.,-0.939692620785909));
#33419=DIRECTION('',(0.,1.,0.));
#33420=DIRECTION('center_axis',(0.,0.,-1.));
#33421=DIRECTION('ref_axis',(-1.,0.,0.));
#33422=DIRECTION('',(1.,0.,0.));
#33423=DIRECTION('',(-1.,0.,0.));
#33424=DIRECTION('',(0.,1.,0.));
#33425=DIRECTION('center_axis',(-0.939692620785909,0.,-0.342020143325667));
#33426=DIRECTION('ref_axis',(-0.342020143325667,0.,0.939692620785909));
#33427=DIRECTION('',(0.342020143325667,0.,-0.939692620785909));
#33428=DIRECTION('',(-0.342020143325667,0.,0.939692620785909));
#33429=DIRECTION('',(0.,1.,0.));
#33430=DIRECTION('center_axis',(0.,0.,-1.));
#33431=DIRECTION('ref_axis',(-1.,0.,0.));
#33432=DIRECTION('',(1.,0.,0.));
#33433=DIRECTION('',(-1.,0.,0.));
#33434=DIRECTION('',(0.,1.,0.));
#33435=DIRECTION('center_axis',(0.939692620785909,0.,-0.342020143325667));
#33436=DIRECTION('ref_axis',(-0.342020143325667,0.,-0.939692620785909));
#33437=DIRECTION('',(0.342020143325667,0.,0.939692620785909));
#33438=DIRECTION('',(-0.342020143325667,0.,-0.939692620785909));
#33439=DIRECTION('center_axis',(0.,1.,0.));
#33440=DIRECTION('ref_axis',(1.,0.,0.));
#33441=DIRECTION('center_axis',(0.,1.,0.));
#33442=DIRECTION('ref_axis',(1.,0.,0.));
#50940=CARTESIAN_POINT('',(0.,0.,0.));
#50941=CARTESIAN_POINT('Origin',(-43.4930033668588,57.395,7.4035));
#50942=CARTESIAN_POINT('',(-87.0588007805708,57.495,7.5035));
#50943=CARTESIAN_POINT('',(-86.9860067337175,57.295,7.3035));
#50944=CARTESIAN_POINT('',(-85.229357070045,52.4686447151669,2.47714471516705));
#50945=CARTESIAN_POINT('',(-88.011,57.295,7.3035));
#50946=CARTESIAN_POINT('',(-43.4930033668588,57.295,7.3035));
#50947=CARTESIAN_POINT('',(-88.011,57.495,7.5035));
#50948=CARTESIAN_POINT('',(-88.011,57.295,7.3035));
#50949=CARTESIAN_POINT('',(-43.4930033668588,57.495,7.5035));
#50950=CARTESIAN_POINT('Origin',(-88.011,57.395,12.066));
#50951=CARTESIAN_POINT('',(-88.011,57.295,16.8285));
#50952=CARTESIAN_POINT('',(-88.011,57.495,16.6285));
#50953=CARTESIAN_POINT('',(-88.011,57.295,16.8285));
#50954=CARTESIAN_POINT('Origin',(-88.011,57.495,12.066));
#50955=CARTESIAN_POINT('Origin',(-88.011,57.295,12.066));
#50956=CARTESIAN_POINT('Origin',(-44.0055,57.395,16.7285));
#50957=CARTESIAN_POINT('',(88.011,57.295,16.8285));
#50958=CARTESIAN_POINT('',(88.011,57.495,16.6285));
#50959=CARTESIAN_POINT('',(88.011,57.295,16.8285));
#50960=CARTESIAN_POINT('',(-44.0055,57.495,16.6285));
#50961=CARTESIAN_POINT('',(-44.0055,57.295,16.8285));
#50962=CARTESIAN_POINT('Origin',(88.011,57.395,12.066));
#50963=CARTESIAN_POINT('',(88.011,57.295,7.3035));
#50964=CARTESIAN_POINT('',(88.011,57.495,7.5035));
#50965=CARTESIAN_POINT('',(88.011,57.295,7.3035));
#50966=CARTESIAN_POINT('Origin',(88.011,57.495,12.066));
#50967=CARTESIAN_POINT('Origin',(88.011,57.295,12.066));
#50968=CARTESIAN_POINT('Origin',(44.0055,57.395,7.4035));
#50969=CARTESIAN_POINT('',(86.9860067337175,57.295,7.3035));
#50970=CARTESIAN_POINT('',(87.0588007805708,57.495,7.5035));
#50971=CARTESIAN_POINT('',(85.4141633601712,52.9763958242619,2.98489582426201));
#50972=CARTESIAN_POINT('',(44.0055,57.495,7.5035));
#50973=CARTESIAN_POINT('',(44.0055,57.295,7.3035));
#50974=CARTESIAN_POINT('Origin',(88.011,54.32,7.3035));
#50975=CARTESIAN_POINT('',(88.011,54.52,7.3035));
#50976=CARTESIAN_POINT('',(88.011,54.32,7.3035));
#50977=CARTESIAN_POINT('',(86.9860067337175,54.52,7.3035));
#50978=CARTESIAN_POINT('',(44.0055,54.52,7.3035));
#50979=CARTESIAN_POINT('',(86.9860067337175,54.32,7.3035));
#50980=CARTESIAN_POINT('Origin',(88.011,54.32,12.066));
#50981=CARTESIAN_POINT('',(88.011,54.52,16.8285));
#50982=CARTESIAN_POINT('',(88.011,54.32,16.8285));
#50983=CARTESIAN_POINT('Origin',(88.011,54.52,12.066));
#50984=CARTESIAN_POINT('Origin',(-88.011,54.32,16.8285));
#50985=CARTESIAN_POINT('',(-88.011,54.52,16.8285));
#50986=CARTESIAN_POINT('',(-88.011,54.32,16.8285));
#50987=CARTESIAN_POINT('',(-44.0055,54.52,16.8285));
#50988=CARTESIAN_POINT('Origin',(-88.011,54.32,12.066));
#50989=CARTESIAN_POINT('',(-88.011,54.52,7.3035));
#50990=CARTESIAN_POINT('',(-88.011,54.32,7.3035));
#50991=CARTESIAN_POINT('Origin',(-88.011,54.52,12.066));
#50992=CARTESIAN_POINT('Origin',(-86.9860067337175,54.32,7.3035));
#50993=CARTESIAN_POINT('',(-86.9860067337175,54.52,7.3035));
#50994=CARTESIAN_POINT('',(-86.9860067337175,54.32,7.3035));
#50995=CARTESIAN_POINT('',(-43.4930033668588,54.52,7.3035));
#50996=CARTESIAN_POINT('Origin',(44.0055,54.42,7.4035));
#50997=CARTESIAN_POINT('',(87.0588007805708,54.32,7.5035));
#50998=CARTESIAN_POINT('',(85.6851174993985,58.0941637965031,3.72933620349686));
#50999=CARTESIAN_POINT('',(88.011,54.32,7.5035));
#51000=CARTESIAN_POINT('',(88.011,54.52,7.3035));
#51001=CARTESIAN_POINT('',(44.0055,54.32,7.5035));
#51002=CARTESIAN_POINT('Origin',(88.011,54.42,12.066));
#51003=CARTESIAN_POINT('',(88.011,54.32,16.6285));
#51004=CARTESIAN_POINT('',(88.011,54.52,16.8285));
#51005=CARTESIAN_POINT('Origin',(88.011,54.32,12.066));
#51006=CARTESIAN_POINT('Origin',(-44.0055,54.42,16.7285));
#51007=CARTESIAN_POINT('',(-88.011,54.32,16.6285));
#51008=CARTESIAN_POINT('',(-88.011,54.52,16.8285));
#51009=CARTESIAN_POINT('',(-44.0055,54.32,16.6285));
#51010=CARTESIAN_POINT('Origin',(-88.011,54.42,12.066));
#51011=CARTESIAN_POINT('',(-88.011,54.32,7.5035));
#51012=CARTESIAN_POINT('',(-88.011,54.52,7.3035));
#51013=CARTESIAN_POINT('Origin',(-88.011,54.32,12.066));
#51014=CARTESIAN_POINT('Origin',(-43.4930033668588,54.42,7.4035));
#51015=CARTESIAN_POINT('',(-87.0588007805708,54.32,7.5035));
#51016=CARTESIAN_POINT('',(-85.5003112092723,58.601914905598,3.22158509440188));
#51017=CARTESIAN_POINT('',(-43.4930033668588,54.32,7.5035));
#51018=CARTESIAN_POINT('Origin',(68.453,57.495,12.066));
#51019=CARTESIAN_POINT('',(66.675,57.495,12.066));
#51020=CARTESIAN_POINT('Origin',(68.453,57.495,12.066));
#51021=CARTESIAN_POINT('',(66.675,54.32,12.066));
#51022=CARTESIAN_POINT('',(66.675,57.495,12.066));
#51023=CARTESIAN_POINT('Origin',(68.453,54.32,12.066));
#51024=CARTESIAN_POINT('Origin',(29.337,57.495,12.066));
#51025=CARTESIAN_POINT('',(27.559,57.495,12.066));
#51026=CARTESIAN_POINT('Origin',(29.337,57.495,12.066));
#51027=CARTESIAN_POINT('',(27.559,54.32,12.066));
#51028=CARTESIAN_POINT('',(27.559,57.495,12.066));
#51029=CARTESIAN_POINT('Origin',(29.337,54.32,12.066));
#51030=CARTESIAN_POINT('Origin',(-88.011,57.495,12.066));
#51031=CARTESIAN_POINT('',(-89.789,57.495,12.066));
#51032=CARTESIAN_POINT('Origin',(-88.011,57.495,12.066));
#51033=CARTESIAN_POINT('',(-89.789,54.32,12.066));
#51034=CARTESIAN_POINT('',(-89.789,57.495,12.066));
#51035=CARTESIAN_POINT('Origin',(-88.011,54.32,12.066));
#51036=CARTESIAN_POINT('Origin',(-29.337,57.495,12.066));
#51037=CARTESIAN_POINT('',(-31.115,57.495,12.066));
#51038=CARTESIAN_POINT('Origin',(-29.337,57.495,12.066));
#51039=CARTESIAN_POINT('',(-31.115,54.32,12.066));
#51040=CARTESIAN_POINT('',(-31.115,57.495,12.066));
#51041=CARTESIAN_POINT('Origin',(-29.337,54.32,12.066));
#51042=CARTESIAN_POINT('Origin',(-68.453,57.495,12.066));
#51043=CARTESIAN_POINT('',(-70.231,57.495,12.066));
#51044=CARTESIAN_POINT('Origin',(-68.453,57.495,12.066));
#51045=CARTESIAN_POINT('',(-70.231,54.32,12.066));
#51046=CARTESIAN_POINT('',(-70.231,57.495,12.066));
#51047=CARTESIAN_POINT('Origin',(-68.453,54.32,12.066));
#51048=CARTESIAN_POINT('Origin',(-48.895,57.495,12.066));
#51049=CARTESIAN_POINT('',(-50.673,57.495,12.066));
#51050=CARTESIAN_POINT('Origin',(-48.895,57.495,12.066));
#51051=CARTESIAN_POINT('',(-50.673,54.32,12.066));
#51052=CARTESIAN_POINT('',(-50.673,57.495,12.066));
#51053=CARTESIAN_POINT('Origin',(-48.895,54.32,12.066));
#51054=CARTESIAN_POINT('Origin',(-9.779,57.495,12.066));
#51055=CARTESIAN_POINT('',(-11.557,57.495,12.066));
#51056=CARTESIAN_POINT('Origin',(-9.779,57.495,12.066));
#51057=CARTESIAN_POINT('',(-11.557,54.32,12.066));
#51058=CARTESIAN_POINT('',(-11.557,57.495,12.066));
#51059=CARTESIAN_POINT('Origin',(-9.779,54.32,12.066));
#51060=CARTESIAN_POINT('Origin',(9.779,57.495,12.066));
#51061=CARTESIAN_POINT('',(8.001,57.495,12.066));
#51062=CARTESIAN_POINT('Origin',(9.779,57.495,12.066));
#51063=CARTESIAN_POINT('',(8.001,54.32,12.066));
#51064=CARTESIAN_POINT('',(8.001,57.495,12.066));
#51065=CARTESIAN_POINT('Origin',(9.779,54.32,12.066));
#51066=CARTESIAN_POINT('Origin',(48.895,57.495,12.066));
#51067=CARTESIAN_POINT('',(47.117,57.495,12.066));
#51068=CARTESIAN_POINT('Origin',(48.895,57.495,12.066));
#51069=CARTESIAN_POINT('',(47.117,54.32,12.066));
#51070=CARTESIAN_POINT('',(47.117,57.495,12.066));
#51071=CARTESIAN_POINT('Origin',(48.895,54.32,12.066));
#51072=CARTESIAN_POINT('Origin',(88.011,57.495,12.066));
#51073=CARTESIAN_POINT('',(86.233,57.495,12.066));
#51074=CARTESIAN_POINT('Origin',(88.011,57.495,12.066));
#51075=CARTESIAN_POINT('',(86.233,54.32,12.066));
#51076=CARTESIAN_POINT('',(86.233,57.495,12.066));
#51077=CARTESIAN_POINT('Origin',(88.011,54.32,12.066));
#51078=CARTESIAN_POINT('Origin',(-86.3499687493374,54.32,5.556));
#51079=CARTESIAN_POINT('',(-86.3499687493374,54.32,5.556));
#51080=CARTESIAN_POINT('',(-86.9860067337175,54.32,7.3035));
#51081=CARTESIAN_POINT('',(-86.3499687493374,57.495,5.556));
#51082=CARTESIAN_POINT('',(-86.9860067337175,57.495,7.3035));
#51083=CARTESIAN_POINT('',(-86.3499687493374,54.32,5.556));
#51084=CARTESIAN_POINT('Origin',(-85.7111338969586,54.32,5.556));
#51085=CARTESIAN_POINT('',(-85.7111338969586,54.32,5.556));
#51086=CARTESIAN_POINT('',(-86.3499687493374,54.32,5.556));
#51087=CARTESIAN_POINT('',(-85.7111338969586,57.495,5.556));
#51088=CARTESIAN_POINT('',(-86.3499687493374,57.495,5.556));
#51089=CARTESIAN_POINT('',(-85.7111338969586,54.32,5.556));
#51090=CARTESIAN_POINT('Origin',(-85.0750959125784,54.32,7.3035));
#51091=CARTESIAN_POINT('',(-85.0750959125784,54.32,7.3035));
#51092=CARTESIAN_POINT('',(-85.7111338969586,54.32,5.556));
#51093=CARTESIAN_POINT('',(-85.0750959125784,57.495,7.3035));
#51094=CARTESIAN_POINT('',(-85.7111338969586,57.495,5.556));
#51095=CARTESIAN_POINT('',(-85.0750959125784,54.32,7.3035));
#51096=CARTESIAN_POINT('Origin',(-84.4923675649306,54.32,7.3035));
#51097=CARTESIAN_POINT('',(-84.4923675649306,54.32,7.3035));
#51098=CARTESIAN_POINT('',(-85.0750959125784,54.32,7.3035));
#51099=CARTESIAN_POINT('',(-84.4923675649306,57.495,7.3035));
#51100=CARTESIAN_POINT('',(-85.0750959125784,57.495,7.3035));
#51101=CARTESIAN_POINT('',(-84.4923675649306,54.32,7.3035));
#51102=CARTESIAN_POINT('Origin',(-83.8563295805504,54.32,5.556));
#51103=CARTESIAN_POINT('',(-83.8563295805504,54.32,5.556));
#51104=CARTESIAN_POINT('',(-84.4923675649306,54.32,7.3035));
#51105=CARTESIAN_POINT('',(-83.8563295805504,57.495,5.556));
#51106=CARTESIAN_POINT('',(-84.4923675649306,57.495,7.3035));
#51107=CARTESIAN_POINT('',(-83.8563295805504,54.32,5.556));
#51108=CARTESIAN_POINT('Origin',(-83.2174947281717,54.32,5.556));
#51109=CARTESIAN_POINT('',(-83.2174947281717,54.32,5.556));
#51110=CARTESIAN_POINT('',(-83.8563295805504,54.32,5.556));
#51111=CARTESIAN_POINT('',(-83.2174947281717,57.495,5.556));
#51112=CARTESIAN_POINT('',(-83.8563295805504,57.495,5.556));
#51113=CARTESIAN_POINT('',(-83.2174947281717,54.32,5.556));
#51114=CARTESIAN_POINT('Origin',(-82.5814567437915,54.32,7.3035));
#51115=CARTESIAN_POINT('',(-82.5814567437915,54.32,7.3035));
#51116=CARTESIAN_POINT('',(-83.2174947281717,54.32,5.556));
#51117=CARTESIAN_POINT('',(-82.5814567437915,57.495,7.3035));
#51118=CARTESIAN_POINT('',(-83.2174947281717,57.495,5.556));
#51119=CARTESIAN_POINT('',(-82.5814567437915,54.32,7.3035));
#51120=CARTESIAN_POINT('Origin',(-81.9987283961437,54.32,7.3035));
#51121=CARTESIAN_POINT('',(-81.9987283961437,54.32,7.3035));
#51122=CARTESIAN_POINT('',(-82.5814567437915,54.32,7.3035));
#51123=CARTESIAN_POINT('',(-81.9987283961437,57.495,7.3035));
#51124=CARTESIAN_POINT('',(-82.5814567437915,57.495,7.3035));
#51125=CARTESIAN_POINT('',(-81.9987283961437,54.32,7.3035));
#51126=CARTESIAN_POINT('Origin',(-81.3626904117636,54.32,5.556));
#51127=CARTESIAN_POINT('',(-81.3626904117636,54.32,5.556));
#51128=CARTESIAN_POINT('',(-81.9987283961437,54.32,7.3035));
#51129=CARTESIAN_POINT('',(-81.3626904117636,57.495,5.556));
#51130=CARTESIAN_POINT('',(-81.9987283961437,57.495,7.3035));
#51131=CARTESIAN_POINT('',(-81.3626904117636,54.32,5.556));
#51132=CARTESIAN_POINT('Origin',(-80.7238555593848,54.32,5.556));
#51133=CARTESIAN_POINT('',(-80.7238555593848,54.32,5.556));
#51134=CARTESIAN_POINT('',(-81.3626904117636,54.32,5.556));
#51135=CARTESIAN_POINT('',(-80.7238555593848,57.495,5.556));
#51136=CARTESIAN_POINT('',(-81.3626904117636,57.495,5.556));
#51137=CARTESIAN_POINT('',(-80.7238555593848,54.32,5.556));
#51138=CARTESIAN_POINT('Origin',(-80.0878175750046,54.32,7.3035));
#51139=CARTESIAN_POINT('',(-80.0878175750046,54.32,7.3035));
#51140=CARTESIAN_POINT('',(-80.7238555593848,54.32,5.556));
#51141=CARTESIAN_POINT('',(-80.0878175750046,57.495,7.3035));
#51142=CARTESIAN_POINT('',(-80.7238555593848,57.495,5.556));
#51143=CARTESIAN_POINT('',(-80.0878175750046,54.32,7.3035));
#51144=CARTESIAN_POINT('Origin',(-79.5050892273568,54.32,7.3035));
#51145=CARTESIAN_POINT('',(-79.5050892273568,54.32,7.3035));
#51146=CARTESIAN_POINT('',(-80.0878175750046,54.32,7.3035));
#51147=CARTESIAN_POINT('',(-79.5050892273568,57.495,7.3035));
#51148=CARTESIAN_POINT('',(-80.0878175750046,57.495,7.3035));
#51149=CARTESIAN_POINT('',(-79.5050892273568,54.32,7.3035));
#51150=CARTESIAN_POINT('Origin',(-78.8690512429767,54.32,5.556));
#51151=CARTESIAN_POINT('',(-78.8690512429767,54.32,5.556));
#51152=CARTESIAN_POINT('',(-79.5050892273568,54.32,7.3035));
#51153=CARTESIAN_POINT('',(-78.8690512429767,57.495,5.556));
#51154=CARTESIAN_POINT('',(-79.5050892273568,57.495,7.3035));
#51155=CARTESIAN_POINT('',(-78.8690512429767,54.32,5.556));
#51156=CARTESIAN_POINT('Origin',(-78.2302163905979,54.32,5.556));
#51157=CARTESIAN_POINT('',(-78.2302163905979,54.32,5.556));
#51158=CARTESIAN_POINT('',(-78.8690512429767,54.32,5.556));
#51159=CARTESIAN_POINT('',(-78.2302163905979,57.495,5.556));
#51160=CARTESIAN_POINT('',(-78.8690512429767,57.495,5.556));
#51161=CARTESIAN_POINT('',(-78.2302163905979,54.32,5.556));
#51162=CARTESIAN_POINT('Origin',(-77.5941784062178,54.32,7.3035));
#51163=CARTESIAN_POINT('',(-77.5941784062178,54.32,7.3035));
#51164=CARTESIAN_POINT('',(-78.2302163905979,54.32,5.556));
#51165=CARTESIAN_POINT('',(-77.5941784062178,57.495,7.3035));
#51166=CARTESIAN_POINT('',(-78.2302163905979,57.495,5.556));
#51167=CARTESIAN_POINT('',(-77.5941784062178,54.32,7.3035));
#51168=CARTESIAN_POINT('Origin',(-77.0114500585699,54.32,7.3035));
#51169=CARTESIAN_POINT('',(-77.0114500585699,54.32,7.3035));
#51170=CARTESIAN_POINT('',(-77.5941784062178,54.32,7.3035));
#51171=CARTESIAN_POINT('',(-77.0114500585699,57.495,7.3035));
#51172=CARTESIAN_POINT('',(-77.5941784062178,57.495,7.3035));
#51173=CARTESIAN_POINT('',(-77.0114500585699,54.32,7.3035));
#51174=CARTESIAN_POINT('Origin',(-76.3754120741898,54.32,5.556));
#51175=CARTESIAN_POINT('',(-76.3754120741898,54.32,5.556));
#51176=CARTESIAN_POINT('',(-77.0114500585699,54.32,7.3035));
#51177=CARTESIAN_POINT('',(-76.3754120741898,57.495,5.556));
#51178=CARTESIAN_POINT('',(-77.0114500585699,57.495,7.3035));
#51179=CARTESIAN_POINT('',(-76.3754120741898,54.32,5.556));
#51180=CARTESIAN_POINT('Origin',(-75.736577221811,54.32,5.556));
#51181=CARTESIAN_POINT('',(-75.736577221811,54.32,5.556));
#51182=CARTESIAN_POINT('',(-76.3754120741898,54.32,5.556));
#51183=CARTESIAN_POINT('',(-75.736577221811,57.495,5.556));
#51184=CARTESIAN_POINT('',(-76.3754120741898,57.495,5.556));
#51185=CARTESIAN_POINT('',(-75.736577221811,54.32,5.556));
#51186=CARTESIAN_POINT('Origin',(-75.1005392374309,54.32,7.3035));
#51187=CARTESIAN_POINT('',(-75.1005392374309,54.32,7.3035));
#51188=CARTESIAN_POINT('',(-75.736577221811,54.32,5.556));
#51189=CARTESIAN_POINT('',(-75.1005392374309,57.495,7.3035));
#51190=CARTESIAN_POINT('',(-75.736577221811,57.495,5.556));
#51191=CARTESIAN_POINT('',(-75.1005392374309,54.32,7.3035));
#51192=CARTESIAN_POINT('Origin',(-74.517810889783,54.32,7.3035));
#51193=CARTESIAN_POINT('',(-74.517810889783,54.32,7.3035));
#51194=CARTESIAN_POINT('',(-75.1005392374309,54.32,7.3035));
#51195=CARTESIAN_POINT('',(-74.517810889783,57.495,7.3035));
#51196=CARTESIAN_POINT('',(-75.1005392374309,57.495,7.3035));
#51197=CARTESIAN_POINT('',(-74.517810889783,54.32,7.3035));
#51198=CARTESIAN_POINT('Origin',(-73.8817729054029,54.32,5.556));
#51199=CARTESIAN_POINT('',(-73.8817729054029,54.32,5.556));
#51200=CARTESIAN_POINT('',(-74.517810889783,54.32,7.3035));
#51201=CARTESIAN_POINT('',(-73.8817729054029,57.495,5.556));
#51202=CARTESIAN_POINT('',(-74.517810889783,57.495,7.3035));
#51203=CARTESIAN_POINT('',(-73.8817729054029,54.32,5.556));
#51204=CARTESIAN_POINT('Origin',(-73.2429380530241,54.32,5.556));
#51205=CARTESIAN_POINT('',(-73.2429380530241,54.32,5.556));
#51206=CARTESIAN_POINT('',(-73.8817729054029,54.32,5.556));
#51207=CARTESIAN_POINT('',(-73.2429380530241,57.495,5.556));
#51208=CARTESIAN_POINT('',(-73.8817729054029,57.495,5.556));
#51209=CARTESIAN_POINT('',(-73.2429380530241,54.32,5.556));
#51210=CARTESIAN_POINT('Origin',(-72.606900068644,54.32,7.3035));
#51211=CARTESIAN_POINT('',(-72.606900068644,54.32,7.3035));
#51212=CARTESIAN_POINT('',(-73.2429380530241,54.32,5.556));
#51213=CARTESIAN_POINT('',(-72.606900068644,57.495,7.3035));
#51214=CARTESIAN_POINT('',(-73.2429380530241,57.495,5.556));
#51215=CARTESIAN_POINT('',(-72.606900068644,54.32,7.3035));
#51216=CARTESIAN_POINT('Origin',(-72.0241717209961,54.32,7.3035));
#51217=CARTESIAN_POINT('',(-72.0241717209961,54.32,7.3035));
#51218=CARTESIAN_POINT('',(-72.606900068644,54.32,7.3035));
#51219=CARTESIAN_POINT('',(-72.0241717209961,57.495,7.3035));
#51220=CARTESIAN_POINT('',(-72.606900068644,57.495,7.3035));
#51221=CARTESIAN_POINT('',(-72.0241717209961,54.32,7.3035));
#51222=CARTESIAN_POINT('Origin',(-71.388133736616,54.32,5.556));
#51223=CARTESIAN_POINT('',(-71.388133736616,54.32,5.556));
#51224=CARTESIAN_POINT('',(-72.0241717209961,54.32,7.3035));
#51225=CARTESIAN_POINT('',(-71.388133736616,57.495,5.556));
#51226=CARTESIAN_POINT('',(-72.0241717209961,57.495,7.3035));
#51227=CARTESIAN_POINT('',(-71.388133736616,54.32,5.556));
#51228=CARTESIAN_POINT('Origin',(-70.7492988842372,54.32,5.556));
#51229=CARTESIAN_POINT('',(-70.7492988842372,54.32,5.556));
#51230=CARTESIAN_POINT('',(-71.388133736616,54.32,5.556));
#51231=CARTESIAN_POINT('',(-70.7492988842372,57.495,5.556));
#51232=CARTESIAN_POINT('',(-71.388133736616,57.495,5.556));
#51233=CARTESIAN_POINT('',(-70.7492988842372,54.32,5.556));
#51234=CARTESIAN_POINT('Origin',(-70.1132608998571,54.32,7.3035));
#51235=CARTESIAN_POINT('',(-70.1132608998571,54.32,7.3035));
#51236=CARTESIAN_POINT('',(-70.7492988842372,54.32,5.556));
#51237=CARTESIAN_POINT('',(-70.1132608998571,57.495,7.3035));
#51238=CARTESIAN_POINT('',(-70.7492988842372,57.495,5.556));
#51239=CARTESIAN_POINT('',(-70.1132608998571,54.32,7.3035));
#51240=CARTESIAN_POINT('Origin',(-69.5305325522092,54.32,7.3035));
#51241=CARTESIAN_POINT('',(-69.5305325522092,54.32,7.3035));
#51242=CARTESIAN_POINT('',(-70.1132608998571,54.32,7.3035));
#51243=CARTESIAN_POINT('',(-69.5305325522092,57.495,7.3035));
#51244=CARTESIAN_POINT('',(-70.1132608998571,57.495,7.3035));
#51245=CARTESIAN_POINT('',(-69.5305325522092,54.32,7.3035));
#51246=CARTESIAN_POINT('Origin',(-68.8944945678291,54.32,5.556));
#51247=CARTESIAN_POINT('',(-68.8944945678291,54.32,5.556));
#51248=CARTESIAN_POINT('',(-69.5305325522092,54.32,7.3035));
#51249=CARTESIAN_POINT('',(-68.8944945678291,57.495,5.556));
#51250=CARTESIAN_POINT('',(-69.5305325522092,57.495,7.3035));
#51251=CARTESIAN_POINT('',(-68.8944945678291,54.32,5.556));
#51252=CARTESIAN_POINT('Origin',(-68.2556597154503,54.32,5.556));
#51253=CARTESIAN_POINT('',(-68.2556597154503,54.32,5.556));
#51254=CARTESIAN_POINT('',(-68.8944945678291,54.32,5.556));
#51255=CARTESIAN_POINT('',(-68.2556597154503,57.495,5.556));
#51256=CARTESIAN_POINT('',(-68.8944945678291,57.495,5.556));
#51257=CARTESIAN_POINT('',(-68.2556597154503,54.32,5.556));
#51258=CARTESIAN_POINT('Origin',(-67.6196217310702,54.32,7.3035));
#51259=CARTESIAN_POINT('',(-67.6196217310702,54.32,7.3035));
#51260=CARTESIAN_POINT('',(-68.2556597154503,54.32,5.556));
#51261=CARTESIAN_POINT('',(-67.6196217310702,57.495,7.3035));
#51262=CARTESIAN_POINT('',(-68.2556597154503,57.495,5.556));
#51263=CARTESIAN_POINT('',(-67.6196217310702,54.32,7.3035));
#51264=CARTESIAN_POINT('Origin',(-67.0368933834223,54.32,7.3035));
#51265=CARTESIAN_POINT('',(-67.0368933834223,54.32,7.3035));
#51266=CARTESIAN_POINT('',(-67.6196217310702,54.32,7.3035));
#51267=CARTESIAN_POINT('',(-67.0368933834223,57.495,7.3035));
#51268=CARTESIAN_POINT('',(-67.6196217310702,57.495,7.3035));
#51269=CARTESIAN_POINT('',(-67.0368933834223,54.32,7.3035));
#51270=CARTESIAN_POINT('Origin',(-66.4008553990422,54.32,5.556));
#51271=CARTESIAN_POINT('',(-66.4008553990422,54.32,5.556));
#51272=CARTESIAN_POINT('',(-67.0368933834223,54.32,7.3035));
#51273=CARTESIAN_POINT('',(-66.4008553990422,57.495,5.556));
#51274=CARTESIAN_POINT('',(-67.0368933834223,57.495,7.3035));
#51275=CARTESIAN_POINT('',(-66.4008553990422,54.32,5.556));
#51276=CARTESIAN_POINT('Origin',(-65.7620205466634,54.32,5.556));
#51277=CARTESIAN_POINT('',(-65.7620205466634,54.32,5.556));
#51278=CARTESIAN_POINT('',(-66.4008553990422,54.32,5.556));
#51279=CARTESIAN_POINT('',(-65.7620205466634,57.495,5.556));
#51280=CARTESIAN_POINT('',(-66.4008553990422,57.495,5.556));
#51281=CARTESIAN_POINT('',(-65.7620205466634,54.32,5.556));
#51282=CARTESIAN_POINT('Origin',(-65.1259825622833,54.32,7.3035));
#51283=CARTESIAN_POINT('',(-65.1259825622833,54.32,7.3035));
#51284=CARTESIAN_POINT('',(-65.7620205466634,54.32,5.556));
#51285=CARTESIAN_POINT('',(-65.1259825622833,57.495,7.3035));
#51286=CARTESIAN_POINT('',(-65.7620205466634,57.495,5.556));
#51287=CARTESIAN_POINT('',(-65.1259825622833,54.32,7.3035));
#51288=CARTESIAN_POINT('Origin',(-64.5432542146355,54.32,7.3035));
#51289=CARTESIAN_POINT('',(-64.5432542146355,54.32,7.3035));
#51290=CARTESIAN_POINT('',(-65.1259825622833,54.32,7.3035));
#51291=CARTESIAN_POINT('',(-64.5432542146355,57.495,7.3035));
#51292=CARTESIAN_POINT('',(-65.1259825622833,57.495,7.3035));
#51293=CARTESIAN_POINT('',(-64.5432542146355,54.32,7.3035));
#51294=CARTESIAN_POINT('Origin',(-63.9072162302553,54.32,5.556));
#51295=CARTESIAN_POINT('',(-63.9072162302553,54.32,5.556));
#51296=CARTESIAN_POINT('',(-64.5432542146355,54.32,7.3035));
#51297=CARTESIAN_POINT('',(-63.9072162302553,57.495,5.556));
#51298=CARTESIAN_POINT('',(-64.5432542146355,57.495,7.3035));
#51299=CARTESIAN_POINT('',(-63.9072162302553,54.32,5.556));
#51300=CARTESIAN_POINT('Origin',(-63.2683813778765,54.32,5.556));
#51301=CARTESIAN_POINT('',(-63.2683813778765,54.32,5.556));
#51302=CARTESIAN_POINT('',(-63.9072162302553,54.32,5.556));
#51303=CARTESIAN_POINT('',(-63.2683813778765,57.495,5.556));
#51304=CARTESIAN_POINT('',(-63.9072162302553,57.495,5.556));
#51305=CARTESIAN_POINT('',(-63.2683813778765,54.32,5.556));
#51306=CARTESIAN_POINT('Origin',(-62.6323433934964,54.32,7.3035));
#51307=CARTESIAN_POINT('',(-62.6323433934964,54.32,7.3035));
#51308=CARTESIAN_POINT('',(-63.2683813778765,54.32,5.556));
#51309=CARTESIAN_POINT('',(-62.6323433934964,57.495,7.3035));
#51310=CARTESIAN_POINT('',(-63.2683813778765,57.495,5.556));
#51311=CARTESIAN_POINT('',(-62.6323433934964,54.32,7.3035));
#51312=CARTESIAN_POINT('Origin',(-62.0496150458486,54.32,7.3035));
#51313=CARTESIAN_POINT('',(-62.0496150458486,54.32,7.3035));
#51314=CARTESIAN_POINT('',(-62.6323433934964,54.32,7.3035));
#51315=CARTESIAN_POINT('',(-62.0496150458486,57.495,7.3035));
#51316=CARTESIAN_POINT('',(-62.6323433934964,57.495,7.3035));
#51317=CARTESIAN_POINT('',(-62.0496150458486,54.32,7.3035));
#51318=CARTESIAN_POINT('Origin',(-61.4135770614684,54.32,5.556));
#51319=CARTESIAN_POINT('',(-61.4135770614684,54.32,5.556));
#51320=CARTESIAN_POINT('',(-62.0496150458486,54.32,7.3035));
#51321=CARTESIAN_POINT('',(-61.4135770614684,57.495,5.556));
#51322=CARTESIAN_POINT('',(-62.0496150458486,57.495,7.3035));
#51323=CARTESIAN_POINT('',(-61.4135770614684,54.32,5.556));
#51324=CARTESIAN_POINT('Origin',(-60.7747422090896,54.32,5.556));
#51325=CARTESIAN_POINT('',(-60.7747422090896,54.32,5.556));
#51326=CARTESIAN_POINT('',(-61.4135770614684,54.32,5.556));
#51327=CARTESIAN_POINT('',(-60.7747422090896,57.495,5.556));
#51328=CARTESIAN_POINT('',(-61.4135770614684,57.495,5.556));
#51329=CARTESIAN_POINT('',(-60.7747422090896,54.32,5.556));
#51330=CARTESIAN_POINT('Origin',(-60.1387042247095,54.32,7.3035));
#51331=CARTESIAN_POINT('',(-60.1387042247095,54.32,7.3035));
#51332=CARTESIAN_POINT('',(-60.7747422090896,54.32,5.556));
#51333=CARTESIAN_POINT('',(-60.1387042247095,57.495,7.3035));
#51334=CARTESIAN_POINT('',(-60.7747422090896,57.495,5.556));
#51335=CARTESIAN_POINT('',(-60.1387042247095,54.32,7.3035));
#51336=CARTESIAN_POINT('Origin',(-59.5559758770617,54.32,7.3035));
#51337=CARTESIAN_POINT('',(-59.5559758770617,54.32,7.3035));
#51338=CARTESIAN_POINT('',(-60.1387042247095,54.32,7.3035));
#51339=CARTESIAN_POINT('',(-59.5559758770617,57.495,7.3035));
#51340=CARTESIAN_POINT('',(-60.1387042247095,57.495,7.3035));
#51341=CARTESIAN_POINT('',(-59.5559758770617,54.32,7.3035));
#51342=CARTESIAN_POINT('Origin',(-58.9199378926815,54.32,5.556));
#51343=CARTESIAN_POINT('',(-58.9199378926815,54.32,5.556));
#51344=CARTESIAN_POINT('',(-59.5559758770617,54.32,7.3035));
#51345=CARTESIAN_POINT('',(-58.9199378926815,57.495,5.556));
#51346=CARTESIAN_POINT('',(-59.5559758770617,57.495,7.3035));
#51347=CARTESIAN_POINT('',(-58.9199378926815,54.32,5.556));
#51348=CARTESIAN_POINT('Origin',(-58.2811030403027,54.32,5.556));
#51349=CARTESIAN_POINT('',(-58.2811030403027,54.32,5.556));
#51350=CARTESIAN_POINT('',(-58.9199378926815,54.32,5.556));
#51351=CARTESIAN_POINT('',(-58.2811030403027,57.495,5.556));
#51352=CARTESIAN_POINT('',(-58.9199378926815,57.495,5.556));
#51353=CARTESIAN_POINT('',(-58.2811030403027,54.32,5.556));
#51354=CARTESIAN_POINT('Origin',(-57.6450650559226,54.32,7.3035));
#51355=CARTESIAN_POINT('',(-57.6450650559226,54.32,7.3035));
#51356=CARTESIAN_POINT('',(-58.2811030403027,54.32,5.556));
#51357=CARTESIAN_POINT('',(-57.6450650559226,57.495,7.3035));
#51358=CARTESIAN_POINT('',(-58.2811030403027,57.495,5.556));
#51359=CARTESIAN_POINT('',(-57.6450650559226,54.32,7.3035));
#51360=CARTESIAN_POINT('Origin',(-57.0623367082748,54.32,7.3035));
#51361=CARTESIAN_POINT('',(-57.0623367082748,54.32,7.3035));
#51362=CARTESIAN_POINT('',(-57.6450650559226,54.32,7.3035));
#51363=CARTESIAN_POINT('',(-57.0623367082748,57.495,7.3035));
#51364=CARTESIAN_POINT('',(-57.6450650559226,57.495,7.3035));
#51365=CARTESIAN_POINT('',(-57.0623367082748,54.32,7.3035));
#51366=CARTESIAN_POINT('Origin',(-56.4262987238946,54.32,5.556));
#51367=CARTESIAN_POINT('',(-56.4262987238946,54.32,5.556));
#51368=CARTESIAN_POINT('',(-57.0623367082748,54.32,7.3035));
#51369=CARTESIAN_POINT('',(-56.4262987238946,57.495,5.556));
#51370=CARTESIAN_POINT('',(-57.0623367082748,57.495,7.3035));
#51371=CARTESIAN_POINT('',(-56.4262987238946,54.32,5.556));
#51372=CARTESIAN_POINT('Origin',(-55.7874638715158,54.32,5.556));
#51373=CARTESIAN_POINT('',(-55.7874638715158,54.32,5.556));
#51374=CARTESIAN_POINT('',(-56.4262987238946,54.32,5.556));
#51375=CARTESIAN_POINT('',(-55.7874638715158,57.495,5.556));
#51376=CARTESIAN_POINT('',(-56.4262987238946,57.495,5.556));
#51377=CARTESIAN_POINT('',(-55.7874638715158,54.32,5.556));
#51378=CARTESIAN_POINT('Origin',(-55.1514258871357,54.32,7.3035));
#51379=CARTESIAN_POINT('',(-55.1514258871357,54.32,7.3035));
#51380=CARTESIAN_POINT('',(-55.7874638715158,54.32,5.556));
#51381=CARTESIAN_POINT('',(-55.1514258871357,57.495,7.3035));
#51382=CARTESIAN_POINT('',(-55.7874638715158,57.495,5.556));
#51383=CARTESIAN_POINT('',(-55.1514258871357,54.32,7.3035));
#51384=CARTESIAN_POINT('Origin',(-54.5686975394879,54.32,7.3035));
#51385=CARTESIAN_POINT('',(-54.5686975394879,54.32,7.3035));
#51386=CARTESIAN_POINT('',(-55.1514258871357,54.32,7.3035));
#51387=CARTESIAN_POINT('',(-54.5686975394879,57.495,7.3035));
#51388=CARTESIAN_POINT('',(-55.1514258871357,57.495,7.3035));
#51389=CARTESIAN_POINT('',(-54.5686975394879,54.32,7.3035));
#51390=CARTESIAN_POINT('Origin',(-53.9326595551077,54.32,5.556));
#51391=CARTESIAN_POINT('',(-53.9326595551077,54.32,5.556));
#51392=CARTESIAN_POINT('',(-54.5686975394879,54.32,7.3035));
#51393=CARTESIAN_POINT('',(-53.9326595551077,57.495,5.556));
#51394=CARTESIAN_POINT('',(-54.5686975394879,57.495,7.3035));
#51395=CARTESIAN_POINT('',(-53.9326595551077,54.32,5.556));
#51396=CARTESIAN_POINT('Origin',(-53.293824702729,54.32,5.556));
#51397=CARTESIAN_POINT('',(-53.293824702729,54.32,5.556));
#51398=CARTESIAN_POINT('',(-53.9326595551077,54.32,5.556));
#51399=CARTESIAN_POINT('',(-53.293824702729,57.495,5.556));
#51400=CARTESIAN_POINT('',(-53.9326595551077,57.495,5.556));
#51401=CARTESIAN_POINT('',(-53.293824702729,54.32,5.556));
#51402=CARTESIAN_POINT('Origin',(-52.6577867183488,54.32,7.3035));
#51403=CARTESIAN_POINT('',(-52.6577867183488,54.32,7.3035));
#51404=CARTESIAN_POINT('',(-53.293824702729,54.32,5.556));
#51405=CARTESIAN_POINT('',(-52.6577867183488,57.495,7.3035));
#51406=CARTESIAN_POINT('',(-53.293824702729,57.495,5.556));
#51407=CARTESIAN_POINT('',(-52.6577867183488,54.32,7.3035));
#51408=CARTESIAN_POINT('Origin',(-52.075058370701,54.32,7.3035));
#51409=CARTESIAN_POINT('',(-52.075058370701,54.32,7.3035));
#51410=CARTESIAN_POINT('',(-52.6577867183488,54.32,7.3035));
#51411=CARTESIAN_POINT('',(-52.075058370701,57.495,7.3035));
#51412=CARTESIAN_POINT('',(-52.6577867183488,57.495,7.3035));
#51413=CARTESIAN_POINT('',(-52.075058370701,54.32,7.3035));
#51414=CARTESIAN_POINT('Origin',(-51.4390203863208,54.32,5.556));
#51415=CARTESIAN_POINT('',(-51.4390203863208,54.32,5.556));
#51416=CARTESIAN_POINT('',(-52.075058370701,54.32,7.3035));
#51417=CARTESIAN_POINT('',(-51.4390203863208,57.495,5.556));
#51418=CARTESIAN_POINT('',(-52.075058370701,57.495,7.3035));
#51419=CARTESIAN_POINT('',(-51.4390203863208,54.32,5.556));
#51420=CARTESIAN_POINT('Origin',(-50.800185533942,54.32,5.556));
#51421=CARTESIAN_POINT('',(-50.800185533942,54.32,5.556));
#51422=CARTESIAN_POINT('',(-51.4390203863208,54.32,5.556));
#51423=CARTESIAN_POINT('',(-50.800185533942,57.495,5.556));
#51424=CARTESIAN_POINT('',(-51.4390203863208,57.495,5.556));
#51425=CARTESIAN_POINT('',(-50.800185533942,54.32,5.556));
#51426=CARTESIAN_POINT('Origin',(-50.1641475495619,54.32,7.3035));
#51427=CARTESIAN_POINT('',(-50.1641475495619,54.32,7.3035));
#51428=CARTESIAN_POINT('',(-50.800185533942,54.32,5.556));
#51429=CARTESIAN_POINT('',(-50.1641475495619,57.495,7.3035));
#51430=CARTESIAN_POINT('',(-50.800185533942,57.495,5.556));
#51431=CARTESIAN_POINT('',(-50.1641475495619,54.32,7.3035));
#51432=CARTESIAN_POINT('Origin',(-49.5814192019141,54.32,7.3035));
#51433=CARTESIAN_POINT('',(-49.5814192019141,54.32,7.3035));
#51434=CARTESIAN_POINT('',(-50.1641475495619,54.32,7.3035));
#51435=CARTESIAN_POINT('',(-49.5814192019141,57.495,7.3035));
#51436=CARTESIAN_POINT('',(-50.1641475495619,57.495,7.3035));
#51437=CARTESIAN_POINT('',(-49.5814192019141,54.32,7.3035));
#51438=CARTESIAN_POINT('Origin',(-48.9453812175339,54.32,5.556));
#51439=CARTESIAN_POINT('',(-48.9453812175339,54.32,5.556));
#51440=CARTESIAN_POINT('',(-49.5814192019141,54.32,7.3035));
#51441=CARTESIAN_POINT('',(-48.9453812175339,57.495,5.556));
#51442=CARTESIAN_POINT('',(-49.5814192019141,57.495,7.3035));
#51443=CARTESIAN_POINT('',(-48.9453812175339,54.32,5.556));
#51444=CARTESIAN_POINT('Origin',(-48.3065463651552,54.32,5.556));
#51445=CARTESIAN_POINT('',(-48.3065463651552,54.32,5.556));
#51446=CARTESIAN_POINT('',(-48.9453812175339,54.32,5.556));
#51447=CARTESIAN_POINT('',(-48.3065463651552,57.495,5.556));
#51448=CARTESIAN_POINT('',(-48.9453812175339,57.495,5.556));
#51449=CARTESIAN_POINT('',(-48.3065463651552,54.32,5.556));
#51450=CARTESIAN_POINT('Origin',(-47.670508380775,54.32,7.3035));
#51451=CARTESIAN_POINT('',(-47.670508380775,54.32,7.3035));
#51452=CARTESIAN_POINT('',(-48.3065463651552,54.32,5.556));
#51453=CARTESIAN_POINT('',(-47.670508380775,57.495,7.3035));
#51454=CARTESIAN_POINT('',(-48.3065463651552,57.495,5.556));
#51455=CARTESIAN_POINT('',(-47.670508380775,54.32,7.3035));
#51456=CARTESIAN_POINT('Origin',(-47.0877800331272,54.32,7.3035));
#51457=CARTESIAN_POINT('',(-47.0877800331272,54.32,7.3035));
#51458=CARTESIAN_POINT('',(-47.670508380775,54.32,7.3035));
#51459=CARTESIAN_POINT('',(-47.0877800331272,57.495,7.3035));
#51460=CARTESIAN_POINT('',(-47.670508380775,57.495,7.3035));
#51461=CARTESIAN_POINT('',(-47.0877800331272,54.32,7.3035));
#51462=CARTESIAN_POINT('Origin',(-46.451742048747,54.32,5.556));
#51463=CARTESIAN_POINT('',(-46.451742048747,54.32,5.556));
#51464=CARTESIAN_POINT('',(-47.0877800331272,54.32,7.3035));
#51465=CARTESIAN_POINT('',(-46.451742048747,57.495,5.556));
#51466=CARTESIAN_POINT('',(-47.0877800331272,57.495,7.3035));
#51467=CARTESIAN_POINT('',(-46.451742048747,54.32,5.556));
#51468=CARTESIAN_POINT('Origin',(-45.8129071963683,54.32,5.556));
#51469=CARTESIAN_POINT('',(-45.8129071963683,54.32,5.556));
#51470=CARTESIAN_POINT('',(-46.451742048747,54.32,5.556));
#51471=CARTESIAN_POINT('',(-45.8129071963683,57.495,5.556));
#51472=CARTESIAN_POINT('',(-46.451742048747,57.495,5.556));
#51473=CARTESIAN_POINT('',(-45.8129071963683,54.32,5.556));
#51474=CARTESIAN_POINT('Origin',(-45.1768692119881,54.32,7.3035));
#51475=CARTESIAN_POINT('',(-45.1768692119881,54.32,7.3035));
#51476=CARTESIAN_POINT('',(-45.8129071963683,54.32,5.556));
#51477=CARTESIAN_POINT('',(-45.1768692119881,57.495,7.3035));
#51478=CARTESIAN_POINT('',(-45.8129071963683,57.495,5.556));
#51479=CARTESIAN_POINT('',(-45.1768692119881,54.32,7.3035));
#51480=CARTESIAN_POINT('Origin',(-44.5941408643403,54.32,7.3035));
#51481=CARTESIAN_POINT('',(-44.5941408643403,54.32,7.3035));
#51482=CARTESIAN_POINT('',(-45.1768692119881,54.32,7.3035));
#51483=CARTESIAN_POINT('',(-44.5941408643403,57.495,7.3035));
#51484=CARTESIAN_POINT('',(-45.1768692119881,57.495,7.3035));
#51485=CARTESIAN_POINT('',(-44.5941408643403,54.32,7.3035));
#51486=CARTESIAN_POINT('Origin',(-43.9581028799601,54.32,5.556));
#51487=CARTESIAN_POINT('',(-43.9581028799601,54.32,5.556));
#51488=CARTESIAN_POINT('',(-44.5941408643403,54.32,7.3035));
#51489=CARTESIAN_POINT('',(-43.9581028799601,57.495,5.556));
#51490=CARTESIAN_POINT('',(-44.5941408643403,57.495,7.3035));
#51491=CARTESIAN_POINT('',(-43.9581028799601,54.32,5.556));
#51492=CARTESIAN_POINT('Origin',(-43.3192680275814,54.32,5.556));
#51493=CARTESIAN_POINT('',(-43.3192680275814,54.32,5.556));
#51494=CARTESIAN_POINT('',(-43.9581028799601,54.32,5.556));
#51495=CARTESIAN_POINT('',(-43.3192680275814,57.495,5.556));
#51496=CARTESIAN_POINT('',(-43.9581028799601,57.495,5.556));
#51497=CARTESIAN_POINT('',(-43.3192680275814,54.32,5.556));
#51498=CARTESIAN_POINT('Origin',(-42.6832300432012,54.32,7.3035));
#51499=CARTESIAN_POINT('',(-42.6832300432012,54.32,7.3035));
#51500=CARTESIAN_POINT('',(-43.3192680275814,54.32,5.556));
#51501=CARTESIAN_POINT('',(-42.6832300432012,57.495,7.3035));
#51502=CARTESIAN_POINT('',(-43.3192680275814,57.495,5.556));
#51503=CARTESIAN_POINT('',(-42.6832300432012,54.32,7.3035));
#51504=CARTESIAN_POINT('Origin',(-42.1005016955534,54.32,7.3035));
#51505=CARTESIAN_POINT('',(-42.1005016955534,54.32,7.3035));
#51506=CARTESIAN_POINT('',(-42.6832300432012,54.32,7.3035));
#51507=CARTESIAN_POINT('',(-42.1005016955534,57.495,7.3035));
#51508=CARTESIAN_POINT('',(-42.6832300432012,57.495,7.3035));
#51509=CARTESIAN_POINT('',(-42.1005016955534,54.32,7.3035));
#51510=CARTESIAN_POINT('Origin',(-41.4644637111732,54.32,5.556));
#51511=CARTESIAN_POINT('',(-41.4644637111732,54.32,5.556));
#51512=CARTESIAN_POINT('',(-42.1005016955534,54.32,7.3035));
#51513=CARTESIAN_POINT('',(-41.4644637111732,57.495,5.556));
#51514=CARTESIAN_POINT('',(-42.1005016955534,57.495,7.3035));
#51515=CARTESIAN_POINT('',(-41.4644637111732,54.32,5.556));
#51516=CARTESIAN_POINT('Origin',(-40.8256288587945,54.32,5.556));
#51517=CARTESIAN_POINT('',(-40.8256288587945,54.32,5.556));
#51518=CARTESIAN_POINT('',(-41.4644637111732,54.32,5.556));
#51519=CARTESIAN_POINT('',(-40.8256288587945,57.495,5.556));
#51520=CARTESIAN_POINT('',(-41.4644637111732,57.495,5.556));
#51521=CARTESIAN_POINT('',(-40.8256288587945,54.32,5.556));
#51522=CARTESIAN_POINT('Origin',(-40.1895908744143,54.32,7.3035));
#51523=CARTESIAN_POINT('',(-40.1895908744143,54.32,7.3035));
#51524=CARTESIAN_POINT('',(-40.8256288587945,54.32,5.556));
#51525=CARTESIAN_POINT('',(-40.1895908744143,57.495,7.3035));
#51526=CARTESIAN_POINT('',(-40.8256288587945,57.495,5.556));
#51527=CARTESIAN_POINT('',(-40.1895908744143,54.32,7.3035));
#51528=CARTESIAN_POINT('Origin',(-39.6068625267665,54.32,7.3035));
#51529=CARTESIAN_POINT('',(-39.6068625267665,54.32,7.3035));
#51530=CARTESIAN_POINT('',(-40.1895908744143,54.32,7.3035));
#51531=CARTESIAN_POINT('',(-39.6068625267665,57.495,7.3035));
#51532=CARTESIAN_POINT('',(-40.1895908744143,57.495,7.3035));
#51533=CARTESIAN_POINT('',(-39.6068625267665,54.32,7.3035));
#51534=CARTESIAN_POINT('Origin',(-38.9708245423863,54.32,5.556));
#51535=CARTESIAN_POINT('',(-38.9708245423863,54.32,5.556));
#51536=CARTESIAN_POINT('',(-39.6068625267665,54.32,7.3035));
#51537=CARTESIAN_POINT('',(-38.9708245423863,57.495,5.556));
#51538=CARTESIAN_POINT('',(-39.6068625267665,57.495,7.3035));
#51539=CARTESIAN_POINT('',(-38.9708245423863,54.32,5.556));
#51540=CARTESIAN_POINT('Origin',(-38.3319896900076,54.32,5.556));
#51541=CARTESIAN_POINT('',(-38.3319896900076,54.32,5.556));
#51542=CARTESIAN_POINT('',(-38.9708245423863,54.32,5.556));
#51543=CARTESIAN_POINT('',(-38.3319896900076,57.495,5.556));
#51544=CARTESIAN_POINT('',(-38.9708245423863,57.495,5.556));
#51545=CARTESIAN_POINT('',(-38.3319896900076,54.32,5.556));
#51546=CARTESIAN_POINT('Origin',(-37.6959517056274,54.32,7.3035));
#51547=CARTESIAN_POINT('',(-37.6959517056274,54.32,7.3035));
#51548=CARTESIAN_POINT('',(-38.3319896900076,54.32,5.556));
#51549=CARTESIAN_POINT('',(-37.6959517056274,57.495,7.3035));
#51550=CARTESIAN_POINT('',(-38.3319896900076,57.495,5.556));
#51551=CARTESIAN_POINT('',(-37.6959517056274,54.32,7.3035));
#51552=CARTESIAN_POINT('Origin',(-37.1132233579796,54.32,7.3035));
#51553=CARTESIAN_POINT('',(-37.1132233579796,54.32,7.3035));
#51554=CARTESIAN_POINT('',(-37.6959517056274,54.32,7.3035));
#51555=CARTESIAN_POINT('',(-37.1132233579796,57.495,7.3035));
#51556=CARTESIAN_POINT('',(-37.6959517056274,57.495,7.3035));
#51557=CARTESIAN_POINT('',(-37.1132233579796,54.32,7.3035));
#51558=CARTESIAN_POINT('Origin',(-36.4771853735994,54.32,5.556));
#51559=CARTESIAN_POINT('',(-36.4771853735994,54.32,5.556));
#51560=CARTESIAN_POINT('',(-37.1132233579796,54.32,7.3035));
#51561=CARTESIAN_POINT('',(-36.4771853735994,57.495,5.556));
#51562=CARTESIAN_POINT('',(-37.1132233579796,57.495,7.3035));
#51563=CARTESIAN_POINT('',(-36.4771853735994,54.32,5.556));
#51564=CARTESIAN_POINT('Origin',(-35.8383505212207,54.32,5.556));
#51565=CARTESIAN_POINT('',(-35.8383505212207,54.32,5.556));
#51566=CARTESIAN_POINT('',(-36.4771853735994,54.32,5.556));
#51567=CARTESIAN_POINT('',(-35.8383505212207,57.495,5.556));
#51568=CARTESIAN_POINT('',(-36.4771853735994,57.495,5.556));
#51569=CARTESIAN_POINT('',(-35.8383505212207,54.32,5.556));
#51570=CARTESIAN_POINT('Origin',(-35.2023125368405,54.32,7.3035));
#51571=CARTESIAN_POINT('',(-35.2023125368405,54.32,7.3035));
#51572=CARTESIAN_POINT('',(-35.8383505212207,54.32,5.556));
#51573=CARTESIAN_POINT('',(-35.2023125368405,57.495,7.3035));
#51574=CARTESIAN_POINT('',(-35.8383505212207,57.495,5.556));
#51575=CARTESIAN_POINT('',(-35.2023125368405,54.32,7.3035));
#51576=CARTESIAN_POINT('Origin',(-34.6195841891927,54.32,7.3035));
#51577=CARTESIAN_POINT('',(-34.6195841891927,54.32,7.3035));
#51578=CARTESIAN_POINT('',(-35.2023125368405,54.32,7.3035));
#51579=CARTESIAN_POINT('',(-34.6195841891927,57.495,7.3035));
#51580=CARTESIAN_POINT('',(-35.2023125368405,57.495,7.3035));
#51581=CARTESIAN_POINT('',(-34.6195841891927,54.32,7.3035));
#51582=CARTESIAN_POINT('Origin',(-33.9835462048125,54.32,5.556));
#51583=CARTESIAN_POINT('',(-33.9835462048125,54.32,5.556));
#51584=CARTESIAN_POINT('',(-34.6195841891927,54.32,7.3035));
#51585=CARTESIAN_POINT('',(-33.9835462048125,57.495,5.556));
#51586=CARTESIAN_POINT('',(-34.6195841891927,57.495,7.3035));
#51587=CARTESIAN_POINT('',(-33.9835462048125,54.32,5.556));
#51588=CARTESIAN_POINT('Origin',(-33.3447113524338,54.32,5.556));
#51589=CARTESIAN_POINT('',(-33.3447113524338,54.32,5.556));
#51590=CARTESIAN_POINT('',(-33.9835462048125,54.32,5.556));
#51591=CARTESIAN_POINT('',(-33.3447113524338,57.495,5.556));
#51592=CARTESIAN_POINT('',(-33.9835462048125,57.495,5.556));
#51593=CARTESIAN_POINT('',(-33.3447113524338,54.32,5.556));
#51594=CARTESIAN_POINT('Origin',(-32.7086733680536,54.32,7.3035));
#51595=CARTESIAN_POINT('',(-32.7086733680536,54.32,7.3035));
#51596=CARTESIAN_POINT('',(-33.3447113524338,54.32,5.556));
#51597=CARTESIAN_POINT('',(-32.7086733680536,57.495,7.3035));
#51598=CARTESIAN_POINT('',(-33.3447113524338,57.495,5.556));
#51599=CARTESIAN_POINT('',(-32.7086733680536,54.32,7.3035));
#51600=CARTESIAN_POINT('Origin',(-32.1259450204058,54.32,7.3035));
#51601=CARTESIAN_POINT('',(-32.1259450204058,54.32,7.3035));
#51602=CARTESIAN_POINT('',(-32.7086733680536,54.32,7.3035));
#51603=CARTESIAN_POINT('',(-32.1259450204058,57.495,7.3035));
#51604=CARTESIAN_POINT('',(-32.7086733680536,57.495,7.3035));
#51605=CARTESIAN_POINT('',(-32.1259450204058,54.32,7.3035));
#51606=CARTESIAN_POINT('Origin',(-31.4899070360256,54.32,5.556));
#51607=CARTESIAN_POINT('',(-31.4899070360256,54.32,5.556));
#51608=CARTESIAN_POINT('',(-32.1259450204058,54.32,7.3035));
#51609=CARTESIAN_POINT('',(-31.4899070360256,57.495,5.556));
#51610=CARTESIAN_POINT('',(-32.1259450204058,57.495,7.3035));
#51611=CARTESIAN_POINT('',(-31.4899070360256,54.32,5.556));
#51612=CARTESIAN_POINT('Origin',(-30.8510721836469,54.32,5.556));
#51613=CARTESIAN_POINT('',(-30.8510721836469,54.32,5.556));
#51614=CARTESIAN_POINT('',(-31.4899070360256,54.32,5.556));
#51615=CARTESIAN_POINT('',(-30.8510721836469,57.495,5.556));
#51616=CARTESIAN_POINT('',(-31.4899070360256,57.495,5.556));
#51617=CARTESIAN_POINT('',(-30.8510721836469,54.32,5.556));
#51618=CARTESIAN_POINT('Origin',(-30.2150341992667,54.32,7.3035));
#51619=CARTESIAN_POINT('',(-30.2150341992667,54.32,7.3035));
#51620=CARTESIAN_POINT('',(-30.8510721836469,54.32,5.556));
#51621=CARTESIAN_POINT('',(-30.2150341992667,57.495,7.3035));
#51622=CARTESIAN_POINT('',(-30.8510721836469,57.495,5.556));
#51623=CARTESIAN_POINT('',(-30.2150341992667,54.32,7.3035));
#51624=CARTESIAN_POINT('Origin',(-29.6323058516189,54.32,7.3035));
#51625=CARTESIAN_POINT('',(-29.6323058516189,54.32,7.3035));
#51626=CARTESIAN_POINT('',(-30.2150341992667,54.32,7.3035));
#51627=CARTESIAN_POINT('',(-29.6323058516189,57.495,7.3035));
#51628=CARTESIAN_POINT('',(-30.2150341992667,57.495,7.3035));
#51629=CARTESIAN_POINT('',(-29.6323058516189,54.32,7.3035));
#51630=CARTESIAN_POINT('Origin',(-28.9962678672387,54.32,5.556));
#51631=CARTESIAN_POINT('',(-28.9962678672387,54.32,5.556));
#51632=CARTESIAN_POINT('',(-29.6323058516189,54.32,7.3035));
#51633=CARTESIAN_POINT('',(-28.9962678672387,57.495,5.556));
#51634=CARTESIAN_POINT('',(-29.6323058516189,57.495,7.3035));
#51635=CARTESIAN_POINT('',(-28.9962678672387,54.32,5.556));
#51636=CARTESIAN_POINT('Origin',(-28.35743301486,54.32,5.556));
#51637=CARTESIAN_POINT('',(-28.35743301486,54.32,5.556));
#51638=CARTESIAN_POINT('',(-28.9962678672387,54.32,5.556));
#51639=CARTESIAN_POINT('',(-28.35743301486,57.495,5.556));
#51640=CARTESIAN_POINT('',(-28.9962678672387,57.495,5.556));
#51641=CARTESIAN_POINT('',(-28.35743301486,54.32,5.556));
#51642=CARTESIAN_POINT('Origin',(-27.7213950304798,54.32,7.3035));
#51643=CARTESIAN_POINT('',(-27.7213950304798,54.32,7.3035));
#51644=CARTESIAN_POINT('',(-28.35743301486,54.32,5.556));
#51645=CARTESIAN_POINT('',(-27.7213950304798,57.495,7.3035));
#51646=CARTESIAN_POINT('',(-28.35743301486,57.495,5.556));
#51647=CARTESIAN_POINT('',(-27.7213950304798,54.32,7.3035));
#51648=CARTESIAN_POINT('Origin',(-27.138666682832,54.32,7.3035));
#51649=CARTESIAN_POINT('',(-27.138666682832,54.32,7.3035));
#51650=CARTESIAN_POINT('',(-27.7213950304798,54.32,7.3035));
#51651=CARTESIAN_POINT('',(-27.138666682832,57.495,7.3035));
#51652=CARTESIAN_POINT('',(-27.7213950304798,57.495,7.3035));
#51653=CARTESIAN_POINT('',(-27.138666682832,54.32,7.3035));
#51654=CARTESIAN_POINT('Origin',(-26.5026286984518,54.32,5.556));
#51655=CARTESIAN_POINT('',(-26.5026286984518,54.32,5.556));
#51656=CARTESIAN_POINT('',(-27.138666682832,54.32,7.3035));
#51657=CARTESIAN_POINT('',(-26.5026286984518,57.495,5.556));
#51658=CARTESIAN_POINT('',(-27.138666682832,57.495,7.3035));
#51659=CARTESIAN_POINT('',(-26.5026286984518,54.32,5.556));
#51660=CARTESIAN_POINT('Origin',(-25.8637938460731,54.32,5.556));
#51661=CARTESIAN_POINT('',(-25.8637938460731,54.32,5.556));
#51662=CARTESIAN_POINT('',(-26.5026286984518,54.32,5.556));
#51663=CARTESIAN_POINT('',(-25.8637938460731,57.495,5.556));
#51664=CARTESIAN_POINT('',(-26.5026286984518,57.495,5.556));
#51665=CARTESIAN_POINT('',(-25.8637938460731,54.32,5.556));
#51666=CARTESIAN_POINT('Origin',(-25.2277558616929,54.32,7.3035));
#51667=CARTESIAN_POINT('',(-25.2277558616929,54.32,7.3035));
#51668=CARTESIAN_POINT('',(-25.8637938460731,54.32,5.556));
#51669=CARTESIAN_POINT('',(-25.2277558616929,57.495,7.3035));
#51670=CARTESIAN_POINT('',(-25.8637938460731,57.495,5.556));
#51671=CARTESIAN_POINT('',(-25.2277558616929,54.32,7.3035));
#51672=CARTESIAN_POINT('Origin',(-24.6450275140451,54.32,7.3035));
#51673=CARTESIAN_POINT('',(-24.6450275140451,54.32,7.3035));
#51674=CARTESIAN_POINT('',(-25.2277558616929,54.32,7.3035));
#51675=CARTESIAN_POINT('',(-24.6450275140451,57.495,7.3035));
#51676=CARTESIAN_POINT('',(-25.2277558616929,57.495,7.3035));
#51677=CARTESIAN_POINT('',(-24.6450275140451,54.32,7.3035));
#51678=CARTESIAN_POINT('Origin',(-24.0089895296649,54.32,5.556));
#51679=CARTESIAN_POINT('',(-24.0089895296649,54.32,5.556));
#51680=CARTESIAN_POINT('',(-24.6450275140451,54.32,7.3035));
#51681=CARTESIAN_POINT('',(-24.0089895296649,57.495,5.556));
#51682=CARTESIAN_POINT('',(-24.6450275140451,57.495,7.3035));
#51683=CARTESIAN_POINT('',(-24.0089895296649,54.32,5.556));
#51684=CARTESIAN_POINT('Origin',(-23.3701546772862,54.32,5.556));
#51685=CARTESIAN_POINT('',(-23.3701546772862,54.32,5.556));
#51686=CARTESIAN_POINT('',(-24.0089895296649,54.32,5.556));
#51687=CARTESIAN_POINT('',(-23.3701546772862,57.495,5.556));
#51688=CARTESIAN_POINT('',(-24.0089895296649,57.495,5.556));
#51689=CARTESIAN_POINT('',(-23.3701546772862,54.32,5.556));
#51690=CARTESIAN_POINT('Origin',(-22.734116692906,54.32,7.3035));
#51691=CARTESIAN_POINT('',(-22.734116692906,54.32,7.3035));
#51692=CARTESIAN_POINT('',(-23.3701546772862,54.32,5.556));
#51693=CARTESIAN_POINT('',(-22.734116692906,57.495,7.3035));
#51694=CARTESIAN_POINT('',(-23.3701546772862,57.495,5.556));
#51695=CARTESIAN_POINT('',(-22.734116692906,54.32,7.3035));
#51696=CARTESIAN_POINT('Origin',(-22.1513883452582,54.32,7.3035));
#51697=CARTESIAN_POINT('',(-22.1513883452582,54.32,7.3035));
#51698=CARTESIAN_POINT('',(-22.734116692906,54.32,7.3035));
#51699=CARTESIAN_POINT('',(-22.1513883452582,57.495,7.3035));
#51700=CARTESIAN_POINT('',(-22.734116692906,57.495,7.3035));
#51701=CARTESIAN_POINT('',(-22.1513883452582,54.32,7.3035));
#51702=CARTESIAN_POINT('Origin',(-21.515350360878,54.32,5.556));
#51703=CARTESIAN_POINT('',(-21.515350360878,54.32,5.556));
#51704=CARTESIAN_POINT('',(-22.1513883452582,54.32,7.3035));
#51705=CARTESIAN_POINT('',(-21.515350360878,57.495,5.556));
#51706=CARTESIAN_POINT('',(-22.1513883452582,57.495,7.3035));
#51707=CARTESIAN_POINT('',(-21.515350360878,54.32,5.556));
#51708=CARTESIAN_POINT('Origin',(-20.8765155084993,54.32,5.556));
#51709=CARTESIAN_POINT('',(-20.8765155084993,54.32,5.556));
#51710=CARTESIAN_POINT('',(-21.515350360878,54.32,5.556));
#51711=CARTESIAN_POINT('',(-20.8765155084993,57.495,5.556));
#51712=CARTESIAN_POINT('',(-21.515350360878,57.495,5.556));
#51713=CARTESIAN_POINT('',(-20.8765155084993,54.32,5.556));
#51714=CARTESIAN_POINT('Origin',(-20.2404775241191,54.32,7.3035));
#51715=CARTESIAN_POINT('',(-20.2404775241191,54.32,7.3035));
#51716=CARTESIAN_POINT('',(-20.8765155084993,54.32,5.556));
#51717=CARTESIAN_POINT('',(-20.2404775241191,57.495,7.3035));
#51718=CARTESIAN_POINT('',(-20.8765155084993,57.495,5.556));
#51719=CARTESIAN_POINT('',(-20.2404775241191,54.32,7.3035));
#51720=CARTESIAN_POINT('Origin',(-19.6577491764713,54.32,7.3035));
#51721=CARTESIAN_POINT('',(-19.6577491764713,54.32,7.3035));
#51722=CARTESIAN_POINT('',(-20.2404775241191,54.32,7.3035));
#51723=CARTESIAN_POINT('',(-19.6577491764713,57.495,7.3035));
#51724=CARTESIAN_POINT('',(-20.2404775241191,57.495,7.3035));
#51725=CARTESIAN_POINT('',(-19.6577491764713,54.32,7.3035));
#51726=CARTESIAN_POINT('Origin',(-19.0217111920911,54.32,5.556));
#51727=CARTESIAN_POINT('',(-19.0217111920911,54.32,5.556));
#51728=CARTESIAN_POINT('',(-19.6577491764713,54.32,7.3035));
#51729=CARTESIAN_POINT('',(-19.0217111920911,57.495,5.556));
#51730=CARTESIAN_POINT('',(-19.6577491764713,57.495,7.3035));
#51731=CARTESIAN_POINT('',(-19.0217111920911,54.32,5.556));
#51732=CARTESIAN_POINT('Origin',(-18.3828763397124,54.32,5.556));
#51733=CARTESIAN_POINT('',(-18.3828763397124,54.32,5.556));
#51734=CARTESIAN_POINT('',(-19.0217111920911,54.32,5.556));
#51735=CARTESIAN_POINT('',(-18.3828763397124,57.495,5.556));
#51736=CARTESIAN_POINT('',(-19.0217111920911,57.495,5.556));
#51737=CARTESIAN_POINT('',(-18.3828763397124,54.32,5.556));
#51738=CARTESIAN_POINT('Origin',(-17.7468383553322,54.32,7.3035));
#51739=CARTESIAN_POINT('',(-17.7468383553322,54.32,7.3035));
#51740=CARTESIAN_POINT('',(-18.3828763397124,54.32,5.556));
#51741=CARTESIAN_POINT('',(-17.7468383553322,57.495,7.3035));
#51742=CARTESIAN_POINT('',(-18.3828763397124,57.495,5.556));
#51743=CARTESIAN_POINT('',(-17.7468383553322,54.32,7.3035));
#51744=CARTESIAN_POINT('Origin',(-17.1641100076844,54.32,7.3035));
#51745=CARTESIAN_POINT('',(-17.1641100076844,54.32,7.3035));
#51746=CARTESIAN_POINT('',(-17.7468383553322,54.32,7.3035));
#51747=CARTESIAN_POINT('',(-17.1641100076844,57.495,7.3035));
#51748=CARTESIAN_POINT('',(-17.7468383553322,57.495,7.3035));
#51749=CARTESIAN_POINT('',(-17.1641100076844,54.32,7.3035));
#51750=CARTESIAN_POINT('Origin',(-16.5280720233042,54.32,5.556));
#51751=CARTESIAN_POINT('',(-16.5280720233042,54.32,5.556));
#51752=CARTESIAN_POINT('',(-17.1641100076844,54.32,7.3035));
#51753=CARTESIAN_POINT('',(-16.5280720233042,57.495,5.556));
#51754=CARTESIAN_POINT('',(-17.1641100076844,57.495,7.3035));
#51755=CARTESIAN_POINT('',(-16.5280720233042,54.32,5.556));
#51756=CARTESIAN_POINT('Origin',(-15.8892371709255,54.32,5.556));
#51757=CARTESIAN_POINT('',(-15.8892371709255,54.32,5.556));
#51758=CARTESIAN_POINT('',(-16.5280720233042,54.32,5.556));
#51759=CARTESIAN_POINT('',(-15.8892371709255,57.495,5.556));
#51760=CARTESIAN_POINT('',(-16.5280720233042,57.495,5.556));
#51761=CARTESIAN_POINT('',(-15.8892371709255,54.32,5.556));
#51762=CARTESIAN_POINT('Origin',(-15.2531991865453,54.32,7.3035));
#51763=CARTESIAN_POINT('',(-15.2531991865453,54.32,7.3035));
#51764=CARTESIAN_POINT('',(-15.8892371709255,54.32,5.556));
#51765=CARTESIAN_POINT('',(-15.2531991865453,57.495,7.3035));
#51766=CARTESIAN_POINT('',(-15.8892371709255,57.495,5.556));
#51767=CARTESIAN_POINT('',(-15.2531991865453,54.32,7.3035));
#51768=CARTESIAN_POINT('Origin',(-14.6704708388975,54.32,7.3035));
#51769=CARTESIAN_POINT('',(-14.6704708388975,54.32,7.3035));
#51770=CARTESIAN_POINT('',(-15.2531991865453,54.32,7.3035));
#51771=CARTESIAN_POINT('',(-14.6704708388975,57.495,7.3035));
#51772=CARTESIAN_POINT('',(-15.2531991865453,57.495,7.3035));
#51773=CARTESIAN_POINT('',(-14.6704708388975,54.32,7.3035));
#51774=CARTESIAN_POINT('Origin',(-14.0344328545173,54.32,5.556));
#51775=CARTESIAN_POINT('',(-14.0344328545173,54.32,5.556));
#51776=CARTESIAN_POINT('',(-14.6704708388975,54.32,7.3035));
#51777=CARTESIAN_POINT('',(-14.0344328545173,57.495,5.556));
#51778=CARTESIAN_POINT('',(-14.6704708388975,57.495,7.3035));
#51779=CARTESIAN_POINT('',(-14.0344328545173,54.32,5.556));
#51780=CARTESIAN_POINT('Origin',(-13.3955980021386,54.32,5.556));
#51781=CARTESIAN_POINT('',(-13.3955980021386,54.32,5.556));
#51782=CARTESIAN_POINT('',(-14.0344328545173,54.32,5.556));
#51783=CARTESIAN_POINT('',(-13.3955980021386,57.495,5.556));
#51784=CARTESIAN_POINT('',(-14.0344328545173,57.495,5.556));
#51785=CARTESIAN_POINT('',(-13.3955980021386,54.32,5.556));
#51786=CARTESIAN_POINT('Origin',(-12.7595600177584,54.32,7.3035));
#51787=CARTESIAN_POINT('',(-12.7595600177584,54.32,7.3035));
#51788=CARTESIAN_POINT('',(-13.3955980021386,54.32,5.556));
#51789=CARTESIAN_POINT('',(-12.7595600177584,57.495,7.3035));
#51790=CARTESIAN_POINT('',(-13.3955980021386,57.495,5.556));
#51791=CARTESIAN_POINT('',(-12.7595600177584,54.32,7.3035));
#51792=CARTESIAN_POINT('Origin',(-12.1768316701106,54.32,7.3035));
#51793=CARTESIAN_POINT('',(-12.1768316701106,54.32,7.3035));
#51794=CARTESIAN_POINT('',(-12.7595600177584,54.32,7.3035));
#51795=CARTESIAN_POINT('',(-12.1768316701106,57.495,7.3035));
#51796=CARTESIAN_POINT('',(-12.7595600177584,57.495,7.3035));
#51797=CARTESIAN_POINT('',(-12.1768316701106,54.32,7.3035));
#51798=CARTESIAN_POINT('Origin',(-11.5407936857304,54.32,5.556));
#51799=CARTESIAN_POINT('',(-11.5407936857304,54.32,5.556));
#51800=CARTESIAN_POINT('',(-12.1768316701106,54.32,7.3035));
#51801=CARTESIAN_POINT('',(-11.5407936857304,57.495,5.556));
#51802=CARTESIAN_POINT('',(-12.1768316701106,57.495,7.3035));
#51803=CARTESIAN_POINT('',(-11.5407936857304,54.32,5.556));
#51804=CARTESIAN_POINT('Origin',(-10.9019588333517,54.32,5.556));
#51805=CARTESIAN_POINT('',(-10.9019588333517,54.32,5.556));
#51806=CARTESIAN_POINT('',(-11.5407936857304,54.32,5.556));
#51807=CARTESIAN_POINT('',(-10.9019588333517,57.495,5.556));
#51808=CARTESIAN_POINT('',(-11.5407936857304,57.495,5.556));
#51809=CARTESIAN_POINT('',(-10.9019588333517,54.32,5.556));
#51810=CARTESIAN_POINT('Origin',(-10.2659208489715,54.32,7.3035));
#51811=CARTESIAN_POINT('',(-10.2659208489715,54.32,7.3035));
#51812=CARTESIAN_POINT('',(-10.9019588333517,54.32,5.556));
#51813=CARTESIAN_POINT('',(-10.2659208489715,57.495,7.3035));
#51814=CARTESIAN_POINT('',(-10.9019588333517,57.495,5.556));
#51815=CARTESIAN_POINT('',(-10.2659208489715,54.32,7.3035));
#51816=CARTESIAN_POINT('Origin',(-9.68319250132369,54.32,7.3035));
#51817=CARTESIAN_POINT('',(-9.68319250132369,54.32,7.3035));
#51818=CARTESIAN_POINT('',(-10.2659208489715,54.32,7.3035));
#51819=CARTESIAN_POINT('',(-9.68319250132369,57.495,7.3035));
#51820=CARTESIAN_POINT('',(-10.2659208489715,57.495,7.3035));
#51821=CARTESIAN_POINT('',(-9.68319250132369,54.32,7.3035));
#51822=CARTESIAN_POINT('Origin',(-9.0471545169435,54.32,5.556));
#51823=CARTESIAN_POINT('',(-9.0471545169435,54.32,5.556));
#51824=CARTESIAN_POINT('',(-9.68319250132369,54.32,7.3035));
#51825=CARTESIAN_POINT('',(-9.0471545169435,57.495,5.556));
#51826=CARTESIAN_POINT('',(-9.68319250132369,57.495,7.3035));
#51827=CARTESIAN_POINT('',(-9.0471545169435,54.32,5.556));
#51828=CARTESIAN_POINT('Origin',(-8.40831966456478,54.32,5.556));
#51829=CARTESIAN_POINT('',(-8.40831966456478,54.32,5.556));
#51830=CARTESIAN_POINT('',(-9.0471545169435,54.32,5.556));
#51831=CARTESIAN_POINT('',(-8.40831966456478,57.495,5.556));
#51832=CARTESIAN_POINT('',(-9.0471545169435,57.495,5.556));
#51833=CARTESIAN_POINT('',(-8.40831966456478,54.32,5.556));
#51834=CARTESIAN_POINT('Origin',(-7.7722816801846,54.32,7.3035));
#51835=CARTESIAN_POINT('',(-7.7722816801846,54.32,7.3035));
#51836=CARTESIAN_POINT('',(-8.40831966456478,54.32,5.556));
#51837=CARTESIAN_POINT('',(-7.77228168018459,57.495,7.3035));
#51838=CARTESIAN_POINT('',(-8.40831966456478,57.495,5.556));
#51839=CARTESIAN_POINT('',(-7.7722816801846,54.32,7.3035));
#51840=CARTESIAN_POINT('Origin',(-7.18955333253679,54.32,7.3035));
#51841=CARTESIAN_POINT('',(-7.18955333253679,54.32,7.3035));
#51842=CARTESIAN_POINT('',(-7.7722816801846,54.32,7.3035));
#51843=CARTESIAN_POINT('',(-7.1895533325368,57.495,7.3035));
#51844=CARTESIAN_POINT('',(-7.7722816801846,57.495,7.3035));
#51845=CARTESIAN_POINT('',(-7.18955333253679,54.32,7.3035));
#51846=CARTESIAN_POINT('Origin',(-6.55351534815661,54.32,5.556));
#51847=CARTESIAN_POINT('',(-6.55351534815661,54.32,5.556));
#51848=CARTESIAN_POINT('',(-7.18955333253679,54.32,7.3035));
#51849=CARTESIAN_POINT('',(-6.5535153481566,57.495,5.556));
#51850=CARTESIAN_POINT('',(-7.18955333253679,57.495,7.3035));
#51851=CARTESIAN_POINT('',(-6.55351534815661,54.32,5.556));
#51852=CARTESIAN_POINT('Origin',(-5.91468049577789,54.32,5.556));
#51853=CARTESIAN_POINT('',(-5.91468049577789,54.32,5.556));
#51854=CARTESIAN_POINT('',(-6.55351534815661,54.32,5.556));
#51855=CARTESIAN_POINT('',(-5.91468049577788,57.495,5.556));
#51856=CARTESIAN_POINT('',(-6.55351534815661,57.495,5.556));
#51857=CARTESIAN_POINT('',(-5.91468049577789,54.32,5.556));
#51858=CARTESIAN_POINT('Origin',(-5.2786425113977,54.32,7.3035));
#51859=CARTESIAN_POINT('',(-5.2786425113977,54.32,7.3035));
#51860=CARTESIAN_POINT('',(-5.91468049577789,54.32,5.556));
#51861=CARTESIAN_POINT('',(-5.2786425113977,57.495,7.3035));
#51862=CARTESIAN_POINT('',(-5.91468049577789,57.495,5.556));
#51863=CARTESIAN_POINT('',(-5.2786425113977,54.32,7.3035));
#51864=CARTESIAN_POINT('Origin',(-4.6959141637499,54.32,7.3035));
#51865=CARTESIAN_POINT('',(-4.6959141637499,54.32,7.3035));
#51866=CARTESIAN_POINT('',(-5.2786425113977,54.32,7.3035));
#51867=CARTESIAN_POINT('',(-4.69591416374989,57.495,7.3035));
#51868=CARTESIAN_POINT('',(-5.2786425113977,57.495,7.3035));
#51869=CARTESIAN_POINT('',(-4.6959141637499,54.32,7.3035));
#51870=CARTESIAN_POINT('Origin',(-4.05987617936971,54.32,5.556));
#51871=CARTESIAN_POINT('',(-4.05987617936971,54.32,5.556));
#51872=CARTESIAN_POINT('',(-4.6959141637499,54.32,7.3035));
#51873=CARTESIAN_POINT('',(-4.05987617936971,57.495,5.556));
#51874=CARTESIAN_POINT('',(-4.6959141637499,57.495,7.3035));
#51875=CARTESIAN_POINT('',(-4.05987617936971,54.32,5.556));
#51876=CARTESIAN_POINT('Origin',(-3.42104132699099,54.32,5.556));
#51877=CARTESIAN_POINT('',(-3.42104132699099,54.32,5.556));
#51878=CARTESIAN_POINT('',(-4.05987617936971,54.32,5.556));
#51879=CARTESIAN_POINT('',(-3.42104132699099,57.495,5.556));
#51880=CARTESIAN_POINT('',(-4.05987617936971,57.495,5.556));
#51881=CARTESIAN_POINT('',(-3.42104132699099,54.32,5.556));
#51882=CARTESIAN_POINT('Origin',(-2.7850033426108,54.32,7.3035));
#51883=CARTESIAN_POINT('',(-2.7850033426108,54.32,7.3035));
#51884=CARTESIAN_POINT('',(-3.42104132699099,54.32,5.556));
#51885=CARTESIAN_POINT('',(-2.7850033426108,57.495,7.3035));
#51886=CARTESIAN_POINT('',(-3.42104132699099,57.495,5.556));
#51887=CARTESIAN_POINT('',(-2.7850033426108,54.32,7.3035));
#51888=CARTESIAN_POINT('Origin',(-2.202274994963,54.32,7.3035));
#51889=CARTESIAN_POINT('',(-2.202274994963,54.32,7.3035));
#51890=CARTESIAN_POINT('',(-2.7850033426108,54.32,7.3035));
#51891=CARTESIAN_POINT('',(-2.202274994963,57.495,7.3035));
#51892=CARTESIAN_POINT('',(-2.7850033426108,57.495,7.3035));
#51893=CARTESIAN_POINT('',(-2.202274994963,54.32,7.3035));
#51894=CARTESIAN_POINT('Origin',(-1.56623701058281,54.32,5.556));
#51895=CARTESIAN_POINT('',(-1.56623701058281,54.32,5.556));
#51896=CARTESIAN_POINT('',(-2.202274994963,54.32,7.3035));
#51897=CARTESIAN_POINT('',(-1.56623701058281,57.495,5.556));
#51898=CARTESIAN_POINT('',(-2.202274994963,57.495,7.3035));
#51899=CARTESIAN_POINT('',(-1.56623701058281,54.32,5.556));
#51900=CARTESIAN_POINT('Origin',(-0.927402158204089,54.32,5.556));
#51901=CARTESIAN_POINT('',(-0.927402158204089,54.32,5.556));
#51902=CARTESIAN_POINT('',(-1.56623701058281,54.32,5.556));
#51903=CARTESIAN_POINT('',(-0.927402158204096,57.495,5.556));
#51904=CARTESIAN_POINT('',(-1.56623701058281,57.495,5.556));
#51905=CARTESIAN_POINT('',(-0.927402158204089,54.32,5.556));
#51906=CARTESIAN_POINT('Origin',(-0.291364173823901,54.32,7.3035));
#51907=CARTESIAN_POINT('',(-0.291364173823901,54.32,7.3035));
#51908=CARTESIAN_POINT('',(-0.927402158204089,54.32,5.556));
#51909=CARTESIAN_POINT('',(-0.291364173823894,57.495,7.3035));
#51910=CARTESIAN_POINT('',(-0.927402158204089,57.495,5.556));
#51911=CARTESIAN_POINT('',(-0.291364173823901,54.32,7.3035));
#51912=CARTESIAN_POINT('Origin',(0.291364173823901,54.32,7.3035));
#51913=CARTESIAN_POINT('',(0.291364173823901,54.32,7.3035));
#51914=CARTESIAN_POINT('',(-0.291364173823901,54.32,7.3035));
#51915=CARTESIAN_POINT('',(0.291364173823894,57.495,7.3035));
#51916=CARTESIAN_POINT('',(-0.291364173823901,57.495,7.3035));
#51917=CARTESIAN_POINT('',(0.291364173823901,54.32,7.3035));
#51918=CARTESIAN_POINT('Origin',(0.927402158204089,54.32,5.556));
#51919=CARTESIAN_POINT('',(0.927402158204089,54.32,5.556));
#51920=CARTESIAN_POINT('',(0.291364173823901,54.32,7.3035));
#51921=CARTESIAN_POINT('',(0.927402158204096,57.495,5.556));
#51922=CARTESIAN_POINT('',(0.291364173823901,57.495,7.3035));
#51923=CARTESIAN_POINT('',(0.927402158204089,54.32,5.556));
#51924=CARTESIAN_POINT('Origin',(1.56623701058281,54.32,5.556));
#51925=CARTESIAN_POINT('',(1.56623701058281,54.32,5.556));
#51926=CARTESIAN_POINT('',(0.927402158204089,54.32,5.556));
#51927=CARTESIAN_POINT('',(1.56623701058281,57.495,5.556));
#51928=CARTESIAN_POINT('',(0.927402158204089,57.495,5.556));
#51929=CARTESIAN_POINT('',(1.56623701058281,54.32,5.556));
#51930=CARTESIAN_POINT('Origin',(2.202274994963,54.32,7.3035));
#51931=CARTESIAN_POINT('',(2.202274994963,54.32,7.3035));
#51932=CARTESIAN_POINT('',(1.56623701058281,54.32,5.556));
#51933=CARTESIAN_POINT('',(2.202274994963,57.495,7.3035));
#51934=CARTESIAN_POINT('',(1.56623701058281,57.495,5.556));
#51935=CARTESIAN_POINT('',(2.202274994963,54.32,7.3035));
#51936=CARTESIAN_POINT('Origin',(2.7850033426108,54.32,7.3035));
#51937=CARTESIAN_POINT('',(2.7850033426108,54.32,7.3035));
#51938=CARTESIAN_POINT('',(2.202274994963,54.32,7.3035));
#51939=CARTESIAN_POINT('',(2.7850033426108,57.495,7.3035));
#51940=CARTESIAN_POINT('',(2.202274994963,57.495,7.3035));
#51941=CARTESIAN_POINT('',(2.7850033426108,54.32,7.3035));
#51942=CARTESIAN_POINT('Origin',(3.42104132699099,54.32,5.556));
#51943=CARTESIAN_POINT('',(3.42104132699099,54.32,5.556));
#51944=CARTESIAN_POINT('',(2.7850033426108,54.32,7.3035));
#51945=CARTESIAN_POINT('',(3.42104132699099,57.495,5.556));
#51946=CARTESIAN_POINT('',(2.7850033426108,57.495,7.3035));
#51947=CARTESIAN_POINT('',(3.42104132699099,54.32,5.556));
#51948=CARTESIAN_POINT('Origin',(4.05987617936971,54.32,5.556));
#51949=CARTESIAN_POINT('',(4.05987617936971,54.32,5.556));
#51950=CARTESIAN_POINT('',(3.42104132699099,54.32,5.556));
#51951=CARTESIAN_POINT('',(4.05987617936971,57.495,5.556));
#51952=CARTESIAN_POINT('',(3.42104132699099,57.495,5.556));
#51953=CARTESIAN_POINT('',(4.05987617936971,54.32,5.556));
#51954=CARTESIAN_POINT('Origin',(4.6959141637499,54.32,7.3035));
#51955=CARTESIAN_POINT('',(4.6959141637499,54.32,7.3035));
#51956=CARTESIAN_POINT('',(4.05987617936971,54.32,5.556));
#51957=CARTESIAN_POINT('',(4.69591416374989,57.495,7.3035));
#51958=CARTESIAN_POINT('',(4.05987617936971,57.495,5.556));
#51959=CARTESIAN_POINT('',(4.6959141637499,54.32,7.3035));
#51960=CARTESIAN_POINT('Origin',(5.2786425113977,54.32,7.3035));
#51961=CARTESIAN_POINT('',(5.2786425113977,54.32,7.3035));
#51962=CARTESIAN_POINT('',(4.6959141637499,54.32,7.3035));
#51963=CARTESIAN_POINT('',(5.2786425113977,57.495,7.3035));
#51964=CARTESIAN_POINT('',(4.6959141637499,57.495,7.3035));
#51965=CARTESIAN_POINT('',(5.2786425113977,54.32,7.3035));
#51966=CARTESIAN_POINT('Origin',(5.91468049577789,54.32,5.556));
#51967=CARTESIAN_POINT('',(5.91468049577789,54.32,5.556));
#51968=CARTESIAN_POINT('',(5.2786425113977,54.32,7.3035));
#51969=CARTESIAN_POINT('',(5.91468049577788,57.495,5.556));
#51970=CARTESIAN_POINT('',(5.2786425113977,57.495,7.3035));
#51971=CARTESIAN_POINT('',(5.91468049577789,54.32,5.556));
#51972=CARTESIAN_POINT('Origin',(6.55351534815661,54.32,5.556));
#51973=CARTESIAN_POINT('',(6.55351534815661,54.32,5.556));
#51974=CARTESIAN_POINT('',(5.91468049577789,54.32,5.556));
#51975=CARTESIAN_POINT('',(6.5535153481566,57.495,5.556));
#51976=CARTESIAN_POINT('',(5.91468049577789,57.495,5.556));
#51977=CARTESIAN_POINT('',(6.55351534815661,54.32,5.556));
#51978=CARTESIAN_POINT('Origin',(7.18955333253679,54.32,7.3035));
#51979=CARTESIAN_POINT('',(7.18955333253679,54.32,7.3035));
#51980=CARTESIAN_POINT('',(6.55351534815661,54.32,5.556));
#51981=CARTESIAN_POINT('',(7.1895533325368,57.495,7.3035));
#51982=CARTESIAN_POINT('',(6.55351534815661,57.495,5.556));
#51983=CARTESIAN_POINT('',(7.18955333253679,54.32,7.3035));
#51984=CARTESIAN_POINT('Origin',(7.7722816801846,54.32,7.3035));
#51985=CARTESIAN_POINT('',(7.7722816801846,54.32,7.3035));
#51986=CARTESIAN_POINT('',(7.18955333253679,54.32,7.3035));
#51987=CARTESIAN_POINT('',(7.77228168018459,57.495,7.3035));
#51988=CARTESIAN_POINT('',(7.18955333253679,57.495,7.3035));
#51989=CARTESIAN_POINT('',(7.7722816801846,54.32,7.3035));
#51990=CARTESIAN_POINT('Origin',(8.40831966456478,54.32,5.556));
#51991=CARTESIAN_POINT('',(8.40831966456478,54.32,5.556));
#51992=CARTESIAN_POINT('',(7.7722816801846,54.32,7.3035));
#51993=CARTESIAN_POINT('',(8.40831966456479,57.495,5.556));
#51994=CARTESIAN_POINT('',(7.7722816801846,57.495,7.3035));
#51995=CARTESIAN_POINT('',(8.40831966456478,54.32,5.556));
#51996=CARTESIAN_POINT('Origin',(9.0471545169435,54.32,5.556));
#51997=CARTESIAN_POINT('',(9.0471545169435,54.32,5.556));
#51998=CARTESIAN_POINT('',(8.40831966456478,54.32,5.556));
#51999=CARTESIAN_POINT('',(9.04715451694351,57.495,5.556));
#52000=CARTESIAN_POINT('',(8.40831966456478,57.495,5.556));
#52001=CARTESIAN_POINT('',(9.0471545169435,54.32,5.556));
#52002=CARTESIAN_POINT('Origin',(9.68319250132369,54.32,7.3035));
#52003=CARTESIAN_POINT('',(9.68319250132369,54.32,7.3035));
#52004=CARTESIAN_POINT('',(9.0471545169435,54.32,5.556));
#52005=CARTESIAN_POINT('',(9.68319250132369,57.495,7.3035));
#52006=CARTESIAN_POINT('',(9.0471545169435,57.495,5.556));
#52007=CARTESIAN_POINT('',(9.68319250132369,54.32,7.3035));
#52008=CARTESIAN_POINT('Origin',(10.2659208489715,54.32,7.3035));
#52009=CARTESIAN_POINT('',(10.2659208489715,54.32,7.3035));
#52010=CARTESIAN_POINT('',(9.68319250132369,54.32,7.3035));
#52011=CARTESIAN_POINT('',(10.2659208489715,57.495,7.3035));
#52012=CARTESIAN_POINT('',(9.68319250132369,57.495,7.3035));
#52013=CARTESIAN_POINT('',(10.2659208489715,54.32,7.3035));
#52014=CARTESIAN_POINT('Origin',(10.9019588333517,54.32,5.556));
#52015=CARTESIAN_POINT('',(10.9019588333517,54.32,5.556));
#52016=CARTESIAN_POINT('',(10.2659208489715,54.32,7.3035));
#52017=CARTESIAN_POINT('',(10.9019588333517,57.495,5.556));
#52018=CARTESIAN_POINT('',(10.2659208489715,57.495,7.3035));
#52019=CARTESIAN_POINT('',(10.9019588333517,54.32,5.556));
#52020=CARTESIAN_POINT('Origin',(11.5407936857304,54.32,5.556));
#52021=CARTESIAN_POINT('',(11.5407936857304,54.32,5.556));
#52022=CARTESIAN_POINT('',(10.9019588333517,54.32,5.556));
#52023=CARTESIAN_POINT('',(11.5407936857304,57.495,5.556));
#52024=CARTESIAN_POINT('',(10.9019588333517,57.495,5.556));
#52025=CARTESIAN_POINT('',(11.5407936857304,54.32,5.556));
#52026=CARTESIAN_POINT('Origin',(12.1768316701106,54.32,7.3035));
#52027=CARTESIAN_POINT('',(12.1768316701106,54.32,7.3035));
#52028=CARTESIAN_POINT('',(11.5407936857304,54.32,5.556));
#52029=CARTESIAN_POINT('',(12.1768316701106,57.495,7.3035));
#52030=CARTESIAN_POINT('',(11.5407936857304,57.495,5.556));
#52031=CARTESIAN_POINT('',(12.1768316701106,54.32,7.3035));
#52032=CARTESIAN_POINT('Origin',(12.7595600177584,54.32,7.3035));
#52033=CARTESIAN_POINT('',(12.7595600177584,54.32,7.3035));
#52034=CARTESIAN_POINT('',(12.1768316701106,54.32,7.3035));
#52035=CARTESIAN_POINT('',(12.7595600177584,57.495,7.3035));
#52036=CARTESIAN_POINT('',(12.1768316701106,57.495,7.3035));
#52037=CARTESIAN_POINT('',(12.7595600177584,54.32,7.3035));
#52038=CARTESIAN_POINT('Origin',(13.3955980021386,54.32,5.556));
#52039=CARTESIAN_POINT('',(13.3955980021386,54.32,5.556));
#52040=CARTESIAN_POINT('',(12.7595600177584,54.32,7.3035));
#52041=CARTESIAN_POINT('',(13.3955980021386,57.495,5.556));
#52042=CARTESIAN_POINT('',(12.7595600177584,57.495,7.3035));
#52043=CARTESIAN_POINT('',(13.3955980021386,54.32,5.556));
#52044=CARTESIAN_POINT('Origin',(14.0344328545173,54.32,5.556));
#52045=CARTESIAN_POINT('',(14.0344328545173,54.32,5.556));
#52046=CARTESIAN_POINT('',(13.3955980021386,54.32,5.556));
#52047=CARTESIAN_POINT('',(14.0344328545173,57.495,5.556));
#52048=CARTESIAN_POINT('',(13.3955980021386,57.495,5.556));
#52049=CARTESIAN_POINT('',(14.0344328545173,54.32,5.556));
#52050=CARTESIAN_POINT('Origin',(14.6704708388975,54.32,7.3035));
#52051=CARTESIAN_POINT('',(14.6704708388975,54.32,7.3035));
#52052=CARTESIAN_POINT('',(14.0344328545173,54.32,5.556));
#52053=CARTESIAN_POINT('',(14.6704708388975,57.495,7.3035));
#52054=CARTESIAN_POINT('',(14.0344328545173,57.495,5.556));
#52055=CARTESIAN_POINT('',(14.6704708388975,54.32,7.3035));
#52056=CARTESIAN_POINT('Origin',(15.2531991865453,54.32,7.3035));
#52057=CARTESIAN_POINT('',(15.2531991865453,54.32,7.3035));
#52058=CARTESIAN_POINT('',(14.6704708388975,54.32,7.3035));
#52059=CARTESIAN_POINT('',(15.2531991865453,57.495,7.3035));
#52060=CARTESIAN_POINT('',(14.6704708388975,57.495,7.3035));
#52061=CARTESIAN_POINT('',(15.2531991865453,54.32,7.3035));
#52062=CARTESIAN_POINT('Origin',(15.8892371709255,54.32,5.556));
#52063=CARTESIAN_POINT('',(15.8892371709255,54.32,5.556));
#52064=CARTESIAN_POINT('',(15.2531991865453,54.32,7.3035));
#52065=CARTESIAN_POINT('',(15.8892371709255,57.495,5.556));
#52066=CARTESIAN_POINT('',(15.2531991865453,57.495,7.3035));
#52067=CARTESIAN_POINT('',(15.8892371709255,54.32,5.556));
#52068=CARTESIAN_POINT('Origin',(16.5280720233042,54.32,5.556));
#52069=CARTESIAN_POINT('',(16.5280720233042,54.32,5.556));
#52070=CARTESIAN_POINT('',(15.8892371709255,54.32,5.556));
#52071=CARTESIAN_POINT('',(16.5280720233042,57.495,5.556));
#52072=CARTESIAN_POINT('',(15.8892371709255,57.495,5.556));
#52073=CARTESIAN_POINT('',(16.5280720233042,54.32,5.556));
#52074=CARTESIAN_POINT('Origin',(17.1641100076844,54.32,7.3035));
#52075=CARTESIAN_POINT('',(17.1641100076844,54.32,7.3035));
#52076=CARTESIAN_POINT('',(16.5280720233042,54.32,5.556));
#52077=CARTESIAN_POINT('',(17.1641100076844,57.495,7.3035));
#52078=CARTESIAN_POINT('',(16.5280720233042,57.495,5.556));
#52079=CARTESIAN_POINT('',(17.1641100076844,54.32,7.3035));
#52080=CARTESIAN_POINT('Origin',(17.7468383553322,54.32,7.3035));
#52081=CARTESIAN_POINT('',(17.7468383553322,54.32,7.3035));
#52082=CARTESIAN_POINT('',(17.1641100076844,54.32,7.3035));
#52083=CARTESIAN_POINT('',(17.7468383553322,57.495,7.3035));
#52084=CARTESIAN_POINT('',(17.1641100076844,57.495,7.3035));
#52085=CARTESIAN_POINT('',(17.7468383553322,54.32,7.3035));
#52086=CARTESIAN_POINT('Origin',(18.3828763397124,54.32,5.556));
#52087=CARTESIAN_POINT('',(18.3828763397124,54.32,5.556));
#52088=CARTESIAN_POINT('',(17.7468383553322,54.32,7.3035));
#52089=CARTESIAN_POINT('',(18.3828763397124,57.495,5.556));
#52090=CARTESIAN_POINT('',(17.7468383553322,57.495,7.3035));
#52091=CARTESIAN_POINT('',(18.3828763397124,54.32,5.556));
#52092=CARTESIAN_POINT('Origin',(19.0217111920911,54.32,5.556));
#52093=CARTESIAN_POINT('',(19.0217111920911,54.32,5.556));
#52094=CARTESIAN_POINT('',(18.3828763397124,54.32,5.556));
#52095=CARTESIAN_POINT('',(19.0217111920911,57.495,5.556));
#52096=CARTESIAN_POINT('',(18.3828763397124,57.495,5.556));
#52097=CARTESIAN_POINT('',(19.0217111920911,54.32,5.556));
#52098=CARTESIAN_POINT('Origin',(19.6577491764713,54.32,7.3035));
#52099=CARTESIAN_POINT('',(19.6577491764713,54.32,7.3035));
#52100=CARTESIAN_POINT('',(19.0217111920911,54.32,5.556));
#52101=CARTESIAN_POINT('',(19.6577491764713,57.495,7.3035));
#52102=CARTESIAN_POINT('',(19.0217111920911,57.495,5.556));
#52103=CARTESIAN_POINT('',(19.6577491764713,54.32,7.3035));
#52104=CARTESIAN_POINT('Origin',(20.2404775241191,54.32,7.3035));
#52105=CARTESIAN_POINT('',(20.2404775241191,54.32,7.3035));
#52106=CARTESIAN_POINT('',(19.6577491764713,54.32,7.3035));
#52107=CARTESIAN_POINT('',(20.2404775241191,57.495,7.3035));
#52108=CARTESIAN_POINT('',(19.6577491764713,57.495,7.3035));
#52109=CARTESIAN_POINT('',(20.2404775241191,54.32,7.3035));
#52110=CARTESIAN_POINT('Origin',(20.8765155084993,54.32,5.556));
#52111=CARTESIAN_POINT('',(20.8765155084993,54.32,5.556));
#52112=CARTESIAN_POINT('',(20.2404775241191,54.32,7.3035));
#52113=CARTESIAN_POINT('',(20.8765155084993,57.495,5.556));
#52114=CARTESIAN_POINT('',(20.2404775241191,57.495,7.3035));
#52115=CARTESIAN_POINT('',(20.8765155084993,54.32,5.556));
#52116=CARTESIAN_POINT('Origin',(21.515350360878,54.32,5.556));
#52117=CARTESIAN_POINT('',(21.515350360878,54.32,5.556));
#52118=CARTESIAN_POINT('',(20.8765155084993,54.32,5.556));
#52119=CARTESIAN_POINT('',(21.515350360878,57.495,5.556));
#52120=CARTESIAN_POINT('',(20.8765155084993,57.495,5.556));
#52121=CARTESIAN_POINT('',(21.515350360878,54.32,5.556));
#52122=CARTESIAN_POINT('Origin',(22.1513883452582,54.32,7.3035));
#52123=CARTESIAN_POINT('',(22.1513883452582,54.32,7.3035));
#52124=CARTESIAN_POINT('',(21.515350360878,54.32,5.556));
#52125=CARTESIAN_POINT('',(22.1513883452582,57.495,7.3035));
#52126=CARTESIAN_POINT('',(21.515350360878,57.495,5.556));
#52127=CARTESIAN_POINT('',(22.1513883452582,54.32,7.3035));
#52128=CARTESIAN_POINT('Origin',(22.734116692906,54.32,7.3035));
#52129=CARTESIAN_POINT('',(22.734116692906,54.32,7.3035));
#52130=CARTESIAN_POINT('',(22.1513883452582,54.32,7.3035));
#52131=CARTESIAN_POINT('',(22.734116692906,57.495,7.3035));
#52132=CARTESIAN_POINT('',(22.1513883452582,57.495,7.3035));
#52133=CARTESIAN_POINT('',(22.734116692906,54.32,7.3035));
#52134=CARTESIAN_POINT('Origin',(23.3701546772862,54.32,5.556));
#52135=CARTESIAN_POINT('',(23.3701546772862,54.32,5.556));
#52136=CARTESIAN_POINT('',(22.734116692906,54.32,7.3035));
#52137=CARTESIAN_POINT('',(23.3701546772862,57.495,5.556));
#52138=CARTESIAN_POINT('',(22.734116692906,57.495,7.3035));
#52139=CARTESIAN_POINT('',(23.3701546772862,54.32,5.556));
#52140=CARTESIAN_POINT('Origin',(24.0089895296649,54.32,5.556));
#52141=CARTESIAN_POINT('',(24.0089895296649,54.32,5.556));
#52142=CARTESIAN_POINT('',(23.3701546772862,54.32,5.556));
#52143=CARTESIAN_POINT('',(24.0089895296649,57.495,5.556));
#52144=CARTESIAN_POINT('',(23.3701546772862,57.495,5.556));
#52145=CARTESIAN_POINT('',(24.0089895296649,54.32,5.556));
#52146=CARTESIAN_POINT('Origin',(24.6450275140451,54.32,7.3035));
#52147=CARTESIAN_POINT('',(24.6450275140451,54.32,7.3035));
#52148=CARTESIAN_POINT('',(24.0089895296649,54.32,5.556));
#52149=CARTESIAN_POINT('',(24.6450275140451,57.495,7.3035));
#52150=CARTESIAN_POINT('',(24.0089895296649,57.495,5.556));
#52151=CARTESIAN_POINT('',(24.6450275140451,54.32,7.3035));
#52152=CARTESIAN_POINT('Origin',(25.2277558616929,54.32,7.3035));
#52153=CARTESIAN_POINT('',(25.2277558616929,54.32,7.3035));
#52154=CARTESIAN_POINT('',(24.6450275140451,54.32,7.3035));
#52155=CARTESIAN_POINT('',(25.2277558616929,57.495,7.3035));
#52156=CARTESIAN_POINT('',(24.6450275140451,57.495,7.3035));
#52157=CARTESIAN_POINT('',(25.2277558616929,54.32,7.3035));
#52158=CARTESIAN_POINT('Origin',(25.8637938460731,54.32,5.556));
#52159=CARTESIAN_POINT('',(25.8637938460731,54.32,5.556));
#52160=CARTESIAN_POINT('',(25.2277558616929,54.32,7.3035));
#52161=CARTESIAN_POINT('',(25.8637938460731,57.495,5.556));
#52162=CARTESIAN_POINT('',(25.2277558616929,57.495,7.3035));
#52163=CARTESIAN_POINT('',(25.8637938460731,54.32,5.556));
#52164=CARTESIAN_POINT('Origin',(26.5026286984518,54.32,5.556));
#52165=CARTESIAN_POINT('',(26.5026286984518,54.32,5.556));
#52166=CARTESIAN_POINT('',(25.8637938460731,54.32,5.556));
#52167=CARTESIAN_POINT('',(26.5026286984518,57.495,5.556));
#52168=CARTESIAN_POINT('',(25.8637938460731,57.495,5.556));
#52169=CARTESIAN_POINT('',(26.5026286984518,54.32,5.556));
#52170=CARTESIAN_POINT('Origin',(27.138666682832,54.32,7.3035));
#52171=CARTESIAN_POINT('',(27.138666682832,54.32,7.3035));
#52172=CARTESIAN_POINT('',(26.5026286984518,54.32,5.556));
#52173=CARTESIAN_POINT('',(27.138666682832,57.495,7.3035));
#52174=CARTESIAN_POINT('',(26.5026286984518,57.495,5.556));
#52175=CARTESIAN_POINT('',(27.138666682832,54.32,7.3035));
#52176=CARTESIAN_POINT('Origin',(27.7213950304798,54.32,7.3035));
#52177=CARTESIAN_POINT('',(27.7213950304798,54.32,7.3035));
#52178=CARTESIAN_POINT('',(27.138666682832,54.32,7.3035));
#52179=CARTESIAN_POINT('',(27.7213950304798,57.495,7.3035));
#52180=CARTESIAN_POINT('',(27.138666682832,57.495,7.3035));
#52181=CARTESIAN_POINT('',(27.7213950304798,54.32,7.3035));
#52182=CARTESIAN_POINT('Origin',(28.35743301486,54.32,5.556));
#52183=CARTESIAN_POINT('',(28.35743301486,54.32,5.556));
#52184=CARTESIAN_POINT('',(27.7213950304798,54.32,7.3035));
#52185=CARTESIAN_POINT('',(28.35743301486,57.495,5.556));
#52186=CARTESIAN_POINT('',(27.7213950304798,57.495,7.3035));
#52187=CARTESIAN_POINT('',(28.35743301486,54.32,5.556));
#52188=CARTESIAN_POINT('Origin',(28.9962678672387,54.32,5.556));
#52189=CARTESIAN_POINT('',(28.9962678672387,54.32,5.556));
#52190=CARTESIAN_POINT('',(28.35743301486,54.32,5.556));
#52191=CARTESIAN_POINT('',(28.9962678672387,57.495,5.556));
#52192=CARTESIAN_POINT('',(28.35743301486,57.495,5.556));
#52193=CARTESIAN_POINT('',(28.9962678672387,54.32,5.556));
#52194=CARTESIAN_POINT('Origin',(29.6323058516189,54.32,7.3035));
#52195=CARTESIAN_POINT('',(29.6323058516189,54.32,7.3035));
#52196=CARTESIAN_POINT('',(28.9962678672387,54.32,5.556));
#52197=CARTESIAN_POINT('',(29.6323058516189,57.495,7.3035));
#52198=CARTESIAN_POINT('',(28.9962678672387,57.495,5.556));
#52199=CARTESIAN_POINT('',(29.6323058516189,54.32,7.3035));
#52200=CARTESIAN_POINT('Origin',(30.2150341992667,54.32,7.3035));
#52201=CARTESIAN_POINT('',(30.2150341992667,54.32,7.3035));
#52202=CARTESIAN_POINT('',(29.6323058516189,54.32,7.3035));
#52203=CARTESIAN_POINT('',(30.2150341992667,57.495,7.3035));
#52204=CARTESIAN_POINT('',(29.6323058516189,57.495,7.3035));
#52205=CARTESIAN_POINT('',(30.2150341992667,54.32,7.3035));
#52206=CARTESIAN_POINT('Origin',(30.8510721836469,54.32,5.556));
#52207=CARTESIAN_POINT('',(30.8510721836469,54.32,5.556));
#52208=CARTESIAN_POINT('',(30.2150341992667,54.32,7.3035));
#52209=CARTESIAN_POINT('',(30.8510721836469,57.495,5.556));
#52210=CARTESIAN_POINT('',(30.2150341992667,57.495,7.3035));
#52211=CARTESIAN_POINT('',(30.8510721836469,54.32,5.556));
#52212=CARTESIAN_POINT('Origin',(31.4899070360256,54.32,5.556));
#52213=CARTESIAN_POINT('',(31.4899070360256,54.32,5.556));
#52214=CARTESIAN_POINT('',(30.8510721836469,54.32,5.556));
#52215=CARTESIAN_POINT('',(31.4899070360256,57.495,5.556));
#52216=CARTESIAN_POINT('',(30.8510721836469,57.495,5.556));
#52217=CARTESIAN_POINT('',(31.4899070360256,54.32,5.556));
#52218=CARTESIAN_POINT('Origin',(32.1259450204058,54.32,7.3035));
#52219=CARTESIAN_POINT('',(32.1259450204058,54.32,7.3035));
#52220=CARTESIAN_POINT('',(31.4899070360256,54.32,5.556));
#52221=CARTESIAN_POINT('',(32.1259450204058,57.495,7.3035));
#52222=CARTESIAN_POINT('',(31.4899070360256,57.495,5.556));
#52223=CARTESIAN_POINT('',(32.1259450204058,54.32,7.3035));
#52224=CARTESIAN_POINT('Origin',(32.7086733680536,54.32,7.3035));
#52225=CARTESIAN_POINT('',(32.7086733680536,54.32,7.3035));
#52226=CARTESIAN_POINT('',(32.1259450204058,54.32,7.3035));
#52227=CARTESIAN_POINT('',(32.7086733680536,57.495,7.3035));
#52228=CARTESIAN_POINT('',(32.1259450204058,57.495,7.3035));
#52229=CARTESIAN_POINT('',(32.7086733680536,54.32,7.3035));
#52230=CARTESIAN_POINT('Origin',(33.3447113524338,54.32,5.556));
#52231=CARTESIAN_POINT('',(33.3447113524338,54.32,5.556));
#52232=CARTESIAN_POINT('',(32.7086733680536,54.32,7.3035));
#52233=CARTESIAN_POINT('',(33.3447113524338,57.495,5.556));
#52234=CARTESIAN_POINT('',(32.7086733680536,57.495,7.3035));
#52235=CARTESIAN_POINT('',(33.3447113524338,54.32,5.556));
#52236=CARTESIAN_POINT('Origin',(33.9835462048125,54.32,5.556));
#52237=CARTESIAN_POINT('',(33.9835462048125,54.32,5.556));
#52238=CARTESIAN_POINT('',(33.3447113524338,54.32,5.556));
#52239=CARTESIAN_POINT('',(33.9835462048125,57.495,5.556));
#52240=CARTESIAN_POINT('',(33.3447113524338,57.495,5.556));
#52241=CARTESIAN_POINT('',(33.9835462048125,54.32,5.556));
#52242=CARTESIAN_POINT('Origin',(34.6195841891927,54.32,7.3035));
#52243=CARTESIAN_POINT('',(34.6195841891927,54.32,7.3035));
#52244=CARTESIAN_POINT('',(33.9835462048125,54.32,5.556));
#52245=CARTESIAN_POINT('',(34.6195841891927,57.495,7.3035));
#52246=CARTESIAN_POINT('',(33.9835462048125,57.495,5.556));
#52247=CARTESIAN_POINT('',(34.6195841891927,54.32,7.3035));
#52248=CARTESIAN_POINT('Origin',(35.2023125368405,54.32,7.3035));
#52249=CARTESIAN_POINT('',(35.2023125368405,54.32,7.3035));
#52250=CARTESIAN_POINT('',(34.6195841891927,54.32,7.3035));
#52251=CARTESIAN_POINT('',(35.2023125368405,57.495,7.3035));
#52252=CARTESIAN_POINT('',(34.6195841891927,57.495,7.3035));
#52253=CARTESIAN_POINT('',(35.2023125368405,54.32,7.3035));
#52254=CARTESIAN_POINT('Origin',(35.8383505212207,54.32,5.556));
#52255=CARTESIAN_POINT('',(35.8383505212207,54.32,5.556));
#52256=CARTESIAN_POINT('',(35.2023125368405,54.32,7.3035));
#52257=CARTESIAN_POINT('',(35.8383505212207,57.495,5.556));
#52258=CARTESIAN_POINT('',(35.2023125368405,57.495,7.3035));
#52259=CARTESIAN_POINT('',(35.8383505212207,54.32,5.556));
#52260=CARTESIAN_POINT('Origin',(36.4771853735994,54.32,5.556));
#52261=CARTESIAN_POINT('',(36.4771853735994,54.32,5.556));
#52262=CARTESIAN_POINT('',(35.8383505212207,54.32,5.556));
#52263=CARTESIAN_POINT('',(36.4771853735994,57.495,5.556));
#52264=CARTESIAN_POINT('',(35.8383505212207,57.495,5.556));
#52265=CARTESIAN_POINT('',(36.4771853735994,54.32,5.556));
#52266=CARTESIAN_POINT('Origin',(37.1132233579796,54.32,7.3035));
#52267=CARTESIAN_POINT('',(37.1132233579796,54.32,7.3035));
#52268=CARTESIAN_POINT('',(36.4771853735994,54.32,5.556));
#52269=CARTESIAN_POINT('',(37.1132233579796,57.495,7.3035));
#52270=CARTESIAN_POINT('',(36.4771853735994,57.495,5.556));
#52271=CARTESIAN_POINT('',(37.1132233579796,54.32,7.3035));
#52272=CARTESIAN_POINT('Origin',(37.6959517056274,54.32,7.3035));
#52273=CARTESIAN_POINT('',(37.6959517056274,54.32,7.3035));
#52274=CARTESIAN_POINT('',(37.1132233579796,54.32,7.3035));
#52275=CARTESIAN_POINT('',(37.6959517056274,57.495,7.3035));
#52276=CARTESIAN_POINT('',(37.1132233579796,57.495,7.3035));
#52277=CARTESIAN_POINT('',(37.6959517056274,54.32,7.3035));
#52278=CARTESIAN_POINT('Origin',(38.3319896900076,54.32,5.556));
#52279=CARTESIAN_POINT('',(38.3319896900076,54.32,5.556));
#52280=CARTESIAN_POINT('',(37.6959517056274,54.32,7.3035));
#52281=CARTESIAN_POINT('',(38.3319896900076,57.495,5.556));
#52282=CARTESIAN_POINT('',(37.6959517056274,57.495,7.3035));
#52283=CARTESIAN_POINT('',(38.3319896900076,54.32,5.556));
#52284=CARTESIAN_POINT('Origin',(38.9708245423863,54.32,5.556));
#52285=CARTESIAN_POINT('',(38.9708245423863,54.32,5.556));
#52286=CARTESIAN_POINT('',(38.3319896900076,54.32,5.556));
#52287=CARTESIAN_POINT('',(38.9708245423863,57.495,5.556));
#52288=CARTESIAN_POINT('',(38.3319896900076,57.495,5.556));
#52289=CARTESIAN_POINT('',(38.9708245423863,54.32,5.556));
#52290=CARTESIAN_POINT('Origin',(39.6068625267665,54.32,7.3035));
#52291=CARTESIAN_POINT('',(39.6068625267665,54.32,7.3035));
#52292=CARTESIAN_POINT('',(38.9708245423863,54.32,5.556));
#52293=CARTESIAN_POINT('',(39.6068625267665,57.495,7.3035));
#52294=CARTESIAN_POINT('',(38.9708245423863,57.495,5.556));
#52295=CARTESIAN_POINT('',(39.6068625267665,54.32,7.3035));
#52296=CARTESIAN_POINT('Origin',(40.1895908744143,54.32,7.3035));
#52297=CARTESIAN_POINT('',(40.1895908744143,54.32,7.3035));
#52298=CARTESIAN_POINT('',(39.6068625267665,54.32,7.3035));
#52299=CARTESIAN_POINT('',(40.1895908744143,57.495,7.3035));
#52300=CARTESIAN_POINT('',(39.6068625267665,57.495,7.3035));
#52301=CARTESIAN_POINT('',(40.1895908744143,54.32,7.3035));
#52302=CARTESIAN_POINT('Origin',(40.8256288587945,54.32,5.556));
#52303=CARTESIAN_POINT('',(40.8256288587945,54.32,5.556));
#52304=CARTESIAN_POINT('',(40.1895908744143,54.32,7.3035));
#52305=CARTESIAN_POINT('',(40.8256288587945,57.495,5.556));
#52306=CARTESIAN_POINT('',(40.1895908744143,57.495,7.3035));
#52307=CARTESIAN_POINT('',(40.8256288587945,54.32,5.556));
#52308=CARTESIAN_POINT('Origin',(41.4644637111732,54.32,5.556));
#52309=CARTESIAN_POINT('',(41.4644637111732,54.32,5.556));
#52310=CARTESIAN_POINT('',(40.8256288587945,54.32,5.556));
#52311=CARTESIAN_POINT('',(41.4644637111732,57.495,5.556));
#52312=CARTESIAN_POINT('',(40.8256288587945,57.495,5.556));
#52313=CARTESIAN_POINT('',(41.4644637111732,54.32,5.556));
#52314=CARTESIAN_POINT('Origin',(42.1005016955534,54.32,7.3035));
#52315=CARTESIAN_POINT('',(42.1005016955534,54.32,7.3035));
#52316=CARTESIAN_POINT('',(41.4644637111732,54.32,5.556));
#52317=CARTESIAN_POINT('',(42.1005016955534,57.495,7.3035));
#52318=CARTESIAN_POINT('',(41.4644637111732,57.495,5.556));
#52319=CARTESIAN_POINT('',(42.1005016955534,54.32,7.3035));
#52320=CARTESIAN_POINT('Origin',(42.6832300432012,54.32,7.3035));
#52321=CARTESIAN_POINT('',(42.6832300432012,54.32,7.3035));
#52322=CARTESIAN_POINT('',(42.1005016955534,54.32,7.3035));
#52323=CARTESIAN_POINT('',(42.6832300432012,57.495,7.3035));
#52324=CARTESIAN_POINT('',(42.1005016955534,57.495,7.3035));
#52325=CARTESIAN_POINT('',(42.6832300432012,54.32,7.3035));
#52326=CARTESIAN_POINT('Origin',(43.3192680275814,54.32,5.556));
#52327=CARTESIAN_POINT('',(43.3192680275814,54.32,5.556));
#52328=CARTESIAN_POINT('',(42.6832300432012,54.32,7.3035));
#52329=CARTESIAN_POINT('',(43.3192680275813,57.495,5.556));
#52330=CARTESIAN_POINT('',(42.6832300432012,57.495,7.3035));
#52331=CARTESIAN_POINT('',(43.3192680275814,54.32,5.556));
#52332=CARTESIAN_POINT('Origin',(43.9581028799601,54.32,5.556));
#52333=CARTESIAN_POINT('',(43.9581028799601,54.32,5.556));
#52334=CARTESIAN_POINT('',(43.3192680275814,54.32,5.556));
#52335=CARTESIAN_POINT('',(43.9581028799601,57.495,5.556));
#52336=CARTESIAN_POINT('',(43.3192680275814,57.495,5.556));
#52337=CARTESIAN_POINT('',(43.9581028799601,54.32,5.556));
#52338=CARTESIAN_POINT('Origin',(44.5941408643403,54.32,7.3035));
#52339=CARTESIAN_POINT('',(44.5941408643403,54.32,7.3035));
#52340=CARTESIAN_POINT('',(43.9581028799601,54.32,5.556));
#52341=CARTESIAN_POINT('',(44.5941408643403,57.495,7.3035));
#52342=CARTESIAN_POINT('',(43.9581028799601,57.495,5.556));
#52343=CARTESIAN_POINT('',(44.5941408643403,54.32,7.3035));
#52344=CARTESIAN_POINT('Origin',(45.1768692119881,54.32,7.3035));
#52345=CARTESIAN_POINT('',(45.1768692119881,54.32,7.3035));
#52346=CARTESIAN_POINT('',(44.5941408643403,54.32,7.3035));
#52347=CARTESIAN_POINT('',(45.1768692119881,57.495,7.3035));
#52348=CARTESIAN_POINT('',(44.5941408643403,57.495,7.3035));
#52349=CARTESIAN_POINT('',(45.1768692119881,54.32,7.3035));
#52350=CARTESIAN_POINT('Origin',(45.8129071963683,54.32,5.556));
#52351=CARTESIAN_POINT('',(45.8129071963683,54.32,5.556));
#52352=CARTESIAN_POINT('',(45.1768692119881,54.32,7.3035));
#52353=CARTESIAN_POINT('',(45.8129071963683,57.495,5.556));
#52354=CARTESIAN_POINT('',(45.1768692119881,57.495,7.3035));
#52355=CARTESIAN_POINT('',(45.8129071963683,54.32,5.556));
#52356=CARTESIAN_POINT('Origin',(46.451742048747,54.32,5.556));
#52357=CARTESIAN_POINT('',(46.451742048747,54.32,5.556));
#52358=CARTESIAN_POINT('',(45.8129071963683,54.32,5.556));
#52359=CARTESIAN_POINT('',(46.451742048747,57.495,5.556));
#52360=CARTESIAN_POINT('',(45.8129071963683,57.495,5.556));
#52361=CARTESIAN_POINT('',(46.451742048747,54.32,5.556));
#52362=CARTESIAN_POINT('Origin',(47.0877800331272,54.32,7.3035));
#52363=CARTESIAN_POINT('',(47.0877800331272,54.32,7.3035));
#52364=CARTESIAN_POINT('',(46.451742048747,54.32,5.556));
#52365=CARTESIAN_POINT('',(47.0877800331272,57.495,7.3035));
#52366=CARTESIAN_POINT('',(46.451742048747,57.495,5.556));
#52367=CARTESIAN_POINT('',(47.0877800331272,54.32,7.3035));
#52368=CARTESIAN_POINT('Origin',(47.670508380775,54.32,7.3035));
#52369=CARTESIAN_POINT('',(47.670508380775,54.32,7.3035));
#52370=CARTESIAN_POINT('',(47.0877800331272,54.32,7.3035));
#52371=CARTESIAN_POINT('',(47.670508380775,57.495,7.3035));
#52372=CARTESIAN_POINT('',(47.0877800331272,57.495,7.3035));
#52373=CARTESIAN_POINT('',(47.670508380775,54.32,7.3035));
#52374=CARTESIAN_POINT('Origin',(48.3065463651552,54.32,5.556));
#52375=CARTESIAN_POINT('',(48.3065463651552,54.32,5.556));
#52376=CARTESIAN_POINT('',(47.670508380775,54.32,7.3035));
#52377=CARTESIAN_POINT('',(48.3065463651552,57.495,5.556));
#52378=CARTESIAN_POINT('',(47.670508380775,57.495,7.3035));
#52379=CARTESIAN_POINT('',(48.3065463651552,54.32,5.556));
#52380=CARTESIAN_POINT('Origin',(48.9453812175339,54.32,5.556));
#52381=CARTESIAN_POINT('',(48.9453812175339,54.32,5.556));
#52382=CARTESIAN_POINT('',(48.3065463651552,54.32,5.556));
#52383=CARTESIAN_POINT('',(48.9453812175339,57.495,5.556));
#52384=CARTESIAN_POINT('',(48.3065463651552,57.495,5.556));
#52385=CARTESIAN_POINT('',(48.9453812175339,54.32,5.556));
#52386=CARTESIAN_POINT('Origin',(49.5814192019141,54.32,7.3035));
#52387=CARTESIAN_POINT('',(49.5814192019141,54.32,7.3035));
#52388=CARTESIAN_POINT('',(48.9453812175339,54.32,5.556));
#52389=CARTESIAN_POINT('',(49.5814192019141,57.495,7.3035));
#52390=CARTESIAN_POINT('',(48.9453812175339,57.495,5.556));
#52391=CARTESIAN_POINT('',(49.5814192019141,54.32,7.3035));
#52392=CARTESIAN_POINT('Origin',(50.1641475495619,54.32,7.3035));
#52393=CARTESIAN_POINT('',(50.1641475495619,54.32,7.3035));
#52394=CARTESIAN_POINT('',(49.5814192019141,54.32,7.3035));
#52395=CARTESIAN_POINT('',(50.1641475495619,57.495,7.3035));
#52396=CARTESIAN_POINT('',(49.5814192019141,57.495,7.3035));
#52397=CARTESIAN_POINT('',(50.1641475495619,54.32,7.3035));
#52398=CARTESIAN_POINT('Origin',(50.800185533942,54.32,5.556));
#52399=CARTESIAN_POINT('',(50.800185533942,54.32,5.556));
#52400=CARTESIAN_POINT('',(50.1641475495619,54.32,7.3035));
#52401=CARTESIAN_POINT('',(50.8001855339421,57.495,5.556));
#52402=CARTESIAN_POINT('',(50.1641475495619,57.495,7.3035));
#52403=CARTESIAN_POINT('',(50.800185533942,54.32,5.556));
#52404=CARTESIAN_POINT('Origin',(51.4390203863208,54.32,5.556));
#52405=CARTESIAN_POINT('',(51.4390203863208,54.32,5.556));
#52406=CARTESIAN_POINT('',(50.800185533942,54.32,5.556));
#52407=CARTESIAN_POINT('',(51.4390203863208,57.495,5.556));
#52408=CARTESIAN_POINT('',(50.800185533942,57.495,5.556));
#52409=CARTESIAN_POINT('',(51.4390203863208,54.32,5.556));
#52410=CARTESIAN_POINT('Origin',(52.075058370701,54.32,7.3035));
#52411=CARTESIAN_POINT('',(52.075058370701,54.32,7.3035));
#52412=CARTESIAN_POINT('',(51.4390203863208,54.32,5.556));
#52413=CARTESIAN_POINT('',(52.075058370701,57.495,7.3035));
#52414=CARTESIAN_POINT('',(51.4390203863208,57.495,5.556));
#52415=CARTESIAN_POINT('',(52.075058370701,54.32,7.3035));
#52416=CARTESIAN_POINT('Origin',(52.6577867183488,54.32,7.3035));
#52417=CARTESIAN_POINT('',(52.6577867183488,54.32,7.3035));
#52418=CARTESIAN_POINT('',(52.075058370701,54.32,7.3035));
#52419=CARTESIAN_POINT('',(52.6577867183487,57.495,7.3035));
#52420=CARTESIAN_POINT('',(52.075058370701,57.495,7.3035));
#52421=CARTESIAN_POINT('',(52.6577867183488,54.32,7.3035));
#52422=CARTESIAN_POINT('Origin',(53.293824702729,54.32,5.556));
#52423=CARTESIAN_POINT('',(53.293824702729,54.32,5.556));
#52424=CARTESIAN_POINT('',(52.6577867183488,54.32,7.3035));
#52425=CARTESIAN_POINT('',(53.293824702729,57.495,5.556));
#52426=CARTESIAN_POINT('',(52.6577867183488,57.495,7.3035));
#52427=CARTESIAN_POINT('',(53.293824702729,54.32,5.556));
#52428=CARTESIAN_POINT('Origin',(53.9326595551077,54.32,5.556));
#52429=CARTESIAN_POINT('',(53.9326595551077,54.32,5.556));
#52430=CARTESIAN_POINT('',(53.293824702729,54.32,5.556));
#52431=CARTESIAN_POINT('',(53.9326595551077,57.495,5.556));
#52432=CARTESIAN_POINT('',(53.293824702729,57.495,5.556));
#52433=CARTESIAN_POINT('',(53.9326595551077,54.32,5.556));
#52434=CARTESIAN_POINT('Origin',(54.5686975394879,54.32,7.3035));
#52435=CARTESIAN_POINT('',(54.5686975394879,54.32,7.3035));
#52436=CARTESIAN_POINT('',(53.9326595551077,54.32,5.556));
#52437=CARTESIAN_POINT('',(54.5686975394879,57.495,7.3035));
#52438=CARTESIAN_POINT('',(53.9326595551077,57.495,5.556));
#52439=CARTESIAN_POINT('',(54.5686975394879,54.32,7.3035));
#52440=CARTESIAN_POINT('Origin',(55.1514258871357,54.32,7.3035));
#52441=CARTESIAN_POINT('',(55.1514258871357,54.32,7.3035));
#52442=CARTESIAN_POINT('',(54.5686975394879,54.32,7.3035));
#52443=CARTESIAN_POINT('',(55.1514258871357,57.495,7.3035));
#52444=CARTESIAN_POINT('',(54.5686975394879,57.495,7.3035));
#52445=CARTESIAN_POINT('',(55.1514258871357,54.32,7.3035));
#52446=CARTESIAN_POINT('Origin',(55.7874638715158,54.32,5.556));
#52447=CARTESIAN_POINT('',(55.7874638715158,54.32,5.556));
#52448=CARTESIAN_POINT('',(55.1514258871357,54.32,7.3035));
#52449=CARTESIAN_POINT('',(55.7874638715158,57.495,5.556));
#52450=CARTESIAN_POINT('',(55.1514258871357,57.495,7.3035));
#52451=CARTESIAN_POINT('',(55.7874638715158,54.32,5.556));
#52452=CARTESIAN_POINT('Origin',(56.4262987238946,54.32,5.556));
#52453=CARTESIAN_POINT('',(56.4262987238946,54.32,5.556));
#52454=CARTESIAN_POINT('',(55.7874638715158,54.32,5.556));
#52455=CARTESIAN_POINT('',(56.4262987238946,57.495,5.556));
#52456=CARTESIAN_POINT('',(55.7874638715158,57.495,5.556));
#52457=CARTESIAN_POINT('',(56.4262987238946,54.32,5.556));
#52458=CARTESIAN_POINT('Origin',(57.0623367082748,54.32,7.3035));
#52459=CARTESIAN_POINT('',(57.0623367082748,54.32,7.3035));
#52460=CARTESIAN_POINT('',(56.4262987238946,54.32,5.556));
#52461=CARTESIAN_POINT('',(57.0623367082747,57.495,7.3035));
#52462=CARTESIAN_POINT('',(56.4262987238946,57.495,5.556));
#52463=CARTESIAN_POINT('',(57.0623367082748,54.32,7.3035));
#52464=CARTESIAN_POINT('Origin',(57.6450650559226,54.32,7.3035));
#52465=CARTESIAN_POINT('',(57.6450650559226,54.32,7.3035));
#52466=CARTESIAN_POINT('',(57.0623367082748,54.32,7.3035));
#52467=CARTESIAN_POINT('',(57.6450650559226,57.495,7.3035));
#52468=CARTESIAN_POINT('',(57.0623367082748,57.495,7.3035));
#52469=CARTESIAN_POINT('',(57.6450650559226,54.32,7.3035));
#52470=CARTESIAN_POINT('Origin',(58.2811030403027,54.32,5.556));
#52471=CARTESIAN_POINT('',(58.2811030403027,54.32,5.556));
#52472=CARTESIAN_POINT('',(57.6450650559226,54.32,7.3035));
#52473=CARTESIAN_POINT('',(58.2811030403027,57.495,5.556));
#52474=CARTESIAN_POINT('',(57.6450650559226,57.495,7.3035));
#52475=CARTESIAN_POINT('',(58.2811030403027,54.32,5.556));
#52476=CARTESIAN_POINT('Origin',(58.9199378926815,54.32,5.556));
#52477=CARTESIAN_POINT('',(58.9199378926815,54.32,5.556));
#52478=CARTESIAN_POINT('',(58.2811030403027,54.32,5.556));
#52479=CARTESIAN_POINT('',(58.9199378926815,57.495,5.556));
#52480=CARTESIAN_POINT('',(58.2811030403027,57.495,5.556));
#52481=CARTESIAN_POINT('',(58.9199378926815,54.32,5.556));
#52482=CARTESIAN_POINT('Origin',(59.5559758770617,54.32,7.3035));
#52483=CARTESIAN_POINT('',(59.5559758770617,54.32,7.3035));
#52484=CARTESIAN_POINT('',(58.9199378926815,54.32,5.556));
#52485=CARTESIAN_POINT('',(59.5559758770617,57.495,7.3035));
#52486=CARTESIAN_POINT('',(58.9199378926815,57.495,5.556));
#52487=CARTESIAN_POINT('',(59.5559758770617,54.32,7.3035));
#52488=CARTESIAN_POINT('Origin',(60.1387042247095,54.32,7.3035));
#52489=CARTESIAN_POINT('',(60.1387042247095,54.32,7.3035));
#52490=CARTESIAN_POINT('',(59.5559758770617,54.32,7.3035));
#52491=CARTESIAN_POINT('',(60.1387042247095,57.495,7.3035));
#52492=CARTESIAN_POINT('',(59.5559758770617,57.495,7.3035));
#52493=CARTESIAN_POINT('',(60.1387042247095,54.32,7.3035));
#52494=CARTESIAN_POINT('Origin',(60.7747422090896,54.32,5.556));
#52495=CARTESIAN_POINT('',(60.7747422090896,54.32,5.556));
#52496=CARTESIAN_POINT('',(60.1387042247095,54.32,7.3035));
#52497=CARTESIAN_POINT('',(60.7747422090896,57.495,5.556));
#52498=CARTESIAN_POINT('',(60.1387042247095,57.495,7.3035));
#52499=CARTESIAN_POINT('',(60.7747422090896,54.32,5.556));
#52500=CARTESIAN_POINT('Origin',(61.4135770614684,54.32,5.556));
#52501=CARTESIAN_POINT('',(61.4135770614684,54.32,5.556));
#52502=CARTESIAN_POINT('',(60.7747422090896,54.32,5.556));
#52503=CARTESIAN_POINT('',(61.4135770614684,57.495,5.556));
#52504=CARTESIAN_POINT('',(60.7747422090896,57.495,5.556));
#52505=CARTESIAN_POINT('',(61.4135770614684,54.32,5.556));
#52506=CARTESIAN_POINT('Origin',(62.0496150458486,54.32,7.3035));
#52507=CARTESIAN_POINT('',(62.0496150458486,54.32,7.3035));
#52508=CARTESIAN_POINT('',(61.4135770614684,54.32,5.556));
#52509=CARTESIAN_POINT('',(62.0496150458486,57.495,7.3035));
#52510=CARTESIAN_POINT('',(61.4135770614684,57.495,5.556));
#52511=CARTESIAN_POINT('',(62.0496150458486,54.32,7.3035));
#52512=CARTESIAN_POINT('Origin',(62.6323433934964,54.32,7.3035));
#52513=CARTESIAN_POINT('',(62.6323433934964,54.32,7.3035));
#52514=CARTESIAN_POINT('',(62.0496150458486,54.32,7.3035));
#52515=CARTESIAN_POINT('',(62.6323433934964,57.495,7.3035));
#52516=CARTESIAN_POINT('',(62.0496150458486,57.495,7.3035));
#52517=CARTESIAN_POINT('',(62.6323433934964,54.32,7.3035));
#52518=CARTESIAN_POINT('Origin',(63.2683813778765,54.32,5.556));
#52519=CARTESIAN_POINT('',(63.2683813778765,54.32,5.556));
#52520=CARTESIAN_POINT('',(62.6323433934964,54.32,7.3035));
#52521=CARTESIAN_POINT('',(63.2683813778766,57.495,5.556));
#52522=CARTESIAN_POINT('',(62.6323433934964,57.495,7.3035));
#52523=CARTESIAN_POINT('',(63.2683813778765,54.32,5.556));
#52524=CARTESIAN_POINT('Origin',(63.9072162302553,54.32,5.556));
#52525=CARTESIAN_POINT('',(63.9072162302553,54.32,5.556));
#52526=CARTESIAN_POINT('',(63.2683813778765,54.32,5.556));
#52527=CARTESIAN_POINT('',(63.9072162302553,57.495,5.556));
#52528=CARTESIAN_POINT('',(63.2683813778765,57.495,5.556));
#52529=CARTESIAN_POINT('',(63.9072162302553,54.32,5.556));
#52530=CARTESIAN_POINT('Origin',(64.5432542146355,54.32,7.3035));
#52531=CARTESIAN_POINT('',(64.5432542146355,54.32,7.3035));
#52532=CARTESIAN_POINT('',(63.9072162302553,54.32,5.556));
#52533=CARTESIAN_POINT('',(64.5432542146355,57.495,7.3035));
#52534=CARTESIAN_POINT('',(63.9072162302553,57.495,5.556));
#52535=CARTESIAN_POINT('',(64.5432542146355,54.32,7.3035));
#52536=CARTESIAN_POINT('Origin',(65.1259825622833,54.32,7.3035));
#52537=CARTESIAN_POINT('',(65.1259825622833,54.32,7.3035));
#52538=CARTESIAN_POINT('',(64.5432542146355,54.32,7.3035));
#52539=CARTESIAN_POINT('',(65.1259825622832,57.495,7.3035));
#52540=CARTESIAN_POINT('',(64.5432542146355,57.495,7.3035));
#52541=CARTESIAN_POINT('',(65.1259825622833,54.32,7.3035));
#52542=CARTESIAN_POINT('Origin',(65.7620205466634,54.32,5.556));
#52543=CARTESIAN_POINT('',(65.7620205466634,54.32,5.556));
#52544=CARTESIAN_POINT('',(65.1259825622833,54.32,7.3035));
#52545=CARTESIAN_POINT('',(65.7620205466635,57.495,5.556));
#52546=CARTESIAN_POINT('',(65.1259825622833,57.495,7.3035));
#52547=CARTESIAN_POINT('',(65.7620205466634,54.32,5.556));
#52548=CARTESIAN_POINT('Origin',(66.4008553990422,54.32,5.556));
#52549=CARTESIAN_POINT('',(66.4008553990422,54.32,5.556));
#52550=CARTESIAN_POINT('',(65.7620205466634,54.32,5.556));
#52551=CARTESIAN_POINT('',(66.4008553990421,57.495,5.556));
#52552=CARTESIAN_POINT('',(65.7620205466634,57.495,5.556));
#52553=CARTESIAN_POINT('',(66.4008553990422,54.32,5.556));
#52554=CARTESIAN_POINT('Origin',(67.0368933834223,54.32,7.3035));
#52555=CARTESIAN_POINT('',(67.0368933834223,54.32,7.3035));
#52556=CARTESIAN_POINT('',(66.4008553990422,54.32,5.556));
#52557=CARTESIAN_POINT('',(67.0368933834224,57.495,7.3035));
#52558=CARTESIAN_POINT('',(66.4008553990422,57.495,5.556));
#52559=CARTESIAN_POINT('',(67.0368933834223,54.32,7.3035));
#52560=CARTESIAN_POINT('Origin',(67.6196217310702,54.32,7.3035));
#52561=CARTESIAN_POINT('',(67.6196217310702,54.32,7.3035));
#52562=CARTESIAN_POINT('',(67.0368933834223,54.32,7.3035));
#52563=CARTESIAN_POINT('',(67.6196217310702,57.495,7.3035));
#52564=CARTESIAN_POINT('',(67.0368933834223,57.495,7.3035));
#52565=CARTESIAN_POINT('',(67.6196217310702,54.32,7.3035));
#52566=CARTESIAN_POINT('Origin',(68.2556597154503,54.32,5.556));
#52567=CARTESIAN_POINT('',(68.2556597154503,54.32,5.556));
#52568=CARTESIAN_POINT('',(67.6196217310702,54.32,7.3035));
#52569=CARTESIAN_POINT('',(68.2556597154503,57.495,5.556));
#52570=CARTESIAN_POINT('',(67.6196217310702,57.495,7.3035));
#52571=CARTESIAN_POINT('',(68.2556597154503,54.32,5.556));
#52572=CARTESIAN_POINT('Origin',(68.8944945678291,54.32,5.556));
#52573=CARTESIAN_POINT('',(68.8944945678291,54.32,5.556));
#52574=CARTESIAN_POINT('',(68.2556597154503,54.32,5.556));
#52575=CARTESIAN_POINT('',(68.8944945678291,57.495,5.556));
#52576=CARTESIAN_POINT('',(68.2556597154503,57.495,5.556));
#52577=CARTESIAN_POINT('',(68.8944945678291,54.32,5.556));
#52578=CARTESIAN_POINT('Origin',(69.5305325522092,54.32,7.3035));
#52579=CARTESIAN_POINT('',(69.5305325522092,54.32,7.3035));
#52580=CARTESIAN_POINT('',(68.8944945678291,54.32,5.556));
#52581=CARTESIAN_POINT('',(69.5305325522092,57.495,7.3035));
#52582=CARTESIAN_POINT('',(68.8944945678291,57.495,5.556));
#52583=CARTESIAN_POINT('',(69.5305325522092,54.32,7.3035));
#52584=CARTESIAN_POINT('Origin',(70.1132608998571,54.32,7.3035));
#52585=CARTESIAN_POINT('',(70.1132608998571,54.32,7.3035));
#52586=CARTESIAN_POINT('',(69.5305325522092,54.32,7.3035));
#52587=CARTESIAN_POINT('',(70.1132608998571,57.495,7.3035));
#52588=CARTESIAN_POINT('',(69.5305325522092,57.495,7.3035));
#52589=CARTESIAN_POINT('',(70.1132608998571,54.32,7.3035));
#52590=CARTESIAN_POINT('Origin',(70.7492988842372,54.32,5.556));
#52591=CARTESIAN_POINT('',(70.7492988842372,54.32,5.556));
#52592=CARTESIAN_POINT('',(70.1132608998571,54.32,7.3035));
#52593=CARTESIAN_POINT('',(70.7492988842372,57.495,5.556));
#52594=CARTESIAN_POINT('',(70.1132608998571,57.495,7.3035));
#52595=CARTESIAN_POINT('',(70.7492988842372,54.32,5.556));
#52596=CARTESIAN_POINT('Origin',(71.388133736616,54.32,5.556));
#52597=CARTESIAN_POINT('',(71.388133736616,54.32,5.556));
#52598=CARTESIAN_POINT('',(70.7492988842372,54.32,5.556));
#52599=CARTESIAN_POINT('',(71.388133736616,57.495,5.556));
#52600=CARTESIAN_POINT('',(70.7492988842372,57.495,5.556));
#52601=CARTESIAN_POINT('',(71.388133736616,54.32,5.556));
#52602=CARTESIAN_POINT('Origin',(72.0241717209961,54.32,7.3035));
#52603=CARTESIAN_POINT('',(72.0241717209961,54.32,7.3035));
#52604=CARTESIAN_POINT('',(71.388133736616,54.32,5.556));
#52605=CARTESIAN_POINT('',(72.0241717209961,57.495,7.3035));
#52606=CARTESIAN_POINT('',(71.388133736616,57.495,5.556));
#52607=CARTESIAN_POINT('',(72.0241717209961,54.32,7.3035));
#52608=CARTESIAN_POINT('Origin',(72.606900068644,54.32,7.3035));
#52609=CARTESIAN_POINT('',(72.606900068644,54.32,7.3035));
#52610=CARTESIAN_POINT('',(72.0241717209961,54.32,7.3035));
#52611=CARTESIAN_POINT('',(72.606900068644,57.495,7.3035));
#52612=CARTESIAN_POINT('',(72.0241717209961,57.495,7.3035));
#52613=CARTESIAN_POINT('',(72.606900068644,54.32,7.3035));
#52614=CARTESIAN_POINT('Origin',(73.2429380530241,54.32,5.556));
#52615=CARTESIAN_POINT('',(73.2429380530241,54.32,5.556));
#52616=CARTESIAN_POINT('',(72.606900068644,54.32,7.3035));
#52617=CARTESIAN_POINT('',(73.2429380530241,57.495,5.556));
#52618=CARTESIAN_POINT('',(72.606900068644,57.495,7.3035));
#52619=CARTESIAN_POINT('',(73.2429380530241,54.32,5.556));
#52620=CARTESIAN_POINT('Origin',(73.8817729054029,54.32,5.556));
#52621=CARTESIAN_POINT('',(73.8817729054029,54.32,5.556));
#52622=CARTESIAN_POINT('',(73.2429380530241,54.32,5.556));
#52623=CARTESIAN_POINT('',(73.8817729054029,57.495,5.556));
#52624=CARTESIAN_POINT('',(73.2429380530241,57.495,5.556));
#52625=CARTESIAN_POINT('',(73.8817729054029,54.32,5.556));
#52626=CARTESIAN_POINT('Origin',(74.517810889783,54.32,7.3035));
#52627=CARTESIAN_POINT('',(74.517810889783,54.32,7.3035));
#52628=CARTESIAN_POINT('',(73.8817729054029,54.32,5.556));
#52629=CARTESIAN_POINT('',(74.517810889783,57.495,7.3035));
#52630=CARTESIAN_POINT('',(73.8817729054029,57.495,5.556));
#52631=CARTESIAN_POINT('',(74.517810889783,54.32,7.3035));
#52632=CARTESIAN_POINT('Origin',(75.1005392374309,54.32,7.3035));
#52633=CARTESIAN_POINT('',(75.1005392374309,54.32,7.3035));
#52634=CARTESIAN_POINT('',(74.517810889783,54.32,7.3035));
#52635=CARTESIAN_POINT('',(75.1005392374309,57.495,7.3035));
#52636=CARTESIAN_POINT('',(74.517810889783,57.495,7.3035));
#52637=CARTESIAN_POINT('',(75.1005392374309,54.32,7.3035));
#52638=CARTESIAN_POINT('Origin',(75.736577221811,54.32,5.556));
#52639=CARTESIAN_POINT('',(75.736577221811,54.32,5.556));
#52640=CARTESIAN_POINT('',(75.1005392374309,54.32,7.3035));
#52641=CARTESIAN_POINT('',(75.736577221811,57.495,5.556));
#52642=CARTESIAN_POINT('',(75.1005392374309,57.495,7.3035));
#52643=CARTESIAN_POINT('',(75.736577221811,54.32,5.556));
#52644=CARTESIAN_POINT('Origin',(76.3754120741898,54.32,5.556));
#52645=CARTESIAN_POINT('',(76.3754120741898,54.32,5.556));
#52646=CARTESIAN_POINT('',(75.736577221811,54.32,5.556));
#52647=CARTESIAN_POINT('',(76.3754120741898,57.495,5.556));
#52648=CARTESIAN_POINT('',(75.736577221811,57.495,5.556));
#52649=CARTESIAN_POINT('',(76.3754120741898,54.32,5.556));
#52650=CARTESIAN_POINT('Origin',(77.0114500585699,54.32,7.3035));
#52651=CARTESIAN_POINT('',(77.0114500585699,54.32,7.3035));
#52652=CARTESIAN_POINT('',(76.3754120741898,54.32,5.556));
#52653=CARTESIAN_POINT('',(77.0114500585699,57.495,7.3035));
#52654=CARTESIAN_POINT('',(76.3754120741898,57.495,5.556));
#52655=CARTESIAN_POINT('',(77.0114500585699,54.32,7.3035));
#52656=CARTESIAN_POINT('Origin',(77.5941784062178,54.32,7.3035));
#52657=CARTESIAN_POINT('',(77.5941784062178,54.32,7.3035));
#52658=CARTESIAN_POINT('',(77.0114500585699,54.32,7.3035));
#52659=CARTESIAN_POINT('',(77.5941784062177,57.495,7.3035));
#52660=CARTESIAN_POINT('',(77.0114500585699,57.495,7.3035));
#52661=CARTESIAN_POINT('',(77.5941784062178,54.32,7.3035));
#52662=CARTESIAN_POINT('Origin',(78.2302163905979,54.32,5.556));
#52663=CARTESIAN_POINT('',(78.2302163905979,54.32,5.556));
#52664=CARTESIAN_POINT('',(77.5941784062178,54.32,7.3035));
#52665=CARTESIAN_POINT('',(78.2302163905979,57.495,5.556));
#52666=CARTESIAN_POINT('',(77.5941784062178,57.495,7.3035));
#52667=CARTESIAN_POINT('',(78.2302163905979,54.32,5.556));
#52668=CARTESIAN_POINT('Origin',(78.8690512429767,54.32,5.556));
#52669=CARTESIAN_POINT('',(78.8690512429767,54.32,5.556));
#52670=CARTESIAN_POINT('',(78.2302163905979,54.32,5.556));
#52671=CARTESIAN_POINT('',(78.8690512429766,57.495,5.556));
#52672=CARTESIAN_POINT('',(78.2302163905979,57.495,5.556));
#52673=CARTESIAN_POINT('',(78.8690512429767,54.32,5.556));
#52674=CARTESIAN_POINT('Origin',(79.5050892273568,54.32,7.3035));
#52675=CARTESIAN_POINT('',(79.5050892273568,54.32,7.3035));
#52676=CARTESIAN_POINT('',(78.8690512429767,54.32,5.556));
#52677=CARTESIAN_POINT('',(79.5050892273568,57.495,7.3035));
#52678=CARTESIAN_POINT('',(78.8690512429767,57.495,5.556));
#52679=CARTESIAN_POINT('',(79.5050892273568,54.32,7.3035));
#52680=CARTESIAN_POINT('Origin',(80.0878175750046,54.32,7.3035));
#52681=CARTESIAN_POINT('',(80.0878175750046,54.32,7.3035));
#52682=CARTESIAN_POINT('',(79.5050892273568,54.32,7.3035));
#52683=CARTESIAN_POINT('',(80.0878175750046,57.495,7.3035));
#52684=CARTESIAN_POINT('',(79.5050892273568,57.495,7.3035));
#52685=CARTESIAN_POINT('',(80.0878175750046,54.32,7.3035));
#52686=CARTESIAN_POINT('Origin',(80.7238555593848,54.32,5.556));
#52687=CARTESIAN_POINT('',(80.7238555593848,54.32,5.556));
#52688=CARTESIAN_POINT('',(80.0878175750046,54.32,7.3035));
#52689=CARTESIAN_POINT('',(80.7238555593848,57.495,5.556));
#52690=CARTESIAN_POINT('',(80.0878175750046,57.495,7.3035));
#52691=CARTESIAN_POINT('',(80.7238555593848,54.32,5.556));
#52692=CARTESIAN_POINT('Origin',(81.3626904117636,54.32,5.556));
#52693=CARTESIAN_POINT('',(81.3626904117636,54.32,5.556));
#52694=CARTESIAN_POINT('',(80.7238555593848,54.32,5.556));
#52695=CARTESIAN_POINT('',(81.3626904117635,57.495,5.556));
#52696=CARTESIAN_POINT('',(80.7238555593848,57.495,5.556));
#52697=CARTESIAN_POINT('',(81.3626904117636,54.32,5.556));
#52698=CARTESIAN_POINT('Origin',(81.9987283961437,54.32,7.3035));
#52699=CARTESIAN_POINT('',(81.9987283961437,54.32,7.3035));
#52700=CARTESIAN_POINT('',(81.3626904117636,54.32,5.556));
#52701=CARTESIAN_POINT('',(81.9987283961437,57.495,7.3035));
#52702=CARTESIAN_POINT('',(81.3626904117636,57.495,5.556));
#52703=CARTESIAN_POINT('',(81.9987283961437,54.32,7.3035));
#52704=CARTESIAN_POINT('Origin',(82.5814567437915,54.32,7.3035));
#52705=CARTESIAN_POINT('',(82.5814567437915,54.32,7.3035));
#52706=CARTESIAN_POINT('',(81.9987283961437,54.32,7.3035));
#52707=CARTESIAN_POINT('',(82.5814567437916,57.495,7.3035));
#52708=CARTESIAN_POINT('',(81.9987283961437,57.495,7.3035));
#52709=CARTESIAN_POINT('',(82.5814567437915,54.32,7.3035));
#52710=CARTESIAN_POINT('Origin',(83.2174947281717,54.32,5.556));
#52711=CARTESIAN_POINT('',(83.2174947281717,54.32,5.556));
#52712=CARTESIAN_POINT('',(82.5814567437915,54.32,7.3035));
#52713=CARTESIAN_POINT('',(83.2174947281717,57.495,5.556));
#52714=CARTESIAN_POINT('',(82.5814567437915,57.495,7.3035));
#52715=CARTESIAN_POINT('',(83.2174947281717,54.32,5.556));
#52716=CARTESIAN_POINT('Origin',(83.8563295805504,54.32,5.556));
#52717=CARTESIAN_POINT('',(83.8563295805504,54.32,5.556));
#52718=CARTESIAN_POINT('',(83.2174947281717,54.32,5.556));
#52719=CARTESIAN_POINT('',(83.8563295805505,57.495,5.556));
#52720=CARTESIAN_POINT('',(83.2174947281717,57.495,5.556));
#52721=CARTESIAN_POINT('',(83.8563295805504,54.32,5.556));
#52722=CARTESIAN_POINT('Origin',(84.4923675649306,54.32,7.3035));
#52723=CARTESIAN_POINT('',(84.4923675649306,54.32,7.3035));
#52724=CARTESIAN_POINT('',(83.8563295805504,54.32,5.556));
#52725=CARTESIAN_POINT('',(84.4923675649306,57.495,7.3035));
#52726=CARTESIAN_POINT('',(83.8563295805504,57.495,5.556));
#52727=CARTESIAN_POINT('',(84.4923675649306,54.32,7.3035));
#52728=CARTESIAN_POINT('Origin',(85.0750959125784,54.32,7.3035));
#52729=CARTESIAN_POINT('',(85.0750959125784,54.32,7.3035));
#52730=CARTESIAN_POINT('',(84.4923675649306,54.32,7.3035));
#52731=CARTESIAN_POINT('',(85.0750959125784,57.495,7.3035));
#52732=CARTESIAN_POINT('',(84.4923675649306,57.495,7.3035));
#52733=CARTESIAN_POINT('',(85.0750959125784,54.32,7.3035));
#52734=CARTESIAN_POINT('Origin',(85.7111338969586,54.32,5.556));
#52735=CARTESIAN_POINT('',(85.7111338969586,54.32,5.556));
#52736=CARTESIAN_POINT('',(85.0750959125784,54.32,7.3035));
#52737=CARTESIAN_POINT('',(85.7111338969587,57.495,5.556));
#52738=CARTESIAN_POINT('',(85.0750959125784,57.495,7.3035));
#52739=CARTESIAN_POINT('',(85.7111338969586,54.32,5.556));
#52740=CARTESIAN_POINT('Origin',(86.3499687493374,54.32,5.556));
#52741=CARTESIAN_POINT('',(86.3499687493374,54.32,5.556));
#52742=CARTESIAN_POINT('',(85.7111338969586,54.32,5.556));
#52743=CARTESIAN_POINT('',(86.3499687493374,57.495,5.556));
#52744=CARTESIAN_POINT('',(85.7111338969586,57.495,5.556));
#52745=CARTESIAN_POINT('',(86.3499687493374,54.32,5.556));
#52746=CARTESIAN_POINT('Origin',(86.9860067337175,54.32,7.3035));
#52747=CARTESIAN_POINT('',(86.3499687493374,54.32,5.556));
#52748=CARTESIAN_POINT('',(86.3499687493374,57.495,5.556));
#52749=CARTESIAN_POINT('Origin',(0.,57.495,11.19225));
#52750=CARTESIAN_POINT('Origin',(0.,54.32,11.19225));
#83195=UNCERTAINTY_MEASURE_WITH_UNIT(LENGTH_MEASURE(0.01),#83220,
'DISTANCE_ACCURACY_VALUE',
'Maximum model space distance between geometric entities at asserted c
onnectivities');
#83203=UNCERTAINTY_MEASURE_WITH_UNIT(LENGTH_MEASURE(0.01),#83220,
'DISTANCE_ACCURACY_VALUE',
'Maximum model space distance between geometric entities at asserted c
onnectivities');
#83211=(
GEOMETRIC_REPRESENTATION_CONTEXT(3)
GLOBAL_UNCERTAINTY_ASSIGNED_CONTEXT((#83195))
GLOBAL_UNIT_ASSIGNED_CONTEXT((#83220,#83222,#83223))
REPRESENTATION_CONTEXT('','3D')
);
#83219=(
GEOMETRIC_REPRESENTATION_CONTEXT(3)
GLOBAL_UNCERTAINTY_ASSIGNED_CONTEXT((#83203))
GLOBAL_UNIT_ASSIGNED_CONTEXT((#83220,#83222,#83223))
REPRESENTATION_CONTEXT('','3D')
);
#83220=(
LENGTH_UNIT()
NAMED_UNIT(*)
SI_UNIT(.MILLI.,.METRE.)
);
#83222=(
NAMED_UNIT(*)
PLANE_ANGLE_UNIT()
SI_UNIT($,.RADIAN.)
);
#83223=(
NAMED_UNIT(*)
SI_UNIT($,.STERADIAN.)
SOLID_ANGLE_UNIT()
);
#83231=SHAPE_DEFINITION_REPRESENTATION(#83246,#83306);
#83246=PRODUCT_DEFINITION_SHAPE('',$,#83322);
#83306=SHAPE_REPRESENTATION('',(#28000),#83211);
#83314=PRODUCT_DEFINITION_CONTEXT('part definition',#83361,'design');
#83322=PRODUCT_DEFINITION('32P Beam Gear Rack Acetal (cut to 70T)',
'32P Beam Gear Rack Acetal (cut to 70T)',#83337,#83314);
#83337=PRODUCT_DEFINITION_FORMATION('',$,#83370);
#83361=APPLICATION_CONTEXT(
'Core Data for Automotive Mechanical Design Process');
#83362=PRODUCT_CONTEXT('part definition',#83361,'mechanical');
#83370=PRODUCT('32P Beam Gear Rack Acetal (cut to 70T)',
'32P Beam Gear Rack Acetal (cut to 70T)',$,(#83362));
#83385=PRESENTATION_STYLE_ASSIGNMENT((#83400));
#83400=SURFACE_STYLE_USAGE(.BOTH.,#83415);
#83415=SURFACE_SIDE_STYLE('',(#83430));
#83430=SURFACE_STYLE_FILL_AREA(#83445);
#83445=FILL_AREA_STYLE('Opaque(206,210,216)',(#83460));
#83460=FILL_AREA_STYLE_COLOUR('Opaque(206,210,216)',#83475);
#83475=COLOUR_RGB('Opaque(206,210,216)', 0.66274510, 0.83137255, 0.94901961);
ENDSEC;
END-ISO-10303-21;
